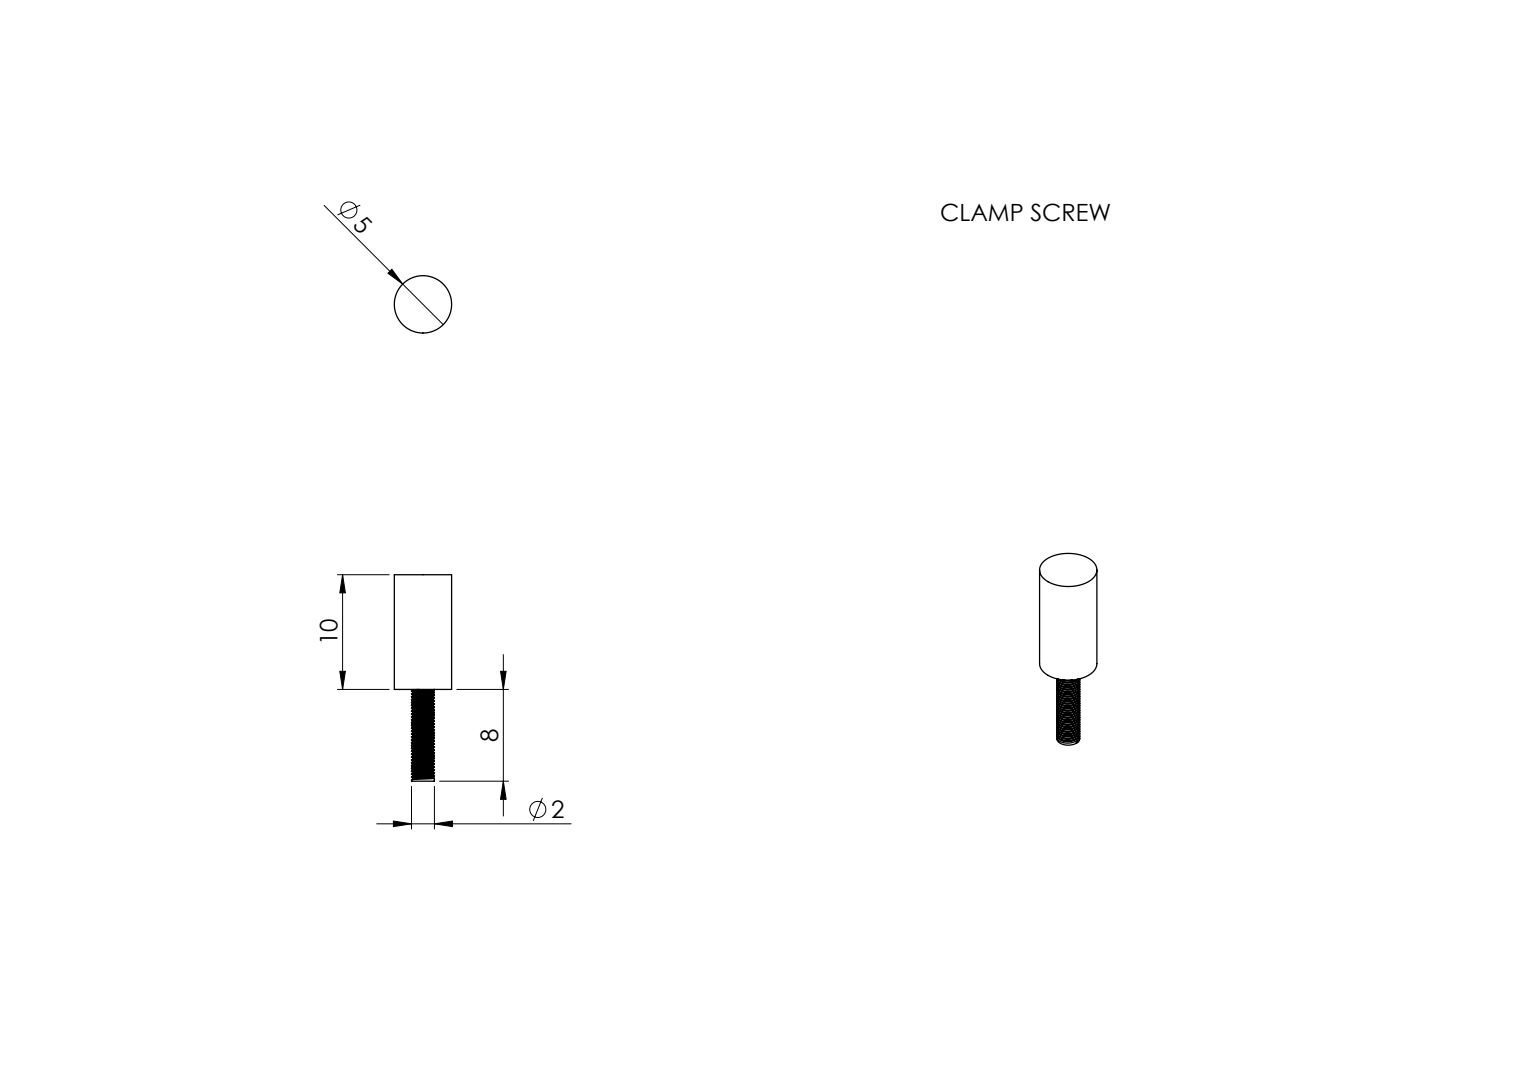
ISO-10303-21;
HEADER;
FILE_DESCRIPTION (('STEP AP214'),
    '1' );
FILE_NAME ('clamp screw.step',
    '2026-10-27T04:40:18',
    ( '' ),
    ( '' ),
    'SwSTEP 2.0',
    'SolidWorks 2026',
    '' );
FILE_SCHEMA (( 'AUTOMOTIVE_DESIGN' ));
ENDSEC;

DATA;
#2=CARTESIAN_POINT ( 'NONE',  ( -60.99999999999998579, 10.72916666666666607, 2.077350269189628840 ) ) ;
#3=CARTESIAN_POINT ( 'NONE',  ( -62.86468353124999453, 12.51562499965860198, 1.500000000000002220 ) ) ;
#4=CARTESIAN_POINT ( 'NONE',  ( -62.43234176562498305, 9.411458332991935904, 0.7511620957034662593 ) ) ;
#5=DIRECTION ( 'NONE',  ( 0.000000000000000000, 0.000000000000000000, -1.000000000000000000 ) ) ;
#7=CARTESIAN_POINT ( 'NONE',  ( -61.99999999999998579, 16.00000000000000000, 1.500000000000002220 ) ) ;
#8=CARTESIAN_POINT ( 'NONE',  ( -62.43234176562498305, 9.223958332991935904, 0.7511620957034662593 ) ) ;
#14=CARTESIAN_POINT ( 'NONE',  ( -62.86468353124998032, 15.68229166632526628, 1.000774730468978024 ) ) ;
#15=CARTESIAN_POINT ( 'NONE',  ( -61.99999999999998579, 11.14062499965860020, 0.5015494609379544944 ) ) ;
#16=CARTESIAN_POINT ( 'NONE',  ( -62.86468353124999453, 16.03645833299193768, 1.999225269531025750 ) ) ;
#17=CARTESIAN_POINT ( 'NONE',  ( -61.49999999999998579, 9.677083332650534331, 2.366025403784441927 ) ) ;
#18=ORIENTED_EDGE ( 'NONE', *, *, #1732, .F. ) ;
#19=CARTESIAN_POINT ( 'NONE',  ( -62.49999999999998579, 14.58333333333333393, 0.6339745962155627357 ) ) ;
#21=CARTESIAN_POINT ( 'NONE',  ( -61.56765823437498852, 8.598958332991934128, 2.248837904296538515 ) ) ;
#23=CARTESIAN_POINT ( 'NONE',  ( -61.49999999999998579, 13.67708333265053433, 2.366025403784441927 ) ) ;
#26=( BOUNDED_CURVE ( )  B_SPLINE_CURVE ( 2, ( #4662, #10727, #5554, #5432, #3111, #6399, #1393, #5495, #3837 ),
 .UNSPECIFIED., .F., .T. ) 
 B_SPLINE_CURVE_WITH_KNOTS ( ( 3, 2, 2, 2, 3 ),
 ( 0.3984375000000000000, 0.4010416666666666852, 0.4062500000000000000, 0.4114583333333333148, 0.4140625000000000000 ),
 .UNSPECIFIED. ) 
 CURVE ( )  GEOMETRIC_REPRESENTATION_ITEM ( )  RATIONAL_B_SPLINE_CURVE ( ( 0.9330127018922194093, 0.9330127018922194093, 1.000000000000000000, 0.8660254037844387076, 1.000000000000000000, 0.8660254037844387076, 1.000000000000000000, 0.9330127018922194093, 0.9330127018922194093 ) ) 
 REPRESENTATION_ITEM ( '' )  );
#27=CARTESIAN_POINT ( 'NONE',  ( -62.86468353124998032, 11.68229166632526983, 1.000774730468978024 ) ) ;
#31=CARTESIAN_POINT ( 'NONE',  ( -62.86468353124998742, 13.28645833299193413, 1.999225269531025972 ) ) ;
#32=CARTESIAN_POINT ( 'NONE',  ( -61.99999999999998579, 11.65624999931720218, 2.500000000000002665 ) ) ;
#35=VERTEX_POINT ( 'NONE', #9289 ) ;
#42=CARTESIAN_POINT ( 'NONE',  ( -61.99999999999998579, 8.703124999658601979, 0.5015494609379544944 ) ) ;
#43=CARTESIAN_POINT ( 'NONE',  ( -61.99999999999998579, 15.93749999999999645, 2.500000000000002665 ) ) ;
#44=AXIS2_PLACEMENT_3D ( 'NONE', #893, #1059, #6847 ) ;
#45=CARTESIAN_POINT ( 'NONE',  ( -61.13531646874998415, 12.66145833299193413, 1.000774730468978468 ) ) ;
#51=CARTESIAN_POINT ( 'NONE',  ( -62.99999999999998579, 11.57291666598387003, 0.9226497308103756012 ) ) ;
#52=CARTESIAN_POINT ( 'NONE',  ( -62.43234176562498305, 15.66145833299193590, 0.7511620957034662593 ) ) ;
#54=CARTESIAN_POINT ( 'NONE',  ( -61.49999999999998579, 12.51041666598386826, 0.6339745962155628467 ) ) ;
#55=CARTESIAN_POINT ( 'NONE',  ( -62.99999999999998579, 8.854166666666666075, 0.9226497308103756012 ) ) ;
#56=CARTESIAN_POINT ( 'NONE',  ( -61.13531646874997705, 12.41145833299193413, 1.000774730468978468 ) ) ;
#58=CARTESIAN_POINT ( 'NONE',  ( -61.13531646874998415, 9.057291666325266277, 1.999225269531026417 ) ) ;
#59=CARTESIAN_POINT ( 'NONE',  ( -61.49999999999998579, 9.208333333333333925, 2.366025403784441927 ) ) ;
#61=CARTESIAN_POINT ( 'NONE',  ( -61.13531646874998415, 9.661458332991932352, 1.000774730468978468 ) ) ;
#62=CARTESIAN_POINT ( 'NONE',  ( -62.99999999999998579, 14.07291666598387003, 0.9226497308103756012 ) ) ;
#64=VECTOR ( 'NONE', #9723, 1000.000000000000000 ) ;
#65=CARTESIAN_POINT ( 'NONE',  ( -61.99999999999998579, 12.81250000000000000, 0.5000000000000013323 ) ) ;
#66=CARTESIAN_POINT ( 'NONE',  ( -61.73205080756886076, 11.16741454900183328, 2.500000000000003109 ) ) ;
#67=CARTESIAN_POINT ( 'NONE',  ( -61.99999999999999289, 15.14062499965860198, 0.5015494609379544944 ) ) ;
#68=CARTESIAN_POINT ( 'NONE',  ( -62.43234176562499016, 10.74479166632526805, 2.248837904296538071 ) ) ;
#69=CARTESIAN_POINT ( 'NONE',  ( -61.99999999999999289, 15.82812499965860198, 2.498450539062049724 ) ) ;
#71=EDGE_LOOP ( 'NONE', ( #7087, #10551, #5486, #977 ) ) ;
#72=CARTESIAN_POINT ( 'NONE',  ( -62.49999999999998579, 15.08333333333333393, 0.6339745962155627357 ) ) ;
#73=CARTESIAN_POINT ( 'NONE',  ( -62.86468353124999453, 8.286458332991934128, 1.999225269531025750 ) ) ;
#74=CARTESIAN_POINT ( 'NONE',  ( -62.49999999999998579, 13.30208333265053433, 0.6339745962155627357 ) ) ;
#75=CARTESIAN_POINT ( 'NONE',  ( -62.99999999999998579, 13.12500000000000178, 1.500000000000001998 ) ) ;
#76=CARTESIAN_POINT ( 'NONE',  ( -61.99999999999998579, 9.812500000000000000, 0.5000000000000013323 ) ) ;
#77=CARTESIAN_POINT ( 'NONE',  ( -61.56765823437498852, 11.03645833299193590, 2.248837904296538515 ) ) ;
#78=( NAMED_UNIT ( * ) SI_UNIT ( $, .STERADIAN. ) SOLID_ANGLE_UNIT ( ) );
#79=CARTESIAN_POINT ( 'NONE',  ( -61.99999999999997868, 8.312499999999998224, 0.5000000000000013323 ) ) ;
#80=ORIENTED_EDGE ( 'NONE', *, *, #3705, .F. ) ;
#81=CARTESIAN_POINT ( 'NONE',  ( -61.99999999999998579, 12.15624999931720041, 2.500000000000002665 ) ) ;
#82=CARTESIAN_POINT ( 'NONE',  ( -61.13531646874998415, 13.16145833299193413, 1.000774730468978468 ) ) ;
#84=DIRECTION ( 'NONE',  ( -0.000000000000000000, -1.000000000000000000, -0.000000000000000000 ) ) ;
#85=CARTESIAN_POINT ( 'NONE',  ( -60.99999999999998579, 8.697916665983868256, 2.077350269189628840 ) ) ;
#87=( BOUNDED_CURVE ( )  B_SPLINE_CURVE ( 2, ( #8357, #10903, #5902, #8456, #10798, #841, #3187, #174, #6119 ),
 .UNSPECIFIED., .F., .T. ) 
 B_SPLINE_CURVE_WITH_KNOTS ( ( 3, 2, 2, 2, 3 ),
 ( 0.5703125000000000000, 0.5729166666666666297, 0.5781250000000000000, 0.5833333333333333703, 0.5859375000000000000 ),
 .UNSPECIFIED. ) 
 CURVE ( )  GEOMETRIC_REPRESENTATION_ITEM ( )  RATIONAL_B_SPLINE_CURVE ( ( 0.9330127018922194093, 0.9330127018922194093, 1.000000000000000000, 0.8660254037844387076, 1.000000000000000000, 0.8660254037844387076, 1.000000000000000000, 0.9330127018922194093, 0.9330127018922194093 ) ) 
 REPRESENTATION_ITEM ( '' )  );
#92=CARTESIAN_POINT ( 'NONE',  ( -62.43234176562498305, 11.91145833299193413, 0.7511620957034662593 ) ) ;
#94=CARTESIAN_POINT ( 'NONE',  ( -62.43234176562499016, 9.057291666325268054, 2.248837904296538071 ) ) ;
#95=LINE ( 'NONE', #7549, #8153 ) ;
#96=CARTESIAN_POINT ( 'NONE',  ( -61.56765823437498852, 12.59895833299193413, 2.248837904296538515 ) ) ;
#98=CARTESIAN_POINT ( 'NONE',  ( -61.99999999999998579, 8.281249999317202182, 0.5000000000000013323 ) ) ;
#100=CARTESIAN_POINT ( 'NONE',  ( -61.99999999999998579, 16.00000000000000000, 2.500000000000000444 ) ) ;
#101=ORIENTED_EDGE ( 'NONE', *, *, #9521, .F. ) ;
#102=CARTESIAN_POINT ( 'NONE',  ( -61.73205080756886076, 14.27008544963257108, 0.5000000000000014433 ) ) ;
#103=CARTESIAN_POINT ( 'NONE',  ( -61.13531646874998415, 15.30729166632526983, 1.999225269531026417 ) ) ;
#104=FACE_OUTER_BOUND ( 'NONE', #8107, .T. ) ;
#106=CARTESIAN_POINT ( 'NONE',  ( -62.49999999999998579, 12.30208333265053611, 0.6339745962155627357 ) ) ;
#108=CARTESIAN_POINT ( 'NONE',  ( -61.56765823437498852, 14.34895833299193413, 2.248837904296538515 ) ) ;
#109=CARTESIAN_POINT ( 'NONE',  ( -62.43234176562499016, 8.494791666325268054, 2.248837904296538071 ) ) ;
#110=CARTESIAN_POINT ( 'NONE',  ( -61.99999999999998579, 9.187500000000000000, 2.500000000000002665 ) ) ;
#112=CARTESIAN_POINT ( 'NONE',  ( -61.56765823437498142, 8.682291666325268054, 0.7511620957034663704 ) ) ;
#113=ADVANCED_FACE ( 'NONE', ( #788 ), #9184, .T. ) ;
#114=CARTESIAN_POINT ( 'NONE',  ( -62.49999999999998579, 14.05208333265053611, 0.6339745962155627357 ) ) ;
#119=CARTESIAN_POINT ( 'NONE',  ( -61.13531646874998415, 15.07812499965860020, 1.500000000000002220 ) ) ;
#120=CARTESIAN_POINT ( 'NONE',  ( -62.86468353124998032, 10.93229166632526805, 1.000774730468978246 ) ) ;
#121=CARTESIAN_POINT ( 'NONE',  ( -61.56765823437498852, 9.536458332991934128, 2.248837904296538515 ) ) ;
#122=ORIENTED_EDGE ( 'NONE', *, *, #10904, .T. ) ;
#123=CARTESIAN_POINT ( 'NONE',  ( -62.99999999999998579, 15.12500000000000000, 1.500000000000001998 ) ) ;
#124=CARTESIAN_POINT ( 'NONE',  ( -61.13531646874998415, 9.640624999658601979, 1.500000000000002220 ) ) ;
#127=CARTESIAN_POINT ( 'NONE',  ( -61.49999999999998579, 13.76041666598387003, 0.6339745962155628467 ) ) ;
#129=CARTESIAN_POINT ( 'NONE',  ( -61.99999999999998579, 14.90624999931720218, 2.500000000000002665 ) ) ;
#131=CARTESIAN_POINT ( 'NONE',  ( -62.86468353124999453, 11.97395833299193413, 1.999225269531025750 ) ) ;
#132=( NAMED_UNIT ( * ) PLANE_ANGLE_UNIT ( ) SI_UNIT ( $, .RADIAN. ) );
#133=LINE ( 'NONE', #9524, #10148 ) ;
#136=CARTESIAN_POINT ( 'NONE',  ( -61.13531646874998415, 12.91145833299193590, 1.000774730468978468 ) ) ;
#138=CARTESIAN_POINT ( 'NONE',  ( -60.99999999999998579, 10.22916666666666785, 2.077350269189628840 ) ) ;
#139=VECTOR ( 'NONE', #2970, 1000.000000000000000 ) ;
#140=CARTESIAN_POINT ( 'NONE',  ( -62.49999999999998579, 9.302083332650536107, 0.6339745962155627357 ) ) ;
#143=CARTESIAN_POINT ( 'NONE',  ( -61.73205080756886076, 14.05133545031537068, 0.5000000000000014433 ) ) ;
#145=CARTESIAN_POINT ( 'NONE',  ( -62.26794919243111082, 15.29241454900183328, 0.5000000000000013323 ) ) ;
#147=CARTESIAN_POINT ( 'NONE',  ( -61.13531646874998415, 11.05729166632526805, 1.999225269531026417 ) ) ;
#151=CARTESIAN_POINT ( 'NONE',  ( -61.13531646874998415, 8.411458332991934128, 1.000774730468978468 ) ) ;
#155=CARTESIAN_POINT ( 'NONE',  ( -61.56765823437498852, 14.09895833299193413, 2.248837904296538515 ) ) ;
#156=CARTESIAN_POINT ( 'NONE',  ( -62.49999999999998579, 9.302083332650536107, 0.6339745962155627357 ) ) ;
#157=ORIENTED_EDGE ( 'NONE', *, *, #473, .F. ) ;
#160=CARTESIAN_POINT ( 'NONE',  ( -62.49999999999998579, 10.83333333333333393, 0.6339745962155627357 ) ) ;
#161=CARTESIAN_POINT ( 'NONE',  ( -62.99999999999998579, 8.104166666666667851, 0.9226497308103756012 ) ) ;
#163=CARTESIAN_POINT ( 'NONE',  ( -61.99999999999997868, 8.781249999317202182, 0.5000000000000013323 ) ) ;
#164=DIRECTION ( 'NONE',  ( -0.000000000000000000, -1.000000000000000000, -0.000000000000000000 ) ) ;
#165=CARTESIAN_POINT ( 'NONE',  ( -61.73205080756888208, 10.69866454968463110, 2.500000000000006661 ) ) ;
#166=CARTESIAN_POINT ( 'NONE',  ( -61.13531646874997705, 13.41145833299193413, 1.000774730468978468 ) ) ;
#167=CARTESIAN_POINT ( 'NONE',  ( -61.56765823437498142, 8.869791666325268054, 0.7511620957034663704 ) ) ;
#168=LINE ( 'NONE', #6113, #341 ) ;
#170=CARTESIAN_POINT ( 'NONE',  ( -62.86468353124998742, 9.786458332991934128, 1.999225269531025972 ) ) ;
#172=ORIENTED_EDGE ( 'NONE', *, *, #7897, .T. ) ;
#174=CARTESIAN_POINT ( 'NONE',  ( -62.26794919243111082, 12.67633545031537068, 2.500000000000003109 ) ) ;
#175=EDGE_CURVE ( 'NONE', #2979, #4700, #8697, .T. ) ;
#177=CARTESIAN_POINT ( 'NONE',  ( -62.43234176562499016, 14.99479166632526805, 2.248837904296538071 ) ) ;
#178=CARTESIAN_POINT ( 'NONE',  ( -62.86468353124998742, 11.47395833299193590, 1.999225269531025972 ) ) ;
#180=ADVANCED_FACE ( 'NONE', ( #9080 ), #7568, .T. ) ;
#181=CARTESIAN_POINT ( 'NONE',  ( -61.13531646874998415, 8.578124999658601979, 1.500000000000002220 ) ) ;
#182=CARTESIAN_POINT ( 'NONE',  ( -61.99999999999998579, 11.40624999931720218, 2.500000000000002665 ) ) ;
#183=ORIENTED_EDGE ( 'NONE', *, *, #3221, .T. ) ;
#184=CARTESIAN_POINT ( 'NONE',  ( -62.99999999999998579, 14.60416666666666785, 0.9226497308103756012 ) ) ;
#185=CARTESIAN_POINT ( 'NONE',  ( -61.56765823437498852, 10.09895833299193413, 2.248837904296538515 ) ) ;
#186=CARTESIAN_POINT ( 'NONE',  ( -62.99999999999998579, 13.59374999931720218, 1.500000000000001998 ) ) ;
#188=ORIENTED_EDGE ( 'NONE', *, *, #5061, .T. ) ;
#189=CYLINDRICAL_SURFACE ( 'NONE', #9638, 0.9999999999999981126 ) ;
#190=CARTESIAN_POINT ( 'NONE',  ( -62.86468353124998032, 10.93229166632526805, 1.000774730468978024 ) ) ;
#191=CARTESIAN_POINT ( 'NONE',  ( -60.99999999999998579, 13.00000000000000178, 1.500000000000002220 ) ) ;
#193=CARTESIAN_POINT ( 'NONE',  ( -62.49999999999998579, 10.58333333333333393, 0.6339745962155627357 ) ) ;
#194=CARTESIAN_POINT ( 'NONE',  ( -61.73205080756886076, 15.91741454900183150, 2.500000000000003109 ) ) ;
#195=CARTESIAN_POINT ( 'NONE',  ( -62.86468353124999453, 14.26562499965860020, 1.500000000000002220 ) ) ;
#196=CARTESIAN_POINT ( 'NONE',  ( -62.49999999999998579, 13.91666666666666785, 2.366025403784441483 ) ) ;
#198=CARTESIAN_POINT ( 'NONE',  ( -62.99999999999998579, 8.614583332650536107, 2.077350269189627952 ) ) ;
#202=CARTESIAN_POINT ( 'NONE',  ( -61.73205080756886076, 10.02008544963257464, 0.5000000000000014433 ) ) ;
#203=CARTESIAN_POINT ( 'NONE',  ( -61.56765823437498142, 11.36979166632526805, 0.7511620957034663704 ) ) ;
#207=CARTESIAN_POINT ( 'NONE',  ( -61.13531646874998415, 10.91145833299193590, 1.000774730468978468 ) ) ;
#209=CARTESIAN_POINT ( 'NONE',  ( -61.13531646874998415, 14.16145833299193413, 1.000774730468978468 ) ) ;
#210=CARTESIAN_POINT ( 'NONE',  ( -62.26794919243111082, 9.292414549001833279, 0.5000000000000013323 ) ) ;
#217=CARTESIAN_POINT ( 'NONE',  ( -61.99999999999998579, 15.03124999931720218, 0.5000000000000013323 ) ) ;
#218=CARTESIAN_POINT ( 'NONE',  ( -61.99999999999998579, 8.437500000000000000, 2.654700538379254571 ) ) ;
#219=CARTESIAN_POINT ( 'NONE',  ( -61.99999999999998579, 13.68749999999999822, 2.500000000000002665 ) ) ;
#221=DIRECTION ( 'NONE',  ( -0.000000000000000000, -1.000000000000000000, -0.000000000000000000 ) ) ;
#223=CARTESIAN_POINT ( 'NONE',  ( -62.86468353124998032, 14.49479166632526983, 1.000774730468978024 ) ) ;
#225=CARTESIAN_POINT ( 'NONE',  ( -61.99999999999998579, 8.515624999658601979, 2.498450539062049724 ) ) ;
#226=CARTESIAN_POINT ( 'NONE',  ( -62.99999999999998579, 11.32291666598387181, 0.9226497308103756012 ) ) ;
#228=CARTESIAN_POINT ( 'NONE',  ( -61.13531646874998415, 10.11979166632526805, 1.999225269531026417 ) ) ;
#229=CARTESIAN_POINT ( 'NONE',  ( -61.99999999999998579, 14.03124999931720218, 0.5000000000000013323 ) ) ;
#232=CARTESIAN_POINT ( 'NONE',  ( -61.99999999999998579, 13.03124999931720218, 0.5000000000000013323 ) ) ;
#235=CARTESIAN_POINT ( 'NONE',  ( -61.13531646874997705, 15.59895833299193590, 1.000774730468978468 ) ) ;
#236=CARTESIAN_POINT ( 'NONE',  ( -61.56765823437498852, 13.03645833299193413, 2.248837904296538515 ) ) ;
#237=CARTESIAN_POINT ( 'NONE',  ( -61.99999999999999289, 8.265624999658601979, 2.498450539062049724 ) ) ;
#239=CARTESIAN_POINT ( 'NONE',  ( -62.26794919243111082, 14.07366454968463110, 0.5000000000000013323 ) ) ;
#240=CARTESIAN_POINT ( 'NONE',  ( -62.43234176562499016, 9.557291666325268054, 2.248837904296538071 ) ) ;
#241=CARTESIAN_POINT ( 'NONE',  ( -61.56765823437498852, 14.78645833299193413, 2.248837904296538515 ) ) ;
#243=CARTESIAN_POINT ( 'NONE',  ( -61.99999999999998579, 14.28124999931720396, 0.3452994616207497591 ) ) ;
#245=ORIENTED_EDGE ( 'NONE', *, *, #9568, .F. ) ;
#246=CARTESIAN_POINT ( 'NONE',  ( -61.73205080756886076, 9.801335450315370679, 0.5000000000000014433 ) ) ;
#248=CARTESIAN_POINT ( 'NONE',  ( -61.13531646874998415, 12.07812499965860198, 1.500000000000002220 ) ) ;
#249=CYLINDRICAL_SURFACE ( 'NONE', #10424, 0.9999999999999981126 ) ;
#252=CARTESIAN_POINT ( 'NONE',  ( -61.49999999999998579, 11.04166666666666607, 0.6339745962155628467 ) ) ;
#253=CARTESIAN_POINT ( 'NONE',  ( -61.99999999999998579, 8.531249999317203958, 0.5000000000000013323 ) ) ;
#254=CARTESIAN_POINT ( 'NONE',  ( -61.99999999999998579, 14.57812499965860198, 2.498450539062049724 ) ) ;
#255=( BOUNDED_CURVE ( )  B_SPLINE_CURVE ( 2, ( #5430, #6282, #8897, #2058, #9721, #9666, #6225, #10606, #9607 ),
 .UNSPECIFIED., .F., .T. ) 
 B_SPLINE_CURVE_WITH_KNOTS ( ( 3, 2, 2, 2, 3 ),
 ( 0.08593750000000000000, 0.08854166666666667129, 0.09375000000000000000, 0.09895833333333332871, 0.1015625000000000833 ),
 .UNSPECIFIED. ) 
 CURVE ( )  GEOMETRIC_REPRESENTATION_ITEM ( )  RATIONAL_B_SPLINE_CURVE ( ( 0.9330127018922194093, 0.9330127018922194093, 1.000000000000000000, 0.8660254037844387076, 1.000000000000000000, 0.8660254037844387076, 1.000000000000000000, 0.9330127018922171889, 0.9330127018922194093 ) ) 
 REPRESENTATION_ITEM ( '' )  );
#257=CARTESIAN_POINT ( 'NONE',  ( -61.99999999999998579, 13.93749999999999822, 2.500000000000002665 ) ) ;
#258=CARTESIAN_POINT ( 'NONE',  ( -62.99999999999998579, 9.364583332650536107, 2.077350269189627952 ) ) ;
#260=CARTESIAN_POINT ( 'NONE',  ( -61.49999999999998579, 13.54166666666666785, 0.6339745962155628467 ) ) ;
#261=CARTESIAN_POINT ( 'NONE',  ( -62.49999999999998579, 15.38541666598387003, 2.366025403784441483 ) ) ;
#262=CARTESIAN_POINT ( 'NONE',  ( -62.43234176562499016, 10.74479166632526805, 2.248837904296538071 ) ) ;
#263=ADVANCED_FACE ( 'NONE', ( #7011 ), #2615, .T. ) ;
#264=ORIENTED_EDGE ( 'NONE', *, *, #1352, .F. ) ;
#265=CARTESIAN_POINT ( 'NONE',  ( -62.43234176562499016, 10.05729166632526805, 2.248837904296538071 ) ) ;
#267=CARTESIAN_POINT ( 'NONE',  ( -61.13531646874998415, 13.86979166632526805, 1.999225269531026417 ) ) ;
#269=ORIENTED_EDGE ( 'NONE', *, *, #9235, .F. ) ;
#273=CARTESIAN_POINT ( 'NONE',  ( -62.49999999999998579, 8.416666666666666075, 2.366025403784441483 ) ) ;
#277=CARTESIAN_POINT ( 'NONE',  ( -61.56765823437498142, 13.93229166632526805, 0.7511620957034663704 ) ) ;
#278=CARTESIAN_POINT ( 'NONE',  ( -62.86468353124998742, 9.723958332991934128, 1.999225269531025972 ) ) ;
#280=CARTESIAN_POINT ( 'NONE',  ( -61.13531646874998415, 9.911458332991935904, 1.000774730468978468 ) ) ;
#281=CARTESIAN_POINT ( 'NONE',  ( -62.49999999999998579, 12.08333333333333393, 0.6339745962155627357 ) ) ;
#283=EDGE_CURVE ( 'NONE', #10857, #3037, #6901, .T. ) ;
#284=VECTOR ( 'NONE', #526, 1000.000000000000000 ) ;
#286=CARTESIAN_POINT ( 'NONE',  ( -60.99999999999998579, 12.98958333265053611, 0.9226497308103762673 ) ) ;
#287=ADVANCED_FACE ( 'NONE', ( #6844 ), #3445, .T. ) ;
#288=CARTESIAN_POINT ( 'NONE',  ( -62.26794919243111082, 10.04241454900183328, 0.5000000000000013323 ) ) ;
#289=CARTESIAN_POINT ( 'NONE',  ( -61.99999999999998579, 12.14062499965860198, 0.5015494609379544944 ) ) ;
#290=CARTESIAN_POINT ( 'NONE',  ( -61.99999999999999289, 8.890624999658601979, 0.5015494609379544944 ) ) ;
#293=CARTESIAN_POINT ( 'NONE',  ( -60.99999999999998579, 15.97916666666666607, 2.077350269189628840 ) ) ;
#294=CARTESIAN_POINT ( 'NONE',  ( -61.13531646874997705, 10.41145833299193413, 1.000774730468978468 ) ) ;
#296=CARTESIAN_POINT ( 'NONE',  ( -61.56765823437498142, 15.61979166632526628, 0.7511620957034663704 ) ) ;
#297=ADVANCED_FACE ( 'NONE', ( #7844 ), #6003, .T. ) ;
#298=CARTESIAN_POINT ( 'NONE',  ( -60.99999999999998579, 14.48958333265053788, 0.9226497308103762673 ) ) ;
#301=CYLINDRICAL_SURFACE ( 'NONE', #3236, 0.9999999999999981126 ) ;
#303=CARTESIAN_POINT ( 'NONE',  ( -61.56765823437498852, 12.78645833299193413, 2.248837904296538515 ) ) ;
#304=CARTESIAN_POINT ( 'NONE',  ( -61.56765823437498142, 8.619791666325268054, 0.7511620957034663704 ) ) ;
#305=CARTESIAN_POINT ( 'NONE',  ( -61.49999999999998579, 15.54166666666666607, 0.6339745962155628467 ) ) ;
#307=CARTESIAN_POINT ( 'NONE',  ( -61.99999999999998579, 12.18750000000000000, 2.654700538379254571 ) ) ;
#308=LINE ( 'NONE', #2873, #10328 ) ;
#309=CARTESIAN_POINT ( 'NONE',  ( -62.86468353124998032, 13.99479166632526983, 1.000774730468978246 ) ) ;
#311=CARTESIAN_POINT ( 'NONE',  ( -61.49999999999998579, 10.26041666598387003, 0.6339745962155628467 ) ) ;
#312=VERTEX_POINT ( 'NONE', #9336 ) ;
#314=CARTESIAN_POINT ( 'NONE',  ( -60.99999999999998579, 9.989583332650536107, 0.9226497308103762673 ) ) ;
#315=CARTESIAN_POINT ( 'NONE',  ( -61.99999999999998579, 12.89062499965860376, 0.5015494609379544944 ) ) ;
#316=ADVANCED_FACE ( 'NONE', ( #9447 ), #3389, .T. ) ;
#317=CARTESIAN_POINT ( 'NONE',  ( -61.49999999999998579, 15.95833333333333215, 2.366025403784441927 ) ) ;
#318=( BOUNDED_CURVE ( )  B_SPLINE_CURVE ( 2, ( #338, #1054, #8015, #9617, #7841, #6343, #2731, #6291, #1116 ),
 .UNSPECIFIED., .F., .T. ) 
 B_SPLINE_CURVE_WITH_KNOTS ( ( 3, 2, 2, 2, 3 ),
 ( 0.1953124999999999722, 0.1979166666666666574, 0.2031250000000000000, 0.2083333333333333426, 0.2109375000000000000 ),
 .UNSPECIFIED. ) 
 CURVE ( )  GEOMETRIC_REPRESENTATION_ITEM ( )  RATIONAL_B_SPLINE_CURVE ( ( 0.9330127018922194093, 0.9330127018922186322, 1.000000000000000000, 0.8660254037844387076, 1.000000000000000000, 0.8660254037844387076, 1.000000000000000000, 0.9330127018922194093, 0.9330127018922194093 ) ) 
 REPRESENTATION_ITEM ( '' )  );
#319=EDGE_LOOP ( 'NONE', ( #4285, #2336, #2477, #10429 ) ) ;
#320=EDGE_CURVE ( 'NONE', #4602, #5526, #6439, .T. ) ;
#321=CARTESIAN_POINT ( 'NONE',  ( -61.99999999999998579, 10.20312499965860198, 0.5015494609379544944 ) ) ;
#323=CARTESIAN_POINT ( 'NONE',  ( -61.56765823437498852, 14.34895833299193413, 2.248837904296538515 ) ) ;
#329=ORIENTED_EDGE ( 'NONE', *, *, #3272, .T. ) ;
#331=CARTESIAN_POINT ( 'NONE',  ( -60.99999999999998579, 8.000000000000000000, 1.500000000000002220 ) ) ;
#335=CARTESIAN_POINT ( 'NONE',  ( -62.86468353124999453, 14.26562499965860020, 1.500000000000002220 ) ) ;
#336=CARTESIAN_POINT ( 'NONE',  ( -61.13531646874998415, 10.32812499965860198, 1.500000000000002220 ) ) ;
#337=CARTESIAN_POINT ( 'NONE',  ( -61.99999999999998579, 13.28124999931720041, 0.5000000000000013323 ) ) ;
#338=CARTESIAN_POINT ( 'NONE',  ( -61.99999999999998579, 9.562500000000000000, 0.5000000000000013323 ) ) ;
#340=CARTESIAN_POINT ( 'NONE',  ( -62.86468353124998742, 10.78645833299193413, 1.999225269531025972 ) ) ;
#341=VECTOR ( 'NONE', #8505, 1000.000000000000000 ) ;
#347=ORIENTED_EDGE ( 'NONE', *, *, #4046, .F. ) ;
#348=CARTESIAN_POINT ( 'NONE',  ( -61.13531646874998415, 8.140624999658601979, 1.500000000000002220 ) ) ;
#349=CARTESIAN_POINT ( 'NONE',  ( -61.13531646874998415, 12.55729166632526805, 1.999225269531026417 ) ) ;
#350=CARTESIAN_POINT ( 'NONE',  ( -61.56765823437498852, 8.786458332991934128, 2.248837904296538515 ) ) ;
#354=DIRECTION ( 'NONE',  ( -0.000000000000000000, -1.000000000000000000, -0.000000000000000000 ) ) ;
#355=CARTESIAN_POINT ( 'NONE',  ( -61.99999999999999289, 10.32812499965860198, 2.498450539062049724 ) ) ;
#357=CARTESIAN_POINT ( 'NONE',  ( -62.43234176562499016, 14.74479166632526805, 2.248837904296538071 ) ) ;
#358=VECTOR ( 'NONE', #7829, 1000.000000000000000 ) ;
#359=CARTESIAN_POINT ( 'NONE',  ( -60.99999999999998579, 13.94791666598387003, 2.077350269189628840 ) ) ;
#360=CYLINDRICAL_SURFACE ( 'NONE', #3974, 0.9999999999999981126 ) ;
#363=CARTESIAN_POINT ( 'NONE',  ( -61.99999999999998579, 16.00000000000000000, 1.500000000000002220 ) ) ;
#366=CARTESIAN_POINT ( 'NONE',  ( -61.13531646874998415, 12.57812499965860198, 1.500000000000002220 ) ) ;
#368=CARTESIAN_POINT ( 'NONE',  ( -62.43234176562499016, 8.994791666325268054, 2.248837904296538071 ) ) ;
#369=CARTESIAN_POINT ( 'NONE',  ( -62.99999999999998579, 10.59374999931720396, 1.500000000000001998 ) ) ;
#370=EDGE_LOOP ( 'NONE', ( #10927, #3084, #707, #1709 ) ) ;
#371=CARTESIAN_POINT ( 'NONE',  ( -62.99999999999998579, 12.87500000000000178, 1.500000000000001998 ) ) ;
#373=CARTESIAN_POINT ( 'NONE',  ( -61.13531646874998415, 14.64062499965860020, 1.500000000000002220 ) ) ;
#374=CARTESIAN_POINT ( 'NONE',  ( -62.26794919243111082, 13.92633545031537068, 2.500000000000003109 ) ) ;
#375=CARTESIAN_POINT ( 'NONE',  ( -61.49999999999998579, 11.26041666598387003, 0.6339745962155628467 ) ) ;
#376=ORIENTED_EDGE ( 'NONE', *, *, #2316, .F. ) ;
#379=CARTESIAN_POINT ( 'NONE',  ( -61.13531646874998415, 12.30729166632526628, 1.999225269531026417 ) ) ;
#381=VERTEX_POINT ( 'NONE', #7734 ) ;
#382=CARTESIAN_POINT ( 'NONE',  ( -61.13531646874998415, 10.14062499965860198, 1.500000000000002220 ) ) ;
#383=CYLINDRICAL_SURFACE ( 'NONE', #5279, 0.9999999999999981126 ) ;
#384=CARTESIAN_POINT ( 'NONE',  ( -62.86468353124999453, 14.76562499965860020, 1.500000000000002220 ) ) ;
#385=DIRECTION ( 'NONE',  ( -0.000000000000000000, -1.000000000000000000, -0.000000000000000000 ) ) ;
#388=EDGE_CURVE ( 'NONE', #8021, #5388, #10231, .T. ) ;
#389=( BOUNDED_CURVE ( )  B_SPLINE_CURVE ( 2, ( #8655, #9486, #5983, #9430, #1883, #5039, #9376, #1038, #1666 ),
 .UNSPECIFIED., .F., .F. ) 
 B_SPLINE_CURVE_WITH_KNOTS ( ( 3, 2, 2, 2, 3 ),
 ( 0.6484375000000000000, 0.6510416666666666297, 0.6562500000000000000, 0.6614583333333333703, 0.6640625000000000000 ),
 .UNSPECIFIED. ) 
 CURVE ( )  GEOMETRIC_REPRESENTATION_ITEM ( )  RATIONAL_B_SPLINE_CURVE ( ( 0.9330127018922194093, 0.9330127018922194093, 1.000000000000000000, 0.8660254037844387076, 1.000000000000000000, 0.8660254037844387076, 1.000000000000000000, 0.9330127018922194093, 0.9330127018922194093 ) ) 
 REPRESENTATION_ITEM ( '' )  );
#390=AXIS2_PLACEMENT_3D ( 'NONE', #8453, #10271, #7624 ) ;
#393=CARTESIAN_POINT ( 'NONE',  ( -60.99999999999998579, 8.479166666666666075, 2.077350269189628840 ) ) ;
#394=CARTESIAN_POINT ( 'NONE',  ( -62.26794919243111082, 9.645085449632574637, 2.500000000000006217 ) ) ;
#395=CARTESIAN_POINT ( 'NONE',  ( -61.99999999999998579, 14.28124999931720218, 0.5000000000000013323 ) ) ;
#397=CARTESIAN_POINT ( 'NONE',  ( -62.86468353124999453, 14.78645833299193058, 1.999225269531025750 ) ) ;
#398=CARTESIAN_POINT ( 'NONE',  ( -62.43234176562498305, 10.16145833299193413, 0.7511620957034662593 ) ) ;
#400=CARTESIAN_POINT ( 'NONE',  ( -62.99999999999998579, 11.36458333265053611, 2.077350269189627952 ) ) ;
#403=CARTESIAN_POINT ( 'NONE',  ( -61.13531646874998415, 11.14062499965860020, 1.500000000000002220 ) ) ;
#411=CARTESIAN_POINT ( 'NONE',  ( -61.73205080756886787, 10.16741454900183150, 2.500000000000004885 ) ) ;
#413=CARTESIAN_POINT ( 'NONE',  ( -61.13531646874998415, 12.84895833299193413, 1.000774730468978468 ) ) ;
#414=VECTOR ( 'NONE', #2699, 1000.000000000000000 ) ;
#415=CARTESIAN_POINT ( 'NONE',  ( -61.56765823437498142, 10.61979166632526805, 0.7511620957034663704 ) ) ;
#416=CARTESIAN_POINT ( 'NONE',  ( -61.99999999999998579, 16.00000000000000000, 0.5000000000000041078 ) ) ;
#418=CARTESIAN_POINT ( 'NONE',  ( -60.99999999999998579, 8.468749999317202182, 1.500000000000002220 ) ) ;
#419=CARTESIAN_POINT ( 'NONE',  ( -61.13531646874998415, 11.14062499965860020, 1.500000000000002220 ) ) ;
#421=CARTESIAN_POINT ( 'NONE',  ( -61.99999999999998579, 14.76562499965859843, 2.498450539062049724 ) ) ;
#422=CARTESIAN_POINT ( 'NONE',  ( -60.99999999999998579, 15.19791666598387181, 2.077350269189628840 ) ) ;
#424=VERTEX_POINT ( 'NONE', #4552 ) ;
#428=CARTESIAN_POINT ( 'NONE',  ( -61.56765823437498852, 13.28645833299193413, 2.248837904296538515 ) ) ;
#429=DIRECTION ( 'NONE',  ( -0.000000000000000000, -1.000000000000000000, -0.000000000000000000 ) ) ;
#432=CARTESIAN_POINT ( 'NONE',  ( -60.99999999999998579, 12.50000000000000000, 1.500000000000002220 ) ) ;
#434=CARTESIAN_POINT ( 'NONE',  ( -60.99999999999998579, 15.94791666598386826, 2.077350269189628840 ) ) ;
#436=CARTESIAN_POINT ( 'NONE',  ( -62.99999999999998579, 14.36458333265053611, 2.077350269189627952 ) ) ;
#437=CARTESIAN_POINT ( 'NONE',  ( -62.99999999999998579, 10.86458333265053611, 2.077350269189627952 ) ) ;
#439=CARTESIAN_POINT ( 'NONE',  ( -61.99999999999998579, 8.000000000000000000, 1.500000000000002220 ) ) ;
#440=CARTESIAN_POINT ( 'NONE',  ( -62.86468353124999453, 12.95312499965860198, 1.500000000000002220 ) ) ;
#442=ORIENTED_EDGE ( 'NONE', *, *, #9663, .T. ) ;
#443=CARTESIAN_POINT ( 'NONE',  ( -61.56765823437498142, 10.68229166632526805, 0.7511620957034663704 ) ) ;
#444=CARTESIAN_POINT ( 'NONE',  ( -62.26794919243111082, 12.54241454900183150, 0.5000000000000013323 ) ) ;
#446=CARTESIAN_POINT ( 'NONE',  ( -62.43234176562498305, 15.47395833299193590, 0.7511620957034662593 ) ) ;
#447=CARTESIAN_POINT ( 'NONE',  ( -61.73205080756885366, 9.020085449632572860, 0.5000000000000028866 ) ) ;
#452=CARTESIAN_POINT ( 'NONE',  ( -62.49999999999998579, 9.416666666666666075, 2.366025403784441483 ) ) ;
#455=CARTESIAN_POINT ( 'NONE',  ( -61.99999999999998579, 8.937500000000001776, 2.500000000000002665 ) ) ;
#456=CARTESIAN_POINT ( 'NONE',  ( -61.56765823437498142, 9.869791666325268054, 0.7511620957034663704 ) ) ;
#458=CARTESIAN_POINT ( 'NONE',  ( -62.49999999999998579, 8.302083332650536107, 0.6339745962155627357 ) ) ;
#459=CARTESIAN_POINT ( 'NONE',  ( -62.86468353124998032, 10.49479166632526983, 1.000774730468978246 ) ) ;
#463=CARTESIAN_POINT ( 'NONE',  ( -62.26794919243111082, 9.073664549684631098, 0.5000000000000013323 ) ) ;
#466=EDGE_CURVE ( 'NONE', #3158, #5222, #8079, .T. ) ;
#467=CARTESIAN_POINT ( 'NONE',  ( -61.13531646874998415, 12.05729166632526628, 1.999225269531026417 ) ) ;
#468=CARTESIAN_POINT ( 'NONE',  ( -62.86468353124999453, 10.20312499965860198, 1.500000000000002220 ) ) ;
#470=VERTEX_POINT ( 'NONE', #8792 ) ;
#471=CARTESIAN_POINT ( 'NONE',  ( -62.49999999999998579, 10.88541666598386826, 2.366025403784441483 ) ) ;
#472=CARTESIAN_POINT ( 'NONE',  ( -62.86468353124999453, 11.28645833299193590, 1.999225269531025750 ) ) ;
#473=EDGE_CURVE ( 'NONE', #4413, #2594, #6911, .T. ) ;
#475=CARTESIAN_POINT ( 'NONE',  ( -62.43234176562499016, 15.99479166632526628, 2.248837904296538071 ) ) ;
#476=CARTESIAN_POINT ( 'NONE',  ( -60.99999999999998579, 14.21874999931720218, 1.500000000000002220 ) ) ;
#479=EDGE_CURVE ( 'NONE', #827, #9464, #8846, .T. ) ;
#481=CARTESIAN_POINT ( 'NONE',  ( -62.43234176562498305, 13.41145833299193413, 0.7511620957034662593 ) ) ;
#482=FACE_OUTER_BOUND ( 'NONE', #8139, .T. ) ;
#483=DIRECTION ( 'NONE',  ( 0.000000000000000000, 0.000000000000000000, 1.000000000000000000 ) ) ;
#485=CARTESIAN_POINT ( 'NONE',  ( -62.99999999999998579, 12.85416666666666607, 0.9226497308103756012 ) ) ;
#486=CARTESIAN_POINT ( 'NONE',  ( -62.99999999999998579, 13.36458333265053433, 2.077350269189627952 ) ) ;
#488=CARTESIAN_POINT ( 'NONE',  ( -62.49999999999998579, 10.88541666598386826, 2.366025403784441483 ) ) ;
#491=CARTESIAN_POINT ( 'NONE',  ( -62.49999999999998579, 14.83333333333333393, 0.6339745962155627357 ) ) ;
#492=( BOUNDED_CURVE ( )  B_SPLINE_CURVE ( 2, ( #3999, #2659, #9428, #769, #3480, #1604, #9318, #6668, #43 ),
 .UNSPECIFIED., .F., .F. ) 
 B_SPLINE_CURVE_WITH_KNOTS ( ( 3, 2, 2, 2, 3 ),
 ( 0.9765625000000000000, 0.9791666666666666297, 0.9843750000000000000, 0.9895833333333333703, 0.9921875000000000000 ),
 .UNSPECIFIED. ) 
 CURVE ( )  GEOMETRIC_REPRESENTATION_ITEM ( )  RATIONAL_B_SPLINE_CURVE ( ( 0.9330127018922194093, 0.9330127018922194093, 1.000000000000000000, 0.8660254037844387076, 1.000000000000000000, 0.8660254037844387076, 1.000000000000000000, 0.9330127018922194093, 0.9330127018922194093 ) ) 
 REPRESENTATION_ITEM ( '' )  );
#493=CARTESIAN_POINT ( 'NONE',  ( -61.56765823437498852, 12.03645833299193413, 2.248837904296538515 ) ) ;
#496=CARTESIAN_POINT ( 'NONE',  ( -62.86468353124999453, 11.76562499965860198, 1.500000000000002220 ) ) ;
#497=EDGE_CURVE ( 'NONE', #2222, #3158, #7324, .T. ) ;
#500=CARTESIAN_POINT ( 'NONE',  ( -62.86468353124999453, 16.01562499965860198, 1.500000000000002220 ) ) ;
#504=DIRECTION ( 'NONE',  ( 0.000000000000000000, 0.000000000000000000, -1.000000000000000000 ) ) ;
#507=CARTESIAN_POINT ( 'NONE',  ( -60.99999999999998579, 8.697916665983868256, 2.077350269189628840 ) ) ;
#509=CARTESIAN_POINT ( 'NONE',  ( -60.99999999999998579, 10.27083333333333393, 0.9226497308103762673 ) ) ;
#513=CARTESIAN_POINT ( 'NONE',  ( -62.49999999999998579, 8.385416665983870033, 2.366025403784441483 ) ) ;
#515=CARTESIAN_POINT ( 'NONE',  ( -61.56765823437498142, 12.43229166632526805, 0.7511620957034663704 ) ) ;
#516=CARTESIAN_POINT ( 'NONE',  ( -62.49999999999998579, 13.58333333333333215, 0.6339745962155627357 ) ) ;
#519=CARTESIAN_POINT ( 'NONE',  ( -61.99999999999998579, 9.187500000000000000, 2.500000000000002665 ) ) ;
#521=ORIENTED_EDGE ( 'NONE', *, *, #9600, .F. ) ;
#522=CARTESIAN_POINT ( 'NONE',  ( -61.99999999999998579, 16.00000000000000000, 1.500000000000002220 ) ) ;
#523=CARTESIAN_POINT ( 'NONE',  ( -62.86468353124998742, 13.72395833299193413, 1.999225269531025972 ) ) ;
#525=CARTESIAN_POINT ( 'NONE',  ( -61.13531646874997705, 10.84895833299193413, 1.000774730468978468 ) ) ;
#526=DIRECTION ( 'NONE',  ( 0.000000000000000000, -1.000000000000000000, 0.000000000000000000 ) ) ;
#529=CARTESIAN_POINT ( 'NONE',  ( -62.43234176562498305, 10.97395833299193590, 0.7511620957034662593 ) ) ;
#532=CARTESIAN_POINT ( 'NONE',  ( -61.99999999999998579, 15.40624999931720218, 2.654700538379254571 ) ) ;
#533=CARTESIAN_POINT ( 'NONE',  ( -62.26794919243111082, 16.04241454900182973, 0.5000000000000013323 ) ) ;
#535=EDGE_CURVE ( 'NONE', #10303, #6298, #1585, .T. ) ;
#538=ADVANCED_FACE ( 'NONE', ( #8017 ), #3731, .F. ) ;
#540=CARTESIAN_POINT ( 'NONE',  ( -61.13531646874998415, 13.07812499965860198, 1.500000000000002220 ) ) ;
#541=CARTESIAN_POINT ( 'NONE',  ( -61.13531646874998415, 9.578124999658600203, 1.500000000000002220 ) ) ;
#543=CARTESIAN_POINT ( 'NONE',  ( -61.99999999999998579, 11.81249999999999822, 0.5000000000000013323 ) ) ;
#545=CARTESIAN_POINT ( 'NONE',  ( -62.49999999999998579, 13.08333333333333215, 0.6339745962155627357 ) ) ;
#546=CARTESIAN_POINT ( 'NONE',  ( -61.99999999999998579, 8.937500000000001776, 2.500000000000002665 ) ) ;
#548=CARTESIAN_POINT ( 'NONE',  ( -62.99999999999998579, 11.11458333265053611, 2.077350269189627952 ) ) ;
#550=CARTESIAN_POINT ( 'NONE',  ( -62.49999999999998579, 14.91666666666666607, 2.366025403784441483 ) ) ;
#552=CARTESIAN_POINT ( 'NONE',  ( -61.99999999999998579, 12.26562499965860198, 2.498450539062049724 ) ) ;
#556=CARTESIAN_POINT ( 'NONE',  ( -61.99999999999998579, 11.82812499965860198, 2.498450539062049724 ) ) ;
#557=CARTESIAN_POINT ( 'NONE',  ( -62.99999999999998579, 12.61458333265053611, 2.077350269189627952 ) ) ;
#559=ORIENTED_EDGE ( 'NONE', *, *, #4763, .T. ) ;
#561=CARTESIAN_POINT ( 'NONE',  ( -62.99999999999998579, 11.10416666666666607, 0.9226497308103756012 ) ) ;
#562=VERTEX_POINT ( 'NONE', #8127 ) ;
#563=CARTESIAN_POINT ( 'NONE',  ( -62.99999999999998579, 9.822916665983871809, 0.9226497308103756012 ) ) ;
#564=CARTESIAN_POINT ( 'NONE',  ( -62.99999999999998579, 9.125000000000000000, 1.500000000000001998 ) ) ;
#565=CARTESIAN_POINT ( 'NONE',  ( -61.99999999999998579, 26.00000000000000355, -1.000000000000000000 ) ) ;
#568=DIRECTION ( 'NONE',  ( -0.000000000000000000, -1.000000000000000000, -0.000000000000000000 ) ) ;
#569=CARTESIAN_POINT ( 'NONE',  ( -62.43234176562498305, 11.72395833299193590, 0.7511620957034662593 ) ) ;
#575=CARTESIAN_POINT ( 'NONE',  ( -60.99999999999998579, 14.21874999931720218, 1.500000000000002220 ) ) ;
#576=CARTESIAN_POINT ( 'NONE',  ( -61.99999999999998579, 13.64062499965860198, 0.5015494609379544944 ) ) ;
#577=CARTESIAN_POINT ( 'NONE',  ( -61.56765823437498852, 9.786458332991934128, 2.248837904296538515 ) ) ;
#579=CARTESIAN_POINT ( 'NONE',  ( -61.99999999999998579, 14.18750000000000000, 2.500000000000002665 ) ) ;
#581=CARTESIAN_POINT ( 'NONE',  ( -61.56765823437498142, 11.68229166632526805, 0.7511620957034663704 ) ) ;
#582=CARTESIAN_POINT ( 'NONE',  ( -62.43234176562498305, 14.72395833299193413, 0.7511620957034662593 ) ) ;
#584=CARTESIAN_POINT ( 'NONE',  ( -62.49999999999998579, 13.55208333265053433, 0.6339745962155627357 ) ) ;
#585=CARTESIAN_POINT ( 'NONE',  ( -61.49999999999998579, 16.17708333265053255, 2.366025403784441927 ) ) ;
#590=CARTESIAN_POINT ( 'NONE',  ( -60.99999999999998579, 15.23958333265053611, 0.9226497308103762673 ) ) ;
#593=CARTESIAN_POINT ( 'NONE',  ( -61.13531646874998415, 14.07812499965860198, 1.500000000000002220 ) ) ;
#594=CARTESIAN_POINT ( 'NONE',  ( -61.99999999999998579, 10.14062499965860198, 0.5015494609379544944 ) ) ;
#597=CARTESIAN_POINT ( 'NONE',  ( -62.99999999999998579, 14.12499999999999822, 1.500000000000001998 ) ) ;
#598=CARTESIAN_POINT ( 'NONE',  ( -61.99999999999998579, 13.40624999931720041, 2.500000000000002665 ) ) ;
#601=CARTESIAN_POINT ( 'NONE',  ( -61.99999999999998579, 11.53124999931720396, 0.3452994616207497591 ) ) ;
#602=EDGE_CURVE ( 'NONE', #6810, #5402, #2367, .T. ) ;
#603=DIRECTION ( 'NONE',  ( 0.000000000000000000, 0.000000000000000000, -1.000000000000000000 ) ) ;
#605=CARTESIAN_POINT ( 'NONE',  ( -61.99999999999998579, 13.89062499965860198, 0.5015494609379544944 ) ) ;
#606=LINE ( 'NONE', #2414, #9719 ) ;
#607=VERTEX_POINT ( 'NONE', #3951 ) ;
#608=CARTESIAN_POINT ( 'NONE',  ( -61.13531646874998415, 12.11979166632526628, 1.999225269531026417 ) ) ;
#609=CARTESIAN_POINT ( 'NONE',  ( -61.99999999999998579, 16.00000000000000000, 1.500000000000002220 ) ) ;
#612=EDGE_LOOP ( 'NONE', ( #5930, #4640, #8433, #5603 ) ) ;
#613=LINE ( 'NONE', #4764, #9060 ) ;
#617=CARTESIAN_POINT ( 'NONE',  ( -61.49999999999998579, 9.458333333333332149, 2.366025403784441927 ) ) ;
#619=CARTESIAN_POINT ( 'NONE',  ( -61.13531646874998415, 8.161458332991935904, 1.000774730468978468 ) ) ;
#620=CARTESIAN_POINT ( 'NONE',  ( -61.99999999999998579, 14.90624999931720218, 2.500000000000002665 ) ) ;
#621=( BOUNDED_CURVE ( )  B_SPLINE_CURVE ( 2, ( #8138, #7301, #6474, #4787, #7352, #7561, #3283, #6631, #630 ),
 .UNSPECIFIED., .F., .T. ) 
 B_SPLINE_CURVE_WITH_KNOTS ( ( 3, 2, 2, 2, 3 ),
 ( 0.4296875000000000555, 0.4322916666666666852, 0.4375000000000000000, 0.4427083333333333148, 0.4453125000000000000 ),
 .UNSPECIFIED. ) 
 CURVE ( )  GEOMETRIC_REPRESENTATION_ITEM ( )  RATIONAL_B_SPLINE_CURVE ( ( 0.9330127018922192983, 0.9330127018922207416, 1.000000000000000000, 0.8660254037844387076, 1.000000000000000000, 0.8660254037844387076, 1.000000000000000000, 0.9330127018922194093, 0.9330127018922194093 ) ) 
 REPRESENTATION_ITEM ( '' )  );
#622=CARTESIAN_POINT ( 'NONE',  ( -61.99999999999998579, 8.406249999317202182, 2.654700538379254571 ) ) ;
#623=CARTESIAN_POINT ( 'NONE',  ( -61.13531646874998415, 12.11979166632526628, 1.999225269531026417 ) ) ;
#625=CARTESIAN_POINT ( 'NONE',  ( -61.99999999999998579, 8.000000000000000000, 0.5000000000000041078 ) ) ;
#628=CARTESIAN_POINT ( 'NONE',  ( -61.13531646874998415, 13.84895833299193413, 1.000774730468978468 ) ) ;
#630=CARTESIAN_POINT ( 'NONE',  ( -61.99999999999998579, 11.78124999931720218, 0.5000000000000013323 ) ) ;
#632=CARTESIAN_POINT ( 'NONE',  ( -62.86468353124998032, 11.99479166632526628, 1.000774730468978024 ) ) ;
#633=CARTESIAN_POINT ( 'NONE',  ( -61.56765823437498852, 15.09895833299193590, 2.248837904296538515 ) ) ;
#635=CARTESIAN_POINT ( 'NONE',  ( -62.43234176562498305, 8.473958332991934128, 0.7511620957034662593 ) ) ;
#636=CARTESIAN_POINT ( 'NONE',  ( -62.49999999999998579, 10.33333333333333393, 0.6339745962155627357 ) ) ;
#637=ORIENTED_EDGE ( 'NONE', *, *, #7042, .T. ) ;
#638=CARTESIAN_POINT ( 'NONE',  ( -62.49999999999998579, 11.80208333265053611, 0.6339745962155627357 ) ) ;
#641=CARTESIAN_POINT ( 'NONE',  ( -62.43234176562499016, 13.74479166632526805, 2.248837904296538071 ) ) ;
#642=CARTESIAN_POINT ( 'NONE',  ( -62.86468353124998742, 10.22395833299193413, 1.999225269531025972 ) ) ;
#645=CARTESIAN_POINT ( 'NONE',  ( -62.99999999999998579, 13.12500000000000178, 1.500000000000001998 ) ) ;
#646=EDGE_CURVE ( 'NONE', #607, #3158, #4934, .T. ) ;
#647=CARTESIAN_POINT ( 'NONE',  ( -62.49999999999998579, 13.30208333265053433, 0.6339745962155627357 ) ) ;
#648=CARTESIAN_POINT ( 'NONE',  ( -62.99999999999998579, 11.32291666598386826, 0.9226497308103756012 ) ) ;
#649=CARTESIAN_POINT ( 'NONE',  ( -61.56765823437498852, 14.03645833299193413, 2.248837904296538515 ) ) ;
#652=CARTESIAN_POINT ( 'NONE',  ( -61.99999999999998579, 11.45312499965860020, 0.5015494609379544944 ) ) ;
#653=CARTESIAN_POINT ( 'NONE',  ( -60.99999999999998579, 12.21874999931720218, 1.500000000000002220 ) ) ;
#654=CARTESIAN_POINT ( 'NONE',  ( -61.13531646874998415, 15.41145833299193413, 1.000774730468978468 ) ) ;
#659=ORIENTED_EDGE ( 'NONE', *, *, #9592, .T. ) ;
#660=CARTESIAN_POINT ( 'NONE',  ( -61.49999999999998579, 8.677083332650536107, 2.366025403784441927 ) ) ;
#661=CARTESIAN_POINT ( 'NONE',  ( -62.49999999999998579, 9.166666666666666075, 2.366025403784441483 ) ) ;
#662=CARTESIAN_POINT ( 'NONE',  ( -61.49999999999998579, 8.541666666666666075, 0.6339745962155628467 ) ) ;
#663=CARTESIAN_POINT ( 'NONE',  ( -61.99999999999998579, 10.53124999931720396, 0.5000000000000013323 ) ) ;
#664=CARTESIAN_POINT ( 'NONE',  ( -62.43234176562499016, 11.55729166632526805, 2.248837904296538071 ) ) ;
#665=CARTESIAN_POINT ( 'NONE',  ( -62.26794919243111082, 14.54241454900183150, 0.5000000000000013323 ) ) ;
#671=CARTESIAN_POINT ( 'NONE',  ( -62.43234176562498305, 13.41145833299193413, 0.7511620957034662593 ) ) ;
#674=( BOUNDED_CURVE ( )  B_SPLINE_CURVE ( 2, ( #2327, #7336, #4041, #563, #4820, #3995, #2377, #9107, #2277 ),
 .UNSPECIFIED., .F., .T. ) 
 B_SPLINE_CURVE_WITH_KNOTS ( ( 3, 2, 2, 2, 3 ),
 ( 0.1953124999999999445, 0.1979166666666666574, 0.2031250000000000000, 0.2083333333333333426, 0.2109375000000000000 ),
 .UNSPECIFIED. ) 
 CURVE ( )  GEOMETRIC_REPRESENTATION_ITEM ( )  RATIONAL_B_SPLINE_CURVE ( ( 0.9330127018922192983, 0.9330127018922178550, 1.000000000000000000, 0.8660254037844387076, 1.000000000000000000, 0.8660254037844387076, 1.000000000000000000, 0.9330127018922194093, 0.9330127018922194093 ) ) 
 REPRESENTATION_ITEM ( '' )  );
#675=CARTESIAN_POINT ( 'NONE',  ( -62.99999999999998579, 14.10416666666666785, 0.9226497308103756012 ) ) ;
#676=CARTESIAN_POINT ( 'NONE',  ( -61.56765823437498142, 12.43229166632526805, 0.7511620957034663704 ) ) ;
#679=CARTESIAN_POINT ( 'NONE',  ( -61.56765823437498142, 15.18229166632526805, 0.7511620957034663704 ) ) ;
#681=CARTESIAN_POINT ( 'NONE',  ( -62.26794919243111082, 15.07366454968462932, 0.5000000000000013323 ) ) ;
#682=CARTESIAN_POINT ( 'NONE',  ( -62.86468353124998032, 8.244791666325268054, 1.000774730468978246 ) ) ;
#684=CARTESIAN_POINT ( 'NONE',  ( -61.99999999999998579, 10.43750000000000000, 2.500000000000002665 ) ) ;
#689=CARTESIAN_POINT ( 'NONE',  ( -61.56765823437498142, 14.36979166632526983, 0.7511620957034663704 ) ) ;
#690=CARTESIAN_POINT ( 'NONE',  ( -62.86468353124998032, 9.932291666325269830, 1.000774730468978246 ) ) ;
#691=CARTESIAN_POINT ( 'NONE',  ( -61.13531646874997705, 15.16145833299193590, 1.000774730468978468 ) ) ;
#695=CARTESIAN_POINT ( 'NONE',  ( -62.99999999999998579, 13.62500000000000000, 1.500000000000001998 ) ) ;
#697=EDGE_CURVE ( 'NONE', #5580, #8781, #5764, .T. ) ;
#700=CARTESIAN_POINT ( 'NONE',  ( -62.49999999999998579, 12.30208333265053611, 0.6339745962155627357 ) ) ;
#703=EDGE_CURVE ( 'NONE', #827, #5087, #9117, .T. ) ;
#704=CARTESIAN_POINT ( 'NONE',  ( -61.13531646874998415, 14.59895833299193590, 1.000774730468978468 ) ) ;
#705=CARTESIAN_POINT ( 'NONE',  ( -61.73205080756886076, 11.55133545031537068, 0.5000000000000014433 ) ) ;
#706=VECTOR ( 'NONE', #9292, 1000.000000000000000 ) ;
#707=ORIENTED_EDGE ( 'NONE', *, *, #7222, .T. ) ;
#708=CARTESIAN_POINT ( 'NONE',  ( -61.56765823437498142, 12.18229166632526628, 0.7511620957034663704 ) ) ;
#709=CARTESIAN_POINT ( 'NONE',  ( -61.99999999999998579, 11.53124999931720218, 0.5000000000000013323 ) ) ;
#711=DIRECTION ( 'NONE',  ( -0.000000000000000000, -1.000000000000000000, -0.000000000000000000 ) ) ;
#714=CARTESIAN_POINT ( 'NONE',  ( -61.56765823437498142, 15.36979166632526805, 0.7511620957034663704 ) ) ;
#717=CARTESIAN_POINT ( 'NONE',  ( -62.99999999999998579, 10.60416666666666607, 0.9226497308103756012 ) ) ;
#718=FACE_OUTER_BOUND ( 'NONE', #3346, .T. ) ;
#720=CARTESIAN_POINT ( 'NONE',  ( -61.99999999999998579, 9.156249999317202182, 2.654700538379254571 ) ) ;
#721=CARTESIAN_POINT ( 'NONE',  ( -62.43234176562498305, 11.97395833299193413, 0.7511620957034662593 ) ) ;
#722=EDGE_CURVE ( 'NONE', #7043, #3002, #2720, .T. ) ;
#723=CARTESIAN_POINT ( 'NONE',  ( -62.49999999999998579, 14.63541666598387003, 2.366025403784441483 ) ) ;
#728=CARTESIAN_POINT ( 'NONE',  ( -61.13531646874998415, 14.34895833299193413, 1.000774730468978468 ) ) ;
#732=CARTESIAN_POINT ( 'NONE',  ( -61.13531646874998415, 13.14062499965860198, 1.500000000000002220 ) ) ;
#733=CARTESIAN_POINT ( 'NONE',  ( -62.86468353124999453, 15.01562499965860020, 1.500000000000002220 ) ) ;
#736=CARTESIAN_POINT ( 'NONE',  ( -62.49999999999998579, 15.80208333265053788, 0.6339745962155627357 ) ) ;
#737=CARTESIAN_POINT ( 'NONE',  ( -61.99999999999998579, 16.00000000000000000, 1.500000000000002220 ) ) ;
#742=( BOUNDED_CURVE ( )  B_SPLINE_CURVE ( 2, ( #3926, #8157, #8263, #9979, #10644, #4696, #7423, #8104, #2361 ),
 .UNSPECIFIED., .F., .T. ) 
 B_SPLINE_CURVE_WITH_KNOTS ( ( 3, 2, 2, 2, 3 ),
 ( 0.3515625000000000000, 0.3541666666666666852, 0.3593750000000000000, 0.3645833333333333148, 0.3671875000000000000 ),
 .UNSPECIFIED. ) 
 CURVE ( )  GEOMETRIC_REPRESENTATION_ITEM ( )  RATIONAL_B_SPLINE_CURVE ( ( 0.9330127018922194093, 0.9330127018922194093, 1.000000000000000000, 0.8660254037844387076, 1.000000000000000000, 0.8660254037844387076, 1.000000000000000000, 0.9330127018922194093, 0.9330127018922194093 ) ) 
 REPRESENTATION_ITEM ( '' )  );
#744=CARTESIAN_POINT ( 'NONE',  ( -62.43234176562499016, 13.99479166632526805, 2.248837904296538071 ) ) ;
#745=CARTESIAN_POINT ( 'NONE',  ( -61.13531646874998415, 9.807291666325268054, 1.999225269531026417 ) ) ;
#746=CARTESIAN_POINT ( 'NONE',  ( -61.99999999999999289, 16.07812499965860198, 2.498450539062049724 ) ) ;
#747=CARTESIAN_POINT ( 'NONE',  ( -61.73205080756886076, 14.41741454900183150, 2.500000000000003109 ) ) ;
#748=ORIENTED_EDGE ( 'NONE', *, *, #4906, .F. ) ;
#749=CARTESIAN_POINT ( 'NONE',  ( -61.99999999999998579, 13.56250000000000000, 0.3452994616207497591 ) ) ;
#750=CARTESIAN_POINT ( 'NONE',  ( -62.43234176562498305, 9.223958332991935904, 0.7511620957034662593 ) ) ;
#751=CARTESIAN_POINT ( 'NONE',  ( -62.49999999999998579, 11.55208333265053611, 0.6339745962155627357 ) ) ;
#752=AXIS2_PLACEMENT_3D ( 'NONE', #1956, #4720, #7126 ) ;
#754=CARTESIAN_POINT ( 'NONE',  ( -61.99999999999998579, 10.93750000000000000, 2.500000000000002665 ) ) ;
#755=CARTESIAN_POINT ( 'NONE',  ( -61.13531646874998415, 13.30729166632526983, 1.999225269531026417 ) ) ;
#757=EDGE_LOOP ( 'NONE', ( #9977, #1342, #4104, #2542 ) ) ;
#758=AXIS2_PLACEMENT_3D ( 'NONE', #10274, #3559, #3502 ) ;
#759=CIRCLE ( 'NONE', #7138, 0.9999999999999983347 ) ;
#760=CARTESIAN_POINT ( 'NONE',  ( -61.99999999999998579, 13.32812499965860198, 2.498450539062049724 ) ) ;
#763=ORIENTED_EDGE ( 'NONE', *, *, #2423, .F. ) ;
#765=ORIENTED_EDGE ( 'NONE', *, *, #9254, .T. ) ;
#766=CARTESIAN_POINT ( 'NONE',  ( -62.49999999999998579, 11.16666666666666607, 2.366025403784441483 ) ) ;
#768=CARTESIAN_POINT ( 'NONE',  ( -60.99999999999998579, 8.520833333333333925, 0.9226497308103762673 ) ) ;
#769=CARTESIAN_POINT ( 'NONE',  ( -62.99999999999998579, 15.85416666666666607, 0.9226497308103756012 ) ) ;
#773=CARTESIAN_POINT ( 'NONE',  ( -61.13531646874998415, 13.61979166632526983, 1.999225269531026417 ) ) ;
#775=ORIENTED_EDGE ( 'NONE', *, *, #4849, .F. ) ;
#776=CARTESIAN_POINT ( 'NONE',  ( -61.49999999999998579, 11.01041666598386826, 0.6339745962155628467 ) ) ;
#778=CARTESIAN_POINT ( 'NONE',  ( -61.99999999999998579, 14.28124999931720218, 0.5000000000000013323 ) ) ;
#779=CARTESIAN_POINT ( 'NONE',  ( -61.13531646874998415, 14.55729166632526628, 1.999225269531026417 ) ) ;
#783=CARTESIAN_POINT ( 'NONE',  ( -61.99999999999999289, 12.70312499965860198, 0.5015494609379544944 ) ) ;
#784=CARTESIAN_POINT ( 'NONE',  ( -62.86468353124998032, 14.99479166632526805, 1.000774730468978246 ) ) ;
#787=CARTESIAN_POINT ( 'NONE',  ( -61.13531646874998415, 8.911458332991934128, 1.000774730468978468 ) ) ;
#788=FACE_OUTER_BOUND ( 'NONE', #1381, .T. ) ;
#791=CARTESIAN_POINT ( 'NONE',  ( -61.99999999999998579, 16.00000000000000000, 1.500000000000002220 ) ) ;
#792=EDGE_CURVE ( 'NONE', #4570, #3615, #389, .T. ) ;
#793=CARTESIAN_POINT ( 'NONE',  ( -61.56765823437498852, 14.03645833299193413, 2.248837904296538515 ) ) ;
#794=CARTESIAN_POINT ( 'NONE',  ( -61.99999999999998579, 11.76562499965860198, 2.498450539062049724 ) ) ;
#796=CARTESIAN_POINT ( 'NONE',  ( -61.99999999999999289, 15.32812499965860198, 2.498450539062049724 ) ) ;
#797=CARTESIAN_POINT ( 'NONE',  ( -61.49999999999998579, 14.42708333265053611, 2.366025403784441927 ) ) ;
#799=CARTESIAN_POINT ( 'NONE',  ( -61.99999999999998579, 13.43749999999999822, 2.654700538379254571 ) ) ;
#800=CARTESIAN_POINT ( 'NONE',  ( -62.86468353124999453, 8.265624999658601979, 1.500000000000002220 ) ) ;
#801=EDGE_CURVE ( 'NONE', #5222, #6754, #4636, .T. ) ;
#802=CARTESIAN_POINT ( 'NONE',  ( -60.99999999999998579, 12.94791666598387003, 2.077350269189628840 ) ) ;
#804=CARTESIAN_POINT ( 'NONE',  ( -61.99999999999998579, 9.437499999999998224, 2.500000000000002665 ) ) ;
#805=( BOUNDED_CURVE ( )  B_SPLINE_CURVE ( 2, ( #6919, #4287, #1801, #9519, #7697, #5285, #9408, #246, #76 ),
 .UNSPECIFIED., .F., .T. ) 
 B_SPLINE_CURVE_WITH_KNOTS ( ( 3, 2, 2, 2, 3 ),
 ( 0.2109375000000000000, 0.2135416666666666574, 0.2187500000000000000, 0.2239583333333333426, 0.2265625000000000000 ),
 .UNSPECIFIED. ) 
 CURVE ( )  GEOMETRIC_REPRESENTATION_ITEM ( )  RATIONAL_B_SPLINE_CURVE ( ( 0.9330127018922194093, 0.9330127018922194093, 1.000000000000000000, 0.8660254037844387076, 1.000000000000000000, 0.8660254037844387076, 1.000000000000000000, 0.9330127018922194093, 0.9330127018922194093 ) ) 
 REPRESENTATION_ITEM ( '' )  );
#806=CARTESIAN_POINT ( 'NONE',  ( -61.13531646874998415, 14.07812499965860198, 1.500000000000002220 ) ) ;
#807=ORIENTED_EDGE ( 'NONE', *, *, #3016, .T. ) ;
#809=CARTESIAN_POINT ( 'NONE',  ( -62.43234176562498305, 12.72395833299193413, 0.7511620957034662593 ) ) ;
#810=CYLINDRICAL_SURFACE ( 'NONE', #2113, 0.9999999999999981126 ) ;
#811=EDGE_CURVE ( 'NONE', #6260, #5909, #3801, .T. ) ;
#815=CARTESIAN_POINT ( 'NONE',  ( -61.49999999999998579, 14.70833333333333393, 2.366025403784441927 ) ) ;
#817=CARTESIAN_POINT ( 'NONE',  ( -60.99999999999998579, 11.52083333333333393, 0.9226497308103762673 ) ) ;
#818=ORIENTED_EDGE ( 'NONE', *, *, #2165, .F. ) ;
#819=CARTESIAN_POINT ( 'NONE',  ( -61.13531646874998415, 8.661458332991935904, 1.000774730468978468 ) ) ;
#820=DIRECTION ( 'NONE',  ( -0.000000000000000000, -1.000000000000000000, -0.000000000000000000 ) ) ;
#821=EDGE_CURVE ( 'NONE', #7309, #7701, #10603, .T. ) ;
#822=CARTESIAN_POINT ( 'NONE',  ( -61.13531646874998415, 13.39062499965860020, 1.500000000000002220 ) ) ;
#823=CARTESIAN_POINT ( 'NONE',  ( -61.73205080756885366, 8.270085449632572860, 0.5000000000000027756 ) ) ;
#827=VERTEX_POINT ( 'NONE', #6776 ) ;
#828=CARTESIAN_POINT ( 'NONE',  ( -60.99999999999998579, 12.75000000000000178, 1.500000000000002220 ) ) ;
#829=CARTESIAN_POINT ( 'NONE',  ( -61.99999999999998579, 15.39062499965860198, 0.5015494609379544944 ) ) ;
#830=CARTESIAN_POINT ( 'NONE',  ( -60.99999999999998579, 16.00000000000000000, 1.500000000000002220 ) ) ;
#832=CARTESIAN_POINT ( 'NONE',  ( -62.43234176562499016, 13.05729166632526805, 2.248837904296538071 ) ) ;
#833=CARTESIAN_POINT ( 'NONE',  ( -61.56765823437498852, 15.34895833299193590, 2.248837904296538515 ) ) ;
#834=CARTESIAN_POINT ( 'NONE',  ( -61.99999999999998579, 16.00000000000000000, 1.500000000000002220 ) ) ;
#835=CARTESIAN_POINT ( 'NONE',  ( -61.99999999999998579, 8.812500000000000000, 0.5000000000000013323 ) ) ;
#837=CARTESIAN_POINT ( 'NONE',  ( -62.86468353124998742, 9.536458332991935904, 1.999225269531025972 ) ) ;
#838=DIRECTION ( 'NONE',  ( 0.000000000000000000, 0.000000000000000000, -1.000000000000000000 ) ) ;
#841=CARTESIAN_POINT ( 'NONE',  ( -62.99999999999998579, 12.64583333333333393, 2.077350269189627952 ) ) ;
#842=CARTESIAN_POINT ( 'NONE',  ( -61.56765823437498142, 15.11979166632526805, 0.7511620957034663704 ) ) ;
#843=CARTESIAN_POINT ( 'NONE',  ( -61.56765823437498142, 11.61979166632526805, 0.7511620957034663704 ) ) ;
#845=CARTESIAN_POINT ( 'NONE',  ( -62.43234176562498305, 15.47395833299193590, 0.7511620957034662593 ) ) ;
#848=CARTESIAN_POINT ( 'NONE',  ( -60.99999999999998579, 14.47916666666666607, 2.077350269189628840 ) ) ;
#849=CARTESIAN_POINT ( 'NONE',  ( -61.13531646874998415, 8.140624999658601979, 1.500000000000002220 ) ) ;
#852=CARTESIAN_POINT ( 'NONE',  ( -60.99999999999998579, 12.96874999931720396, 1.500000000000002220 ) ) ;
#857=CARTESIAN_POINT ( 'NONE',  ( -62.86468353124998032, 12.18229166632526628, 1.000774730468978024 ) ) ;
#858=ORIENTED_EDGE ( 'NONE', *, *, #4449, .T. ) ;
#860=CARTESIAN_POINT ( 'NONE',  ( -61.13531646874998415, 13.41145833299193235, 1.000774730468978468 ) ) ;
#861=CARTESIAN_POINT ( 'NONE',  ( -61.06765823437498852, 16.03906249982930277, 1.500000000000002220 ) ) ;
#864=CARTESIAN_POINT ( 'NONE',  ( -61.99999999999998579, 9.281249999317202182, 0.5000000000000013323 ) ) ;
#867=VECTOR ( 'NONE', #10902, 1000.000000000000000 ) ;
#868=ADVANCED_FACE ( 'NONE', ( #4599 ), #2169, .T. ) ;
#869=VERTEX_POINT ( 'NONE', #5544 ) ;
#871=CARTESIAN_POINT ( 'NONE',  ( -62.43234176562499016, 8.557291666325268054, 2.248837904296538071 ) ) ;
#872=CARTESIAN_POINT ( 'NONE',  ( -60.99999999999998579, 14.22916666666666785, 2.077350269189628840 ) ) ;
#874=CARTESIAN_POINT ( 'NONE',  ( -62.43234176562499016, 13.55729166632526805, 2.248837904296538071 ) ) ;
#876=CARTESIAN_POINT ( 'NONE',  ( -62.99999999999998579, 12.84374999931720396, 1.500000000000001998 ) ) ;
#878=CARTESIAN_POINT ( 'NONE',  ( -61.49999999999998579, 10.92708333265053611, 2.366025403784441927 ) ) ;
#879=AXIS2_PLACEMENT_3D ( 'NONE', #2223, #3056, #5655 ) ;
#881=CARTESIAN_POINT ( 'NONE',  ( -62.26794919243111082, 11.54241454900183150, 0.5000000000000013323 ) ) ;
#882=CARTESIAN_POINT ( 'NONE',  ( -61.99999999999998579, 14.64062499965860020, 0.5015494609379544944 ) ) ;
#884=CARTESIAN_POINT ( 'NONE',  ( -61.99999999999998579, 12.40624999931720218, 2.500000000000002665 ) ) ;
#885=CARTESIAN_POINT ( 'NONE',  ( -61.73205080756886076, 10.80133545031537068, 0.5000000000000014433 ) ) ;
#886=CARTESIAN_POINT ( 'NONE',  ( -61.56765823437498852, 12.34895833299193413, 2.248837904296538515 ) ) ;
#887=CARTESIAN_POINT ( 'NONE',  ( -62.43234176562498305, 8.661458332991934128, 0.7511620957034662593 ) ) ;
#889=CARTESIAN_POINT ( 'NONE',  ( -62.43234176562498305, 8.973958332991934128, 0.7511620957034662593 ) ) ;
#890=CARTESIAN_POINT ( 'NONE',  ( -61.73205080756886076, 15.66741454900183506, 2.500000000000003109 ) ) ;
#893=CARTESIAN_POINT ( 'NONE',  ( -61.99999999999998579, 16.00000000000000000, 1.500000000000002220 ) ) ;
#894=CARTESIAN_POINT ( 'NONE',  ( -62.86468353124999453, 15.45312499965860020, 1.500000000000002220 ) ) ;
#895=CARTESIAN_POINT ( 'NONE',  ( -61.13531646874998415, 11.84895833299193413, 1.000774730468978468 ) ) ;
#896=CARTESIAN_POINT ( 'NONE',  ( -62.86468353124998032, 15.24479166632526805, 1.000774730468978024 ) ) ;
#899=CARTESIAN_POINT ( 'NONE',  ( -62.99999999999998579, 14.62500000000000000, 1.500000000000001998 ) ) ;
#900=CARTESIAN_POINT ( 'NONE',  ( -61.99999999999999289, 8.453124999658601979, 0.5015494609379544944 ) ) ;
#901=EDGE_CURVE ( 'NONE', #10100, #8518, #3651, .T. ) ;
#902=CARTESIAN_POINT ( 'NONE',  ( -61.49999999999998579, 13.01041666598386826, 0.6339745962155628467 ) ) ;
#904=CARTESIAN_POINT ( 'NONE',  ( -61.99999999999998579, 11.31250000000000000, 0.5000000000000013323 ) ) ;
#906=CARTESIAN_POINT ( 'NONE',  ( -62.86468353124999453, 10.97395833299193413, 1.999225269531025750 ) ) ;
#909=ORIENTED_EDGE ( 'NONE', *, *, #963, .T. ) ;
#910=CARTESIAN_POINT ( 'NONE',  ( -62.99999999999998579, 12.89583333333333037, 2.077350269189627952 ) ) ;
#912=CARTESIAN_POINT ( 'NONE',  ( -61.56765823437498142, 13.18229166632526805, 0.7511620957034663704 ) ) ;
#913=CARTESIAN_POINT ( 'NONE',  ( -61.99999999999998579, 16.00000000000000000, 2.500000000000000444 ) ) ;
#915=CARTESIAN_POINT ( 'NONE',  ( -62.49999999999998579, 9.885416665983870033, 2.366025403784441483 ) ) ;
#916=ORIENTED_EDGE ( 'NONE', *, *, #2745, .F. ) ;
#918=VERTEX_POINT ( 'NONE', #9716 ) ;
#919=CARTESIAN_POINT ( 'NONE',  ( -60.99999999999998579, 14.72916666666666607, 2.077350269189628840 ) ) ;
#920=CARTESIAN_POINT ( 'NONE',  ( -62.43234176562498305, 10.66145833299193413, 0.7511620957034662593 ) ) ;
#923=ORIENTED_EDGE ( 'NONE', *, *, #6486, .F. ) ;
#925=CARTESIAN_POINT ( 'NONE',  ( -61.99999999999998579, 9.453124999658600203, 0.5015494609379544944 ) ) ;
#926=CARTESIAN_POINT ( 'NONE',  ( -62.99999999999998579, 13.82291666598387003, 0.9226497308103756012 ) ) ;
#929=CARTESIAN_POINT ( 'NONE',  ( -62.86468353124998032, 13.49479166632526805, 1.000774730468978246 ) ) ;
#934=VECTOR ( 'NONE', #6411, 1000.000000000000000 ) ;
#935=CARTESIAN_POINT ( 'NONE',  ( -62.49999999999998579, 11.63541666598387003, 2.366025403784441483 ) ) ;
#936=CARTESIAN_POINT ( 'NONE',  ( -61.56765823437498852, 14.53645833299193413, 2.248837904296538515 ) ) ;
#938=CARTESIAN_POINT ( 'NONE',  ( -60.99999999999998579, 12.47916666666666785, 2.077350269189628840 ) ) ;
#940=CARTESIAN_POINT ( 'NONE',  ( -61.99999999999999289, 14.07812499965860020, 2.498450539062049724 ) ) ;
#941=CARTESIAN_POINT ( 'NONE',  ( -62.86468353124999453, 8.453124999658601979, 1.500000000000002220 ) ) ;
#942=CARTESIAN_POINT ( 'NONE',  ( -61.99999999999998579, 16.00000000000000000, 1.500000000000002220 ) ) ;
#945=CARTESIAN_POINT ( 'NONE',  ( -62.86468353124998742, 9.286458332991934128, 1.999225269531025972 ) ) ;
#947=VERTEX_POINT ( 'NONE', #1277 ) ;
#950=CARTESIAN_POINT ( 'NONE',  ( -61.56765823437498852, 15.78645833299193590, 2.248837904296538515 ) ) ;
#951=CARTESIAN_POINT ( 'NONE',  ( -61.13531646874998415, 10.55729166632526805, 1.999225269531026417 ) ) ;
#952=CARTESIAN_POINT ( 'NONE',  ( -62.43234176562499016, 9.494791666325268054, 2.248837904296538071 ) ) ;
#954=CARTESIAN_POINT ( 'NONE',  ( -62.99999999999998579, 14.85416666666666607, 0.9226497308103756012 ) ) ;
#955=CARTESIAN_POINT ( 'NONE',  ( -61.99999999999999289, 10.70312499965860198, 0.5015494609379544944 ) ) ;
#957=CARTESIAN_POINT ( 'NONE',  ( -61.99999999999998579, 12.90624999931720396, 2.654700538379254571 ) ) ;
#958=CARTESIAN_POINT ( 'NONE',  ( -62.49999999999998579, 13.16666666666666607, 2.366025403784441483 ) ) ;
#959=( BOUNDED_CURVE ( )  B_SPLINE_CURVE ( 2, ( #8529, #966, #8702, #10294, #191, #3522, #4402, #10355, #8759 ),
 .UNSPECIFIED., .F., .T. ) 
 B_SPLINE_CURVE_WITH_KNOTS ( ( 3, 2, 2, 2, 3 ),
 ( 0.6171875000000000000, 0.6197916666666666297, 0.6250000000000000000, 0.6302083333333333703, 0.6328125000000000000 ),
 .UNSPECIFIED. ) 
 CURVE ( )  GEOMETRIC_REPRESENTATION_ITEM ( )  RATIONAL_B_SPLINE_CURVE ( ( 0.9330127018922194093, 0.9330127018922194093, 1.000000000000000000, 0.8660254037844387076, 1.000000000000000000, 0.8660254037844387076, 1.000000000000000000, 0.9330127018922194093, 0.9330127018922194093 ) ) 
 REPRESENTATION_ITEM ( '' )  );
#962=CARTESIAN_POINT ( 'NONE',  ( -61.99999999999999289, 11.89062499965860553, 0.5015494609379544944 ) ) ;
#963=EDGE_CURVE ( 'NONE', #2018, #6810, #1525, .T. ) ;
#965=DIRECTION ( 'NONE',  ( -0.000000000000000000, -1.000000000000000000, -0.000000000000000000 ) ) ;
#966=CARTESIAN_POINT ( 'NONE',  ( -61.73205080756886076, 12.94866454968462932, 2.500000000000003109 ) ) ;
#967=EDGE_LOOP ( 'NONE', ( #3059, #1127, #10448, #2159 ) ) ;
#969=CARTESIAN_POINT ( 'NONE',  ( -61.56765823437498852, 12.34895833299193413, 2.248837904296538515 ) ) ;
#971=CARTESIAN_POINT ( 'NONE',  ( -62.26794919243111082, 13.82366454968463110, 0.5000000000000013323 ) ) ;
#972=CARTESIAN_POINT ( 'NONE',  ( -62.99999999999998579, 9.843749999317202182, 1.500000000000001998 ) ) ;
#975=CARTESIAN_POINT ( 'NONE',  ( -61.99999999999998579, 16.00000000000000000, 1.500000000000002220 ) ) ;
#976=CARTESIAN_POINT ( 'NONE',  ( -62.43234176562498305, 11.16145833299193590, 0.7511620957034662593 ) ) ;
#977=ORIENTED_EDGE ( 'NONE', *, *, #9014, .T. ) ;
#978=CARTESIAN_POINT ( 'NONE',  ( -62.86468353124999453, 9.265624999658600203, 1.500000000000002220 ) ) ;
#981=CARTESIAN_POINT ( 'NONE',  ( -62.86468353124998032, 14.99479166632526805, 1.000774730468978246 ) ) ;
#982=CARTESIAN_POINT ( 'NONE',  ( -62.99999999999998579, 9.343749999317202182, 1.500000000000001998 ) ) ;
#986=EDGE_LOOP ( 'NONE', ( #1772, #5582, #9425, #3019 ) ) ;
#987=CARTESIAN_POINT ( 'NONE',  ( -61.99999999999998579, 13.15624999931720218, 2.500000000000002665 ) ) ;
#988=CARTESIAN_POINT ( 'NONE',  ( -60.99999999999998579, 8.250000000000000000, 1.500000000000002220 ) ) ;
#990=CARTESIAN_POINT ( 'NONE',  ( -60.99999999999998579, 12.52083333333333215, 0.9226497308103762673 ) ) ;
#992=CARTESIAN_POINT ( 'NONE',  ( -61.13531646874997705, 14.11979166632526805, 1.999225269531026417 ) ) ;
#993=CARTESIAN_POINT ( 'NONE',  ( -61.99999999999998579, 8.640624999658601979, 0.5015494609379544944 ) ) ;
#996=CARTESIAN_POINT ( 'NONE',  ( -62.86468353124999453, 9.765624999658601979, 1.500000000000002220 ) ) ;
#1000=FACE_OUTER_BOUND ( 'NONE', #6370, .T. ) ;
#1002=CARTESIAN_POINT ( 'NONE',  ( -61.56765823437498852, 16.03645833299193768, 2.248837904296538515 ) ) ;
#1003=EDGE_CURVE ( 'NONE', #6871, #7309, #7220, .T. ) ;
#1004=CARTESIAN_POINT ( 'NONE',  ( -62.86468353124999453, 11.45312499965860020, 1.500000000000002220 ) ) ;
#1005=CARTESIAN_POINT ( 'NONE',  ( -61.56765823437498852, 8.286458332991934128, 2.248837904296538515 ) ) ;
#1007=CARTESIAN_POINT ( 'NONE',  ( -61.49999999999998579, 15.29166666666666607, 0.6339745962155628467 ) ) ;
#1008=CARTESIAN_POINT ( 'NONE',  ( -61.99999999999999289, 10.20312499965860198, 0.5015494609379544944 ) ) ;
#1011=CARTESIAN_POINT ( 'NONE',  ( -62.99999999999998579, 13.11458333265053433, 2.077350269189627952 ) ) ;
#1012=CARTESIAN_POINT ( 'NONE',  ( -62.26794919243111082, 13.17633545031536890, 2.500000000000003109 ) ) ;
#1014=DIRECTION ( 'NONE',  ( 0.000000000000000000, 0.000000000000000000, -1.000000000000000000 ) ) ;
#1015=AXIS2_PLACEMENT_3D ( 'NONE', #7511, #8290, #2342 ) ;
#1016=CARTESIAN_POINT ( 'NONE',  ( -61.13531646874998415, 11.32812499965860020, 1.500000000000002220 ) ) ;
#1018=DIRECTION ( 'NONE',  ( 0.8660254037844418162, 0.4999999999999947264, -0.000000000000000000 ) ) ;
#1019=ORIENTED_EDGE ( 'NONE', *, *, #10039, .F. ) ;
#1020=CARTESIAN_POINT ( 'NONE',  ( -62.49999999999998579, 11.33333333333333393, 0.6339745962155627357 ) ) ;
#1022=CARTESIAN_POINT ( 'NONE',  ( -61.56765823437498142, 14.18229166632526805, 0.7511620957034663704 ) ) ;
#1023=( BOUNDED_CURVE ( )  B_SPLINE_CURVE ( 2, ( #1890, #6286, #10383, #10558, #1287, #9611, #1048, #2843, #8840 ),
 .UNSPECIFIED., .F., .F. ) 
 B_SPLINE_CURVE_WITH_KNOTS ( ( 3, 2, 2, 2, 3 ),
 ( 0.3046874999999999445, 0.3072916666666666852, 0.3125000000000000000, 0.3177083333333333148, 0.3203125000000000000 ),
 .UNSPECIFIED. ) 
 CURVE ( )  GEOMETRIC_REPRESENTATION_ITEM ( )  RATIONAL_B_SPLINE_CURVE ( ( 0.9330127018922192983, 0.9330127018922178550, 1.000000000000000000, 0.8660254037844387076, 1.000000000000000000, 0.8660254037844387076, 1.000000000000000000, 0.9330127018922194093, 0.9330127018922194093 ) ) 
 REPRESENTATION_ITEM ( '' )  );
#1026=CARTESIAN_POINT ( 'NONE',  ( -60.99999999999998579, 8.989583332650536107, 0.9226497308103762673 ) ) ;
#1031=CARTESIAN_POINT ( 'NONE',  ( -62.86468353124999453, 10.95312499965860020, 1.500000000000002220 ) ) ;
#1032=AXIS2_PLACEMENT_3D ( 'NONE', #4772, #3269, #6667 ) ;
#1034=CARTESIAN_POINT ( 'NONE',  ( -62.43234176562498305, 9.723958332991934128, 0.7511620957034662593 ) ) ;
#1035=CARTESIAN_POINT ( 'NONE',  ( -62.26794919243111082, 15.54241454900183506, 0.5000000000000013323 ) ) ;
#1036=AXIS2_PLACEMENT_3D ( 'NONE', #5926, #711, #4093 ) ;
#1037=CARTESIAN_POINT ( 'NONE',  ( -61.56765823437498852, 15.09895833299193590, 2.248837904296538515 ) ) ;
#1038=CARTESIAN_POINT ( 'NONE',  ( -61.73205080756886076, 13.30133545031536890, 0.5000000000000014433 ) ) ;
#1040=CARTESIAN_POINT ( 'NONE',  ( -61.99999999999998579, 15.31250000000000000, 0.5000000000000013323 ) ) ;
#1044=CARTESIAN_POINT ( 'NONE',  ( -61.99999999999998579, 15.89062499965860198, 0.5015494609379544944 ) ) ;
#1046=CARTESIAN_POINT ( 'NONE',  ( -61.99999999999998579, 16.00000000000000000, 1.500000000000002220 ) ) ;
#1047=CARTESIAN_POINT ( 'NONE',  ( -61.49999999999998579, 12.42708333265053611, 2.366025403784441927 ) ) ;
#1048=CARTESIAN_POINT ( 'NONE',  ( -61.49999999999998579, 10.76041666598386826, 0.6339745962155628467 ) ) ;
#1049=CARTESIAN_POINT ( 'NONE',  ( -61.13531646874997705, 14.41145833299193413, 1.000774730468978468 ) ) ;
#1050=CARTESIAN_POINT ( 'NONE',  ( -61.99999999999998579, 9.140624999658601979, 0.5015494609379544944 ) ) ;
#1054=CARTESIAN_POINT ( 'NONE',  ( -62.26794919243111082, 9.573664549684629321, 0.4999999999999998890 ) ) ;
#1055=CARTESIAN_POINT ( 'NONE',  ( -62.86468353124998032, 9.994791666325268054, 1.000774730468978246 ) ) ;
#1057=ORIENTED_EDGE ( 'NONE', *, *, #4867, .F. ) ;
#1059=DIRECTION ( 'NONE',  ( -0.000000000000000000, -1.000000000000000000, -0.000000000000000000 ) ) ;
#1060=VECTOR ( 'NONE', #10492, 1000.000000000000000 ) ;
#1062=CARTESIAN_POINT ( 'NONE',  ( -61.13531646874998415, 15.82812499965860198, 1.500000000000002220 ) ) ;
#1063=CARTESIAN_POINT ( 'NONE',  ( -61.99999999999998579, 12.26562499965860198, 2.498450539062049724 ) ) ;
#1064=CARTESIAN_POINT ( 'NONE',  ( -62.86468353124999453, 9.223958332991935904, 1.999225269531025750 ) ) ;
#1066=VERTEX_POINT ( 'NONE', #4484 ) ;
#1067=CARTESIAN_POINT ( 'NONE',  ( -60.99999999999998579, 14.52083333333333215, 0.9226497308103762673 ) ) ;
#1068=CARTESIAN_POINT ( 'NONE',  ( -61.13531646874997705, 9.869791666325266277, 1.999225269531026417 ) ) ;
#1069=CARTESIAN_POINT ( 'NONE',  ( -61.13531646874998415, 14.82812499965860020, 1.500000000000002220 ) ) ;
#1070=CARTESIAN_POINT ( 'NONE',  ( -60.99999999999998579, 14.69791666598386826, 2.077350269189628840 ) ) ;
#1071=CARTESIAN_POINT ( 'NONE',  ( -62.99999999999998579, 13.14583333333333215, 2.077350269189627952 ) ) ;
#1072=ORIENTED_EDGE ( 'NONE', *, *, #7222, .F. ) ;
#1073=ADVANCED_FACE ( 'NONE', ( #5964 ), #10913, .T. ) ;
#1074=CARTESIAN_POINT ( 'NONE',  ( -61.99999999999998579, 12.93750000000000178, 2.500000000000002665 ) ) ;
#1075=CARTESIAN_POINT ( 'NONE',  ( -62.43234176562498305, 11.91145833299193413, 0.7511620957034662593 ) ) ;
#1076=CARTESIAN_POINT ( 'NONE',  ( -62.43234176562498305, 9.161458332991935904, 0.7511620957034662593 ) ) ;
#1079=CARTESIAN_POINT ( 'NONE',  ( -62.49999999999998579, 10.83333333333333393, 0.6339745962155627357 ) ) ;
#1081=CARTESIAN_POINT ( 'NONE',  ( -62.86468353124998032, 14.49479166632526805, 1.000774730468978246 ) ) ;
#1083=CARTESIAN_POINT ( 'NONE',  ( -60.99999999999998579, 8.739583332650536107, 0.9226497308103762673 ) ) ;
#1086=CARTESIAN_POINT ( 'NONE',  ( -61.49999999999998579, 14.04166666666666785, 0.6339745962155628467 ) ) ;
#1089=CARTESIAN_POINT ( 'NONE',  ( -61.13531646874998415, 11.32812499965860020, 1.500000000000002220 ) ) ;
#1091=( BOUNDED_CURVE ( )  B_SPLINE_CURVE ( 2, ( #4781, #2016, #7067, #9850, #10450, #2236, #5617, #2964, #2851 ),
 .UNSPECIFIED., .F., .T. ) 
 B_SPLINE_CURVE_WITH_KNOTS ( ( 3, 2, 2, 2, 3 ),
 ( 0.8984375000000000000, 0.9010416666666666297, 0.9062500000000000000, 0.9114583333333333703, 0.9140625000000000000 ),
 .UNSPECIFIED. ) 
 CURVE ( )  GEOMETRIC_REPRESENTATION_ITEM ( )  RATIONAL_B_SPLINE_CURVE ( ( 0.9330127018922194093, 0.9330127018922194093, 1.000000000000000000, 0.8660254037844387076, 1.000000000000000000, 0.8660254037844387076, 1.000000000000000000, 0.9330127018922194093, 0.9330127018922194093 ) ) 
 REPRESENTATION_ITEM ( '' )  );
#1094=CARTESIAN_POINT ( 'NONE',  ( -61.13531646874998415, 9.661458332991932352, 1.000774730468978468 ) ) ;
#1095=CARTESIAN_POINT ( 'NONE',  ( -61.99999999999998579, 15.53124999931720041, 0.5000000000000013323 ) ) ;
#1097=CARTESIAN_POINT ( 'NONE',  ( -61.13531646874998415, 14.36979166632527161, 1.999225269531026417 ) ) ;
#1099=ORIENTED_EDGE ( 'NONE', *, *, #10096, .F. ) ;
#1102=CARTESIAN_POINT ( 'NONE',  ( -61.73205080756886076, 10.44866454968463110, 2.500000000000003109 ) ) ;
#1103=VECTOR ( 'NONE', #4447, 1000.000000000000000 ) ;
#1104=VERTEX_POINT ( 'NONE', #7534 ) ;
#1105=FACE_BOUND ( 'NONE', #1192, .T. ) ;
#1108=CARTESIAN_POINT ( 'NONE',  ( -61.49999999999998579, 8.458333333333333925, 2.366025403784441927 ) ) ;
#1109=DIRECTION ( 'NONE',  ( -0.000000000000000000, -1.000000000000000000, -0.000000000000000000 ) ) ;
#1113=CARTESIAN_POINT ( 'NONE',  ( -61.99999999999999289, 13.45312499965860376, 0.5015494609379544944 ) ) ;
#1114=AXIS2_PLACEMENT_3D ( 'NONE', #2207, #7091, #483 ) ;
#1115=CARTESIAN_POINT ( 'NONE',  ( -62.86468353124998742, 8.973958332991934128, 1.999225269531025972 ) ) ;
#1116=CARTESIAN_POINT ( 'NONE',  ( -61.99999999999998579, 9.687500000000000000, 2.500000000000002665 ) ) ;
#1117=CARTESIAN_POINT ( 'NONE',  ( -61.56765823437498142, 10.18229166632526805, 0.7511620957034663704 ) ) ;
#1121=CARTESIAN_POINT ( 'NONE',  ( -62.99999999999998579, 11.39583333333333393, 2.077350269189627952 ) ) ;
#1123=CARTESIAN_POINT ( 'NONE',  ( -61.99999999999998579, 16.00000000000000000, 0.5000000000000041078 ) ) ;
#1124=CARTESIAN_POINT ( 'NONE',  ( -61.56765823437498852, 12.53645833299193413, 2.248837904296538515 ) ) ;
#1125=CARTESIAN_POINT ( 'NONE',  ( -62.43234176562499016, 8.494791666325268054, 2.248837904296538071 ) ) ;
#1127=ORIENTED_EDGE ( 'NONE', *, *, #1789, .T. ) ;
#1129=CARTESIAN_POINT ( 'NONE',  ( -61.99999999999999289, 9.953124999658601979, 0.5015494609379544944 ) ) ;
#1131=CARTESIAN_POINT ( 'NONE',  ( -62.86468353124998032, 15.18229166632526805, 1.000774730468978246 ) ) ;
#1132=CARTESIAN_POINT ( 'NONE',  ( -61.99999999999998579, 14.15624999931720218, 2.654700538379254571 ) ) ;
#1137=ADVANCED_FACE ( 'NONE', ( #1695 ), #5069, .T. ) ;
#1138=CARTESIAN_POINT ( 'NONE',  ( -61.99999999999999289, 12.39062499965860376, 0.5015494609379544944 ) ) ;
#1139=CARTESIAN_POINT ( 'NONE',  ( -62.43234176562499016, 8.244791666325268054, 2.248837904296538071 ) ) ;
#1140=DIRECTION ( 'NONE',  ( -0.000000000000000000, -1.000000000000000000, -0.000000000000000000 ) ) ;
#1142=CARTESIAN_POINT ( 'NONE',  ( -60.99999999999998579, 12.52083333333333215, 0.9226497308103762673 ) ) ;
#1143=CARTESIAN_POINT ( 'NONE',  ( -62.99999999999998579, 10.14583333333333570, 2.077350269189627952 ) ) ;
#1144=CARTESIAN_POINT ( 'NONE',  ( -61.56765823437498142, 14.68229166632526805, 0.7511620957034663704 ) ) ;
#1147=CARTESIAN_POINT ( 'NONE',  ( -61.99999999999998579, 10.53124999931720396, 0.3452994616207497591 ) ) ;
#1151=CARTESIAN_POINT ( 'NONE',  ( -62.86468353124998032, 11.68229166632526805, 1.000774730468978246 ) ) ;
#1155=CARTESIAN_POINT ( 'NONE',  ( -62.86468353124999453, 10.01562499965860198, 1.500000000000002220 ) ) ;
#1156=CARTESIAN_POINT ( 'NONE',  ( -61.99999999999998579, 14.31250000000000000, 0.5000000000000013323 ) ) ;
#1157=CARTESIAN_POINT ( 'NONE',  ( -61.56765823437498142, 14.93229166632526805, 0.7511620957034663704 ) ) ;
#1158=CARTESIAN_POINT ( 'NONE',  ( -60.99999999999998579, 8.989583332650536107, 0.9226497308103762673 ) ) ;
#1159=VERTEX_POINT ( 'NONE', #754 ) ;
#1160=DIRECTION ( 'NONE',  ( -0.000000000000000000, -1.000000000000000000, -0.000000000000000000 ) ) ;
#1161=( BOUNDED_CURVE ( )  B_SPLINE_CURVE ( 2, ( #5127, #7756, #2642, #10771, #5968, #910, #4240, #3161, #7702 ),
 .UNSPECIFIED., .F., .T. ) 
 B_SPLINE_CURVE_WITH_KNOTS ( ( 3, 2, 2, 2, 3 ),
 ( 0.6015625000000000000, 0.6041666666666666297, 0.6093750000000000000, 0.6145833333333333703, 0.6171875000000000000 ),
 .UNSPECIFIED. ) 
 CURVE ( )  GEOMETRIC_REPRESENTATION_ITEM ( )  RATIONAL_B_SPLINE_CURVE ( ( 0.9330127018922194093, 0.9330127018922194093, 1.000000000000000000, 0.8660254037844387076, 1.000000000000000000, 0.8660254037844387076, 1.000000000000000000, 0.9330127018922194093, 0.9330127018922194093 ) ) 
 REPRESENTATION_ITEM ( '' )  );
#1164=CARTESIAN_POINT ( 'NONE',  ( -62.49999999999998579, 9.083333333333333925, 0.6339745962155627357 ) ) ;
#1166=EDGE_CURVE ( 'NONE', #6004, #424, #5332, .T. ) ;
#1167=FACE_OUTER_BOUND ( 'NONE', #6254, .T. ) ;
#1168=CARTESIAN_POINT ( 'NONE',  ( -61.99999999999999289, 14.57812499965860198, 2.498450539062049724 ) ) ;
#1169=CARTESIAN_POINT ( 'NONE',  ( -61.56765823437498852, 10.03645833299193413, 2.248837904296538515 ) ) ;
#1171=CARTESIAN_POINT ( 'NONE',  ( -60.99999999999998579, 11.96874999931720218, 1.500000000000002220 ) ) ;
#1173=CARTESIAN_POINT ( 'NONE',  ( -62.43234176562498305, 10.97395833299193590, 0.7511620957034662593 ) ) ;
#1174=CARTESIAN_POINT ( 'NONE',  ( -62.26794919243111082, 13.57366454968463110, 0.5000000000000013323 ) ) ;
#1176=CARTESIAN_POINT ( 'NONE',  ( -61.73205080756886076, 14.02008544963257286, 0.5000000000000014433 ) ) ;
#1178=CARTESIAN_POINT ( 'NONE',  ( -61.99999999999998579, 13.15624999931720218, 2.500000000000002665 ) ) ;
#1180=CARTESIAN_POINT ( 'NONE',  ( -61.99999999999998579, 16.00000000000000000, 0.5000000000000041078 ) ) ;
#1181=CARTESIAN_POINT ( 'NONE',  ( -61.99999999999998579, 13.14062499965860198, 0.5015494609379544944 ) ) ;
#1182=CARTESIAN_POINT ( 'NONE',  ( -61.13531646874997705, 8.557291666325268054, 1.999225269531026417 ) ) ;
#1183=LINE ( 'NONE', #2138, #284 ) ;
#1185=CARTESIAN_POINT ( 'NONE',  ( -61.99999999999998579, 15.93750000000000000, 2.654700538379254571 ) ) ;
#1186=CARTESIAN_POINT ( 'NONE',  ( -62.86468353124999453, 9.786458332991934128, 1.999225269531025750 ) ) ;
#1187=CARTESIAN_POINT ( 'NONE',  ( -61.99999999999998579, 15.39062499965860198, 0.5015494609379544944 ) ) ;
#1188=CARTESIAN_POINT ( 'NONE',  ( -62.49999999999998579, 14.38541666598387003, 2.366025403784441483 ) ) ;
#1189=CARTESIAN_POINT ( 'NONE',  ( -61.99999999999998579, 14.65624999931719863, 2.500000000000002665 ) ) ;
#1191=FACE_OUTER_BOUND ( 'NONE', #4245, .T. ) ;
#1192=EDGE_LOOP ( 'NONE', ( #4332, #9103, #1729, #5757 ) ) ;
#1193=CARTESIAN_POINT ( 'NONE',  ( -61.13531646874997705, 12.30729166632526628, 1.999225269531026417 ) ) ;
#1194=CARTESIAN_POINT ( 'NONE',  ( -62.86468353124998032, 8.182291666325269830, 1.000774730468978246 ) ) ;
#1196=CARTESIAN_POINT ( 'NONE',  ( -61.99999999999998579, 15.15624999931720218, 2.500000000000002665 ) ) ;
#1197=ORIENTED_EDGE ( 'NONE', *, *, #1892, .T. ) ;
#1198=CARTESIAN_POINT ( 'NONE',  ( -62.99999999999998579, 12.60416666666666607, 0.9226497308103756012 ) ) ;
#1199=CARTESIAN_POINT ( 'NONE',  ( -61.99999999999998579, 10.06250000000000000, 0.5000000000000013323 ) ) ;
#1200=CARTESIAN_POINT ( 'NONE',  ( -61.13531646874998415, 13.66145833299193590, 1.000774730468978468 ) ) ;
#1202=CARTESIAN_POINT ( 'NONE',  ( -61.99999999999998579, 16.00000000000000000, 2.500000000000000444 ) ) ;
#1203=CARTESIAN_POINT ( 'NONE',  ( -60.99999999999998579, 10.21874999931720218, 1.500000000000002220 ) ) ;
#1204=EDGE_CURVE ( 'NONE', #6502, #5311, #805, .T. ) ;
#1207=DIRECTION ( 'NONE',  ( -0.000000000000000000, -1.000000000000000000, -0.000000000000000000 ) ) ;
#1209=CARTESIAN_POINT ( 'NONE',  ( -61.13531646874998415, 12.80729166632526805, 1.999225269531026417 ) ) ;
#1212=CARTESIAN_POINT ( 'NONE',  ( -61.99999999999998579, 10.45312499965860198, 0.5015494609379544944 ) ) ;
#1213=CARTESIAN_POINT ( 'NONE',  ( -62.49999999999998579, 15.55208333265053611, 0.6339745962155627357 ) ) ;
#1215=CARTESIAN_POINT ( 'NONE',  ( -61.13531646874998415, 13.89062499965860198, 1.500000000000002220 ) ) ;
#1216=CARTESIAN_POINT ( 'NONE',  ( -61.99999999999998579, 16.00000000000000000, 0.5000000000000041078 ) ) ;
#1217=EDGE_LOOP ( 'NONE', ( #6853, #818, #9578, #559 ) ) ;
#1221=VECTOR ( 'NONE', #1539, 1000.000000000000000 ) ;
#1224=CARTESIAN_POINT ( 'NONE',  ( -60.99999999999998579, 8.770833333333333925, 0.9226497308103762673 ) ) ;
#1225=CARTESIAN_POINT ( 'NONE',  ( -62.99999999999998579, 9.593749999317202182, 1.500000000000001998 ) ) ;
#1228=CARTESIAN_POINT ( 'NONE',  ( -61.13531646874997705, 14.86979166632526805, 1.999225269531026417 ) ) ;
#1229=CARTESIAN_POINT ( 'NONE',  ( -61.13531646874998415, 9.578124999658600203, 1.500000000000002220 ) ) ;
#1231=CARTESIAN_POINT ( 'NONE',  ( -62.43234176562499016, 11.05729166632526805, 2.248837904296538071 ) ) ;
#1233=CARTESIAN_POINT ( 'NONE',  ( -62.99999999999998579, 13.62500000000000000, 1.500000000000001998 ) ) ;
#1235=( BOUNDED_CURVE ( )  B_SPLINE_CURVE ( 2, ( #2228, #3944, #10497, #7288, #1225, #10608, #2896, #394, #2117 ),
 .UNSPECIFIED., .F., .T. ) 
 B_SPLINE_CURVE_WITH_KNOTS ( ( 3, 2, 2, 2, 3 ),
 ( 0.1640624999999999722, 0.1666666666666666574, 0.1718750000000000000, 0.1770833333333333426, 0.1796875000000000555 ),
 .UNSPECIFIED. ) 
 CURVE ( )  GEOMETRIC_REPRESENTATION_ITEM ( )  RATIONAL_B_SPLINE_CURVE ( ( 0.9330127018922194093, 0.9330127018922186322, 1.000000000000000000, 0.8660254037844387076, 1.000000000000000000, 0.8660254037844387076, 1.000000000000000000, 0.9330127018922178550, 0.9330127018922192983 ) ) 
 REPRESENTATION_ITEM ( '' )  );
#1237=CARTESIAN_POINT ( 'NONE',  ( -62.49999999999998579, 9.083333333333333925, 0.6339745962155627357 ) ) ;
#1239=VERTEX_POINT ( 'NONE', #129 ) ;
#1240=CARTESIAN_POINT ( 'NONE',  ( -61.99999999999998579, 10.15624999931720041, 2.500000000000002665 ) ) ;
#1241=CARTESIAN_POINT ( 'NONE',  ( -61.99999999999998579, 12.89062499965860376, 0.5015494609379544944 ) ) ;
#1242=CARTESIAN_POINT ( 'NONE',  ( -61.13531646874997705, 10.05729166632526983, 1.999225269531026417 ) ) ;
#1245=VERTEX_POINT ( 'NONE', #1074 ) ;
#1246=CARTESIAN_POINT ( 'NONE',  ( -61.99999999999998579, 14.06250000000000000, 0.5000000000000013323 ) ) ;
#1247=CARTESIAN_POINT ( 'NONE',  ( -62.43234176562499016, 12.05729166632526628, 2.248837904296538071 ) ) ;
#1249=CARTESIAN_POINT ( 'NONE',  ( -61.99999999999998579, 15.76562499965860020, 2.498450539062049724 ) ) ;
#1251=CARTESIAN_POINT ( 'NONE',  ( -61.49999999999998579, 15.01041666598386826, 0.6339745962155628467 ) ) ;
#1254=CARTESIAN_POINT ( 'NONE',  ( -61.99999999999998579, 15.28124999931720218, 0.5000000000000013323 ) ) ;
#1257=CARTESIAN_POINT ( 'NONE',  ( -61.13531646874997705, 12.84895833299193413, 1.000774730468978468 ) ) ;
#1258=CARTESIAN_POINT ( 'NONE',  ( -62.43234176562498305, 8.661458332991934128, 0.7511620957034662593 ) ) ;
#1259=DIRECTION ( 'NONE',  ( -0.000000000000000000, -1.000000000000000000, -0.000000000000000000 ) ) ;
#1260=VERTEX_POINT ( 'NONE', #3461 ) ;
#1261=CARTESIAN_POINT ( 'NONE',  ( -62.99999999999998579, 11.89583333333333215, 2.077350269189627952 ) ) ;
#1263=CARTESIAN_POINT ( 'NONE',  ( -61.49999999999998579, 15.92708333265053433, 2.366025403784441927 ) ) ;
#1264=CARTESIAN_POINT ( 'NONE',  ( -62.43234176562499016, 14.05729166632526805, 2.248837904296538071 ) ) ;
#1266=CARTESIAN_POINT ( 'NONE',  ( -62.99999999999998579, 14.32291666598387003, 0.9226497308103756012 ) ) ;
#1267=CARTESIAN_POINT ( 'NONE',  ( -60.99999999999998579, 9.947916665983868256, 2.077350269189628840 ) ) ;
#1268=VERTEX_POINT ( 'NONE', #904 ) ;
#1269=CARTESIAN_POINT ( 'NONE',  ( -61.99999999999998579, 15.40624999931720218, 2.500000000000002665 ) ) ;
#1270=CARTESIAN_POINT ( 'NONE',  ( -61.56765823437498852, 12.28645833299193413, 2.248837904296538515 ) ) ;
#1272=ADVANCED_FACE ( 'NONE', ( #8756 ), #189, .T. ) ;
#1274=CARTESIAN_POINT ( 'NONE',  ( -61.13531646874998415, 10.16145833299193413, 1.000774730468978468 ) ) ;
#1276=CARTESIAN_POINT ( 'NONE',  ( -61.13531646874998415, 15.89062499965860198, 1.500000000000002220 ) ) ;
#1277=CARTESIAN_POINT ( 'NONE',  ( -61.99999999999998579, 26.00000000000000355, 4.000000000000004441 ) ) ;
#1278=EDGE_LOOP ( 'NONE', ( #2312, #1859, #4529, #3092 ) ) ;
#1279=FACE_OUTER_BOUND ( 'NONE', #6316, .T. ) ;
#1281=EDGE_CURVE ( 'NONE', #10876, #5522, #9466, .T. ) ;
#1283=CARTESIAN_POINT ( 'NONE',  ( -62.49999999999998579, 15.13541666598387003, 2.366025403784441483 ) ) ;
#1284=CARTESIAN_POINT ( 'NONE',  ( -62.49999999999998579, 10.08333333333333215, 0.6339745962155627357 ) ) ;
#1287=CARTESIAN_POINT ( 'NONE',  ( -60.99999999999998579, 10.71874999931720396, 1.500000000000002220 ) ) ;
#1289=CARTESIAN_POINT ( 'NONE',  ( -61.13531646874998415, 10.05729166632526983, 1.999225269531026417 ) ) ;
#1290=CARTESIAN_POINT ( 'NONE',  ( -61.99999999999998579, 16.00000000000000000, 2.500000000000000444 ) ) ;
#1292=AXIS2_PLACEMENT_3D ( 'NONE', #7583, #3406, #9982 ) ;
#1293=CARTESIAN_POINT ( 'NONE',  ( -62.86468353124998032, 10.24479166632526983, 1.000774730468978246 ) ) ;
#1294=DIRECTION ( 'NONE',  ( 0.000000000000000000, 0.000000000000000000, 1.000000000000000000 ) ) ;
#1298=PRODUCT_DEFINITION_CONTEXT ( 'detailed design', #6771, 'design' ) ;
#1299=CARTESIAN_POINT ( 'NONE',  ( -61.99999999999998579, 16.00000000000000000, 2.500000000000000444 ) ) ;
#1300=ORIENTED_EDGE ( 'NONE', *, *, #4359, .T. ) ;
#1301=CARTESIAN_POINT ( 'NONE',  ( -60.99999999999998579, 10.21874999931720218, 1.500000000000002220 ) ) ;
#1302=CARTESIAN_POINT ( 'NONE',  ( -62.86468353124999453, 12.95312499965860198, 1.500000000000002220 ) ) ;
#1303=CARTESIAN_POINT ( 'NONE',  ( -61.13531646874997705, 10.09895833299193413, 1.000774730468978468 ) ) ;
#1304=PLANE ( 'NONE',  #10493 ) ;
#1305=ORIENTED_EDGE ( 'NONE', *, *, #1734, .F. ) ;
#1307=CARTESIAN_POINT ( 'NONE',  ( -62.43234176562499016, 10.80729166632526805, 2.248837904296538071 ) ) ;
#1308=ADVANCED_FACE ( 'NONE', ( #7920 ), #301, .T. ) ;
#1310=CARTESIAN_POINT ( 'NONE',  ( -61.56765823437498852, 15.03645833299193590, 2.248837904296538515 ) ) ;
#1311=CARTESIAN_POINT ( 'NONE',  ( -61.99999999999998579, 14.40624999931720218, 2.654700538379254571 ) ) ;
#1315=CARTESIAN_POINT ( 'NONE',  ( -61.99999999999998579, 13.53124999931720041, 0.5000000000000013323 ) ) ;
#1316=EDGE_LOOP ( 'NONE', ( #2338, #10742, #637, #5601 ) ) ;
#1318=CARTESIAN_POINT ( 'NONE',  ( -61.56765823437498142, 13.11979166632526805, 0.7511620957034663704 ) ) ;
#1319=CARTESIAN_POINT ( 'NONE',  ( -61.99999999999998579, 8.640624999658601979, 0.5015494609379544944 ) ) ;
#1323=CARTESIAN_POINT ( 'NONE',  ( -60.99999999999998579, 12.27083333333333393, 0.9226497308103762673 ) ) ;
#1325=CARTESIAN_POINT ( 'NONE',  ( -62.26794919243111082, 13.39508544963257286, 2.500000000000003109 ) ) ;
#1326=EDGE_CURVE ( 'NONE', #869, #5526, #7085, .T. ) ;
#1329=CARTESIAN_POINT ( 'NONE',  ( -61.99999999999998579, 10.03124999931720396, 0.3452994616207497591 ) ) ;
#1330=VERTEX_POINT ( 'NONE', #1315 ) ;
#1331=DIRECTION ( 'NONE',  ( 0.000000000000000000, 0.000000000000000000, 1.000000000000000000 ) ) ;
#1333=CARTESIAN_POINT ( 'NONE',  ( -62.86468353124999453, 12.70312499965860198, 1.500000000000002220 ) ) ;
#1336=CARTESIAN_POINT ( 'NONE',  ( -61.56765823437498852, 11.34895833299193590, 2.248837904296538515 ) ) ;
#1337=CARTESIAN_POINT ( 'NONE',  ( -61.99999999999998579, 13.03124999931720218, 0.5000000000000013323 ) ) ;
#1338=CARTESIAN_POINT ( 'NONE',  ( -61.56765823437498142, 15.68229166632526628, 0.7511620957034663704 ) ) ;
#1339=CARTESIAN_POINT ( 'NONE',  ( -61.99999999999998579, 9.031249999317202182, 0.5000000000000013323 ) ) ;
#1342=ORIENTED_EDGE ( 'NONE', *, *, #7597, .T. ) ;
#1343=DIRECTION ( 'NONE',  ( -0.000000000000000000, -1.000000000000000000, -0.000000000000000000 ) ) ;
#1344=CARTESIAN_POINT ( 'NONE',  ( -62.99999999999998579, 9.645833333333332149, 2.077350269189627952 ) ) ;
#1346=CARTESIAN_POINT ( 'NONE',  ( -61.99999999999998579, 10.28124999931720218, 0.5000000000000013323 ) ) ;
#1347=CARTESIAN_POINT ( 'NONE',  ( -60.99999999999998579, 8.270833333333333925, 0.9226497308103762673 ) ) ;
#1348=EDGE_CURVE ( 'NONE', #4452, #8833, #3865, .T. ) ;
#1349=CARTESIAN_POINT ( 'NONE',  ( -61.13531646874998415, 10.55729166632526805, 1.999225269531026417 ) ) ;
#1351=CARTESIAN_POINT ( 'NONE',  ( -62.43234176562499016, 12.30729166632526805, 2.248837904296538071 ) ) ;
#1352=EDGE_CURVE ( 'NONE', #2202, #2668, #7554, .T. ) ;
#1353=DIRECTION ( 'NONE',  ( 0.000000000000000000, 1.000000000000000000, 0.000000000000000000 ) ) ;
#1358=CARTESIAN_POINT ( 'NONE',  ( -62.99999999999998579, 10.09374999931720218, 1.500000000000001998 ) ) ;
#1359=CARTESIAN_POINT ( 'NONE',  ( -62.43234176562498305, 13.66145833299193413, 0.7511620957034662593 ) ) ;
#1360=CARTESIAN_POINT ( 'NONE',  ( -62.86468353124999453, 10.47395833299193235, 1.999225269531025750 ) ) ;
#1363=CARTESIAN_POINT ( 'NONE',  ( -61.99999999999998579, 11.43750000000000000, 2.500000000000002665 ) ) ;
#1364=CARTESIAN_POINT ( 'NONE',  ( -62.86468353124998032, 10.74479166632526805, 1.000774730468978024 ) ) ;
#1365=CARTESIAN_POINT ( 'NONE',  ( -62.99999999999998579, 15.14583333333333215, 2.077350269189627952 ) ) ;
#1366=CARTESIAN_POINT ( 'NONE',  ( -62.49999999999998579, 16.05208333265053255, 0.6339745962155627357 ) ) ;
#1367=CARTESIAN_POINT ( 'NONE',  ( -61.99999999999998579, 14.78124999931720218, 0.5000000000000013323 ) ) ;
#1371=EDGE_CURVE ( 'NONE', #2202, #3478, #5006, .T. ) ;
#1372=CARTESIAN_POINT ( 'NONE',  ( -62.86468353124998032, 12.93229166632526805, 1.000774730468978024 ) ) ;
#1373=CARTESIAN_POINT ( 'NONE',  ( -61.99999999999998579, 10.26562499965860376, 2.498450539062049724 ) ) ;
#1375=CARTESIAN_POINT ( 'NONE',  ( -61.49999999999998579, 13.04166666666666607, 0.6339745962155628467 ) ) ;
#1377=CARTESIAN_POINT ( 'NONE',  ( -62.99999999999998579, 11.07291666598386826, 0.9226497308103756012 ) ) ;
#1378=CARTESIAN_POINT ( 'NONE',  ( -61.99999999999998579, 13.43749999999999822, 2.500000000000002665 ) ) ;
#1379=CARTESIAN_POINT ( 'NONE',  ( -62.43234176562499016, 12.99479166632526805, 2.248837904296538071 ) ) ;
#1381=EDGE_LOOP ( 'NONE', ( #2924, #6869, #5450, #5185 ) ) ;
#1382=CARTESIAN_POINT ( 'NONE',  ( -61.56765823437498142, 10.93229166632526805, 0.7511620957034663704 ) ) ;
#1384=EDGE_CURVE ( 'NONE', #8873, #9906, #9440, .T. ) ;
#1386=CARTESIAN_POINT ( 'NONE',  ( -61.99999999999998579, 15.57812499965860198, 2.498450539062049724 ) ) ;
#1389=VECTOR ( 'NONE', #1722, 1000.000000000000000 ) ;
#1390=ORIENTED_EDGE ( 'NONE', *, *, #8995, .F. ) ;
#1392=CARTESIAN_POINT ( 'NONE',  ( -62.99999999999998579, 9.395833333333333925, 2.077350269189627952 ) ) ;
#1393=CARTESIAN_POINT ( 'NONE',  ( -61.49999999999998579, 11.29166666666666607, 0.6339745962155628467 ) ) ;
#1394=DIRECTION ( 'NONE',  ( 0.000000000000000000, 0.000000000000000000, -1.000000000000000000 ) ) ;
#1395=CARTESIAN_POINT ( 'NONE',  ( -62.49999999999998579, 14.80208333265053611, 0.6339745962155627357 ) ) ;
#1396=( BOUNDED_CURVE ( )  B_SPLINE_CURVE ( 2, ( #7764, #145, #6149, #10482, #6326, #9655, #261, #3644, #1269 ),
 .UNSPECIFIED., .F., .T. ) 
 B_SPLINE_CURVE_WITH_KNOTS ( ( 3, 2, 2, 2, 3 ),
 ( 0.8828125000000000000, 0.8854166666666666297, 0.8906250000000000000, 0.8958333333333333703, 0.8984375000000000000 ),
 .UNSPECIFIED. ) 
 CURVE ( )  GEOMETRIC_REPRESENTATION_ITEM ( )  RATIONAL_B_SPLINE_CURVE ( ( 0.9330127018922194093, 0.9330127018922194093, 1.000000000000000000, 0.8660254037844387076, 1.000000000000000000, 0.8660254037844387076, 1.000000000000000000, 0.9330127018922194093, 0.9330127018922194093 ) ) 
 REPRESENTATION_ITEM ( '' )  );
#1397=CARTESIAN_POINT ( 'NONE',  ( -62.99999999999998579, 8.364583332650536107, 2.077350269189627952 ) ) ;
#1399=CARTESIAN_POINT ( 'NONE',  ( -61.56765823437498142, 11.43229166632526805, 0.7511620957034663704 ) ) ;
#1402=CARTESIAN_POINT ( 'NONE',  ( -61.73205080756886076, 9.270085449632572860, 0.5000000000000014433 ) ) ;
#1403=DIRECTION ( 'NONE',  ( 0.000000000000000000, 0.000000000000000000, -1.000000000000000000 ) ) ;
#1406=CARTESIAN_POINT ( 'NONE',  ( -61.73205080756886076, 14.16741454900183328, 2.500000000000003109 ) ) ;
#1407=CARTESIAN_POINT ( 'NONE',  ( -61.13531646874998415, 14.30729166632526983, 1.999225269531026417 ) ) ;
#1409=CARTESIAN_POINT ( 'NONE',  ( -62.43234176562499016, 10.49479166632526983, 2.248837904296538071 ) ) ;
#1413=CARTESIAN_POINT ( 'NONE',  ( -62.86468353124999453, 11.03645833299193590, 1.999225269531025750 ) ) ;
#1416=CARTESIAN_POINT ( 'NONE',  ( -60.99999999999998579, 15.73958333265053611, 0.9226497308103762673 ) ) ;
#1422=CARTESIAN_POINT ( 'NONE',  ( -62.43234176562498305, 14.16145833299193413, 0.7511620957034662593 ) ) ;
#1423=CARTESIAN_POINT ( 'NONE',  ( -61.56765823437498142, 10.11979166632526805, 0.7511620957034663704 ) ) ;
#1424=CARTESIAN_POINT ( 'NONE',  ( -60.99999999999998579, 16.10937499965860198, 1.500000000000002220 ) ) ;
#1426=CARTESIAN_POINT ( 'NONE',  ( -61.49999999999998579, 14.29166666666666785, 0.6339745962155628467 ) ) ;
#1430=CARTESIAN_POINT ( 'NONE',  ( -62.49999999999998579, 11.63541666598387003, 2.366025403784441483 ) ) ;
#1433=CARTESIAN_POINT ( 'NONE',  ( -62.99999999999998579, 14.89583333333333925, 2.077350269189627952 ) ) ;
#1434=AXIS2_PLACEMENT_3D ( 'NONE', #8540, #1762, #10194 ) ;
#1435=CARTESIAN_POINT ( 'NONE',  ( -61.13531646874998415, 12.55729166632526805, 1.999225269531026417 ) ) ;
#1437=CARTESIAN_POINT ( 'NONE',  ( -62.43234176562498305, 11.97395833299193413, 0.7511620957034662593 ) ) ;
#1439=CARTESIAN_POINT ( 'NONE',  ( -61.99999999999998579, 15.95312499965860198, 0.5015494609379544944 ) ) ;
#1443=CARTESIAN_POINT ( 'NONE',  ( -61.49999999999998579, 8.760416665983868256, 0.6339745962155628467 ) ) ;
#1444=CARTESIAN_POINT ( 'NONE',  ( -61.49999999999998579, 9.291666666666666075, 0.6339745962155628467 ) ) ;
#1446=FACE_OUTER_BOUND ( 'NONE', #6334, .T. ) ;
#1448=EDGE_CURVE ( 'NONE', #8888, #10687, #4798, .T. ) ;
#1449=CARTESIAN_POINT ( 'NONE',  ( -62.99999999999998579, 8.343749999317202182, 1.500000000000001998 ) ) ;
#1450=CARTESIAN_POINT ( 'NONE',  ( -62.86468353124998742, 12.03645833299193413, 1.999225269531025972 ) ) ;
#1455=DIRECTION ( 'NONE',  ( -0.000000000000000000, -1.000000000000000000, -0.000000000000000000 ) ) ;
#1460=CARTESIAN_POINT ( 'NONE',  ( -62.43234176562498305, 14.16145833299193413, 0.7511620957034662593 ) ) ;
#1461=CARTESIAN_POINT ( 'NONE',  ( -61.99999999999999289, 10.26562499965860376, 2.498450539062049724 ) ) ;
#1463=( BOUNDED_CURVE ( )  B_SPLINE_CURVE ( 2, ( #9631, #3856, #2025, #4682, #418, #7137, #3741, #7856, #10519 ),
 .UNSPECIFIED., .F., .F. ) 
 B_SPLINE_CURVE_WITH_KNOTS ( ( 3, 2, 2, 2, 3 ),
 ( 0.02343749999999996531, 0.02604166666666666782, 0.03125000000000000000, 0.03645833333333333565, 0.03906250000000003469 ),
 .UNSPECIFIED. ) 
 CURVE ( )  GEOMETRIC_REPRESENTATION_ITEM ( )  RATIONAL_B_SPLINE_CURVE ( ( 0.9330127018922194093, 0.9330127018922185211, 1.000000000000000000, 0.8660254037844387076, 1.000000000000000000, 0.8660254037844387076, 1.000000000000000000, 0.9330127018922185211, 0.9330127018922194093 ) ) 
 REPRESENTATION_ITEM ( '' )  );
#1464=CARTESIAN_POINT ( 'NONE',  ( -61.99999999999998579, 8.281249999317202182, 0.5000000000000013323 ) ) ;
#1466=CARTESIAN_POINT ( 'NONE',  ( -61.56765823437498852, 11.34895833299193590, 2.248837904296538515 ) ) ;
#1467=CARTESIAN_POINT ( 'NONE',  ( -61.13531646874998415, 8.098958332991934128, 1.000774730468978468 ) ) ;
#1470=CARTESIAN_POINT ( 'NONE',  ( -61.13531646874998415, 8.390624999658601979, 1.500000000000002220 ) ) ;
#1471=DIRECTION ( 'NONE',  ( 0.000000000000000000, 0.000000000000000000, -1.000000000000000000 ) ) ;
#1475=CARTESIAN_POINT ( 'NONE',  ( -62.86468353124998032, 13.93229166632526805, 1.000774730468978024 ) ) ;
#1476=CARTESIAN_POINT ( 'NONE',  ( -61.56765823437498142, 9.369791666325268054, 0.7511620957034663704 ) ) ;
#1477=CARTESIAN_POINT ( 'NONE',  ( -61.99999999999998579, 10.43750000000000000, 2.500000000000002665 ) ) ;
#1479=CARTESIAN_POINT ( 'NONE',  ( -62.49999999999998579, 14.33333333333333393, 0.6339745962155627357 ) ) ;
#1483=ADVANCED_FACE ( 'NONE', ( #1191 ), #4634, .T. ) ;
#1484=CARTESIAN_POINT ( 'NONE',  ( -61.99999999999998579, 12.40624999931720218, 2.654700538379254571 ) ) ;
#1487=CARTESIAN_POINT ( 'NONE',  ( -62.86468353124998032, 14.43229166632526805, 1.000774730468978246 ) ) ;
#1488=ORIENTED_EDGE ( 'NONE', *, *, #6990, .F. ) ;
#1489=CARTESIAN_POINT ( 'NONE',  ( -61.99999999999998579, 10.95312499965860020, 0.5015494609379544944 ) ) ;
#1491=VECTOR ( 'NONE', #1699, 1000.000000000000000 ) ;
#1492=CARTESIAN_POINT ( 'NONE',  ( -61.56765823437498852, 15.59895833299193590, 2.248837904296538515 ) ) ;
#1493=ORIENTED_EDGE ( 'NONE', *, *, #9866, .F. ) ;
#1496=ORIENTED_EDGE ( 'NONE', *, *, #3408, .F. ) ;
#1498=CARTESIAN_POINT ( 'NONE',  ( -60.99999999999998579, 9.229166666666667851, 2.077350269189628840 ) ) ;
#1502=DIRECTION ( 'NONE',  ( -0.000000000000000000, -1.000000000000000000, -0.000000000000000000 ) ) ;
#1503=CARTESIAN_POINT ( 'NONE',  ( -61.99999999999998579, 12.20312499965860198, 0.5015494609379544944 ) ) ;
#1504=CARTESIAN_POINT ( 'NONE',  ( -62.99999999999998579, 9.114583332650536107, 2.077350269189627952 ) ) ;
#1510=CARTESIAN_POINT ( 'NONE',  ( -62.43234176562499016, 13.49479166632526805, 2.248837904296538071 ) ) ;
#1512=CARTESIAN_POINT ( 'NONE',  ( -61.99999999999998579, 14.56249999999999822, 0.5000000000000013323 ) ) ;
#1513=DIRECTION ( 'NONE',  ( -0.000000000000000000, -1.000000000000000000, -0.000000000000000000 ) ) ;
#1514=CARTESIAN_POINT ( 'NONE',  ( -62.86468353124999453, 12.28645833299193413, 1.999225269531025750 ) ) ;
#1515=CARTESIAN_POINT ( 'NONE',  ( -62.86468353124998032, 15.99479166632526805, 1.000774730468978246 ) ) ;
#1518=CYLINDRICAL_SURFACE ( 'NONE', #8159, 2.500000000000002220 ) ;
#1520=CARTESIAN_POINT ( 'NONE',  ( -61.49999999999998579, 15.51041666598387003, 0.6339745962155628467 ) ) ;
#1521=DIRECTION ( 'NONE',  ( -0.000000000000000000, -1.000000000000000000, -0.000000000000000000 ) ) ;
#1523=DIRECTION ( 'NONE',  ( -0.000000000000000000, -1.000000000000000000, -0.000000000000000000 ) ) ;
#1524=CARTESIAN_POINT ( 'NONE',  ( -61.99999999999998579, 8.062500000000000000, 0.5000000000000013323 ) ) ;
#1525=( BOUNDED_CURVE ( )  B_SPLINE_CURVE ( 2, ( #7048, #8778, #9543, #4655, #8948, #1158, #8116, #447, #1339 ),
 .UNSPECIFIED., .F., .T. ) 
 B_SPLINE_CURVE_WITH_KNOTS ( ( 3, 2, 2, 2, 3 ),
 ( 0.08593750000000000000, 0.08854166666666667129, 0.09375000000000000000, 0.09895833333333332871, 0.1015624999999999722 ),
 .UNSPECIFIED. ) 
 CURVE ( )  GEOMETRIC_REPRESENTATION_ITEM ( )  RATIONAL_B_SPLINE_CURVE ( ( 0.9330127018922194093, 0.9330127018922194093, 1.000000000000000000, 0.8660254037844387076, 1.000000000000000000, 0.8660254037844387076, 1.000000000000000000, 0.9330127018922200755, 0.9330127018922194093 ) ) 
 REPRESENTATION_ITEM ( '' )  );
#1526=CARTESIAN_POINT ( 'NONE',  ( -61.13531646874997705, 14.84895833299193413, 1.000774730468978468 ) ) ;
#1527=CARTESIAN_POINT ( 'NONE',  ( -62.43234176562499016, 9.244791666325268054, 2.248837904296538071 ) ) ;
#1528=CARTESIAN_POINT ( 'NONE',  ( -62.86468353124999453, 15.78645833299193590, 1.999225269531025750 ) ) ;
#1530=CARTESIAN_POINT ( 'NONE',  ( -62.49999999999998579, 14.41666666666666785, 2.366025403784441483 ) ) ;
#1531=CARTESIAN_POINT ( 'NONE',  ( -61.99999999999998579, 13.65624999931720218, 2.500000000000002665 ) ) ;
#1532=CARTESIAN_POINT ( 'NONE',  ( -61.49999999999998579, 12.42708333265053611, 2.366025403784441927 ) ) ;
#1534=CARTESIAN_POINT ( 'NONE',  ( -62.43234176562499016, 13.49479166632526805, 2.248837904296538071 ) ) ;
#1535=CARTESIAN_POINT ( 'NONE',  ( -60.99999999999998579, 11.50000000000000000, 1.500000000000002220 ) ) ;
#1538=CARTESIAN_POINT ( 'NONE',  ( -62.86468353124998742, 11.78645833299193590, 1.999225269531025972 ) ) ;
#1539=DIRECTION ( 'NONE',  ( -0.000000000000000000, -1.000000000000000000, -0.000000000000000000 ) ) ;
#1541=ORIENTED_EDGE ( 'NONE', *, *, #7256, .T. ) ;
#1543=ORIENTED_EDGE ( 'NONE', *, *, #5697, .T. ) ;
#1544=CARTESIAN_POINT ( 'NONE',  ( -60.99999999999998579, 9.468749999317202182, 1.500000000000002220 ) ) ;
#1545=CARTESIAN_POINT ( 'NONE',  ( -61.49999999999998579, 11.45833333333333393, 2.366025403784441927 ) ) ;
#1547=CARTESIAN_POINT ( 'NONE',  ( -60.99999999999998579, 8.479166666666666075, 2.077350269189628840 ) ) ;
#1548=CARTESIAN_POINT ( 'NONE',  ( -61.49999999999998579, 12.29166666666666607, 0.6339745962155628467 ) ) ;
#1549=CARTESIAN_POINT ( 'NONE',  ( -61.99999999999998579, 8.656249999317202182, 2.654700538379254571 ) ) ;
#1551=CARTESIAN_POINT ( 'NONE',  ( -61.13531646874998415, 11.89062499965860198, 1.500000000000002220 ) ) ;
#1554=CARTESIAN_POINT ( 'NONE',  ( -61.99999999999998579, 9.156249999317203958, 2.500000000000002665 ) ) ;
#1559=CARTESIAN_POINT ( 'NONE',  ( -61.56765823437498142, 14.36979166632526983, 0.7511620957034663704 ) ) ;
#1561=CARTESIAN_POINT ( 'NONE',  ( -62.99999999999998579, 8.364583332650536107, 2.077350269189627952 ) ) ;
#1562=CARTESIAN_POINT ( 'NONE',  ( -61.13531646874998415, 12.14062499965860198, 1.500000000000002220 ) ) ;
#1564=CARTESIAN_POINT ( 'NONE',  ( -61.13531646874998415, 8.078124999658601979, 1.500000000000002220 ) ) ;
#1567=CARTESIAN_POINT ( 'NONE',  ( -62.99999999999998579, 15.36458333265053611, 2.077350269189627952 ) ) ;
#1573=CARTESIAN_POINT ( 'NONE',  ( -61.99999999999999289, 14.01562499965860376, 2.498450539062049724 ) ) ;
#1574=CARTESIAN_POINT ( 'NONE',  ( -61.13531646874998415, 10.09895833299193413, 1.000774730468978468 ) ) ;
#1575=CARTESIAN_POINT ( 'NONE',  ( -61.56765823437498852, 15.09895833299193590, 2.248837904296538515 ) ) ;
#1579=CARTESIAN_POINT ( 'NONE',  ( -61.49999999999998579, 13.20833333333333215, 2.366025403784441927 ) ) ;
#1580=CARTESIAN_POINT ( 'NONE',  ( -61.13531646874997705, 9.369791666325268054, 1.999225269531026417 ) ) ;
#1581=VECTOR ( 'NONE', #4734, 1000.000000000000000 ) ;
#1582=CARTESIAN_POINT ( 'NONE',  ( -62.99999999999998579, 12.07291666598386826, 0.9226497308103756012 ) ) ;
#1585=( BOUNDED_CURVE ( )  B_SPLINE_CURVE ( 2, ( #6236, #9729, #281, #3844, #2013, #7234, #5387, #7959, #5563 ),
 .UNSPECIFIED., .F., .F. ) 
 B_SPLINE_CURVE_WITH_KNOTS ( ( 3, 2, 2, 2, 3 ),
 ( 0.5078125000000000000, 0.5104166666666666297, 0.5156250000000000000, 0.5208333333333333703, 0.5234375000000000000 ),
 .UNSPECIFIED. ) 
 CURVE ( )  GEOMETRIC_REPRESENTATION_ITEM ( )  RATIONAL_B_SPLINE_CURVE ( ( 0.9330127018922194093, 0.9330127018922194093, 1.000000000000000000, 0.8660254037844387076, 1.000000000000000000, 0.8660254037844387076, 1.000000000000000000, 0.9330127018922194093, 0.9330127018922194093 ) ) 
 REPRESENTATION_ITEM ( '' )  );
#1586=CARTESIAN_POINT ( 'NONE',  ( -61.99999999999998579, 14.14062499965860020, 0.5015494609379544944 ) ) ;
#1592=CARTESIAN_POINT ( 'NONE',  ( -61.56765823437498852, 12.59895833299193413, 2.248837904296538515 ) ) ;
#1593=CARTESIAN_POINT ( 'NONE',  ( -61.99999999999998579, 16.00000000000000000, 1.500000000000002220 ) ) ;
#1601=CARTESIAN_POINT ( 'NONE',  ( -62.99999999999998579, 11.14583333333333393, 2.077350269189627952 ) ) ;
#1603=CARTESIAN_POINT ( 'NONE',  ( -61.49999999999998579, 8.458333333333333925, 2.366025403784441927 ) ) ;
#1604=CARTESIAN_POINT ( 'NONE',  ( -62.99999999999998579, 15.89583333333333215, 2.077350269189627952 ) ) ;
#1606=CARTESIAN_POINT ( 'NONE',  ( -62.43234176562498305, 12.97395833299193590, 0.7511620957034662593 ) ) ;
#1607=CARTESIAN_POINT ( 'NONE',  ( -62.99999999999998579, 9.072916665983868256, 0.9226497308103756012 ) ) ;
#1608=VERTEX_POINT ( 'NONE', #5742 ) ;
#1611=( BOUNDED_CURVE ( )  B_SPLINE_CURVE ( 2, ( #9651, #9237, #4999, #7208, #10058, #2212, #4164, #1621, #6635 ),
 .UNSPECIFIED., .F., .F. ) 
 B_SPLINE_CURVE_WITH_KNOTS ( ( 3, 2, 2, 2, 3 ),
 ( 0.8671875000000000000, 0.8697916666666666297, 0.8750000000000000000, 0.8802083333333333703, 0.8828125000000000000 ),
 .UNSPECIFIED. ) 
 CURVE ( )  GEOMETRIC_REPRESENTATION_ITEM ( )  RATIONAL_B_SPLINE_CURVE ( ( 0.9330127018922194093, 0.9330127018922194093, 1.000000000000000000, 0.8660254037844387076, 1.000000000000000000, 0.8660254037844387076, 1.000000000000000000, 0.9330127018922194093, 0.9330127018922194093 ) ) 
 REPRESENTATION_ITEM ( '' )  );
#1614=EDGE_CURVE ( 'NONE', #3158, #10494, #1941, .T. ) ;
#1615=CARTESIAN_POINT ( 'NONE',  ( -61.13531646874998415, 14.59895833299193590, 1.000774730468978468 ) ) ;
#1617=DIRECTION ( 'NONE',  ( -0.000000000000000000, -1.000000000000000000, -0.000000000000000000 ) ) ;
#1618=CARTESIAN_POINT ( 'NONE',  ( -62.43234176562499016, 12.55729166632526805, 2.248837904296538071 ) ) ;
#1619=CARTESIAN_POINT ( 'NONE',  ( -62.43234176562498305, 15.22395833299193590, 0.7511620957034662593 ) ) ;
#1621=CARTESIAN_POINT ( 'NONE',  ( -61.73205080756886076, 15.05133545031537068, 0.5000000000000014433 ) ) ;
#1624=CARTESIAN_POINT ( 'NONE',  ( -61.13531646874998415, 8.640624999658601979, 1.500000000000002220 ) ) ;
#1626=EDGE_LOOP ( 'NONE', ( #5551, #6407, #1989, #2000 ) ) ;
#1628=CARTESIAN_POINT ( 'NONE',  ( -60.99999999999998579, 8.000000000000000000, 1.500000000000002220 ) ) ;
#1630=CARTESIAN_POINT ( 'NONE',  ( -62.43234176562498305, 14.66145833299193413, 0.7511620957034662593 ) ) ;
#1632=CARTESIAN_POINT ( 'NONE',  ( -61.13531646874998415, 11.57812499965860198, 1.500000000000002220 ) ) ;
#1633=CARTESIAN_POINT ( 'NONE',  ( -62.86468353124999453, 8.203124999658601979, 1.500000000000002220 ) ) ;
#1636=CARTESIAN_POINT ( 'NONE',  ( -62.49999999999998579, 13.91666666666666785, 2.366025403784441483 ) ) ;
#1637=CARTESIAN_POINT ( 'NONE',  ( -61.13531646874998415, 8.890624999658601979, 1.500000000000002220 ) ) ;
#1638=( LENGTH_UNIT ( ) NAMED_UNIT ( * ) SI_UNIT ( .MILLI., .METRE. ) );
#1639=CARTESIAN_POINT ( 'NONE',  ( -62.49999999999998579, 12.55208333265053611, 0.6339745962155627357 ) ) ;
#1645=CARTESIAN_POINT ( 'NONE',  ( -61.13531646874998415, 13.55729166632526805, 1.999225269531026417 ) ) ;
#1647=EDGE_CURVE ( 'NONE', #10509, #1800, #87, .T. ) ;
#1649=AXIS2_PLACEMENT_3D ( 'NONE', #791, #6592, #7472 ) ;
#1651=CARTESIAN_POINT ( 'NONE',  ( -62.86468353124999453, 13.51562499965860020, 1.500000000000002220 ) ) ;
#1653=ADVANCED_FACE ( 'NONE', ( #2736 ), #8678, .T. ) ;
#1655=ORIENTED_EDGE ( 'NONE', *, *, #8885, .T. ) ;
#1659=CARTESIAN_POINT ( 'NONE',  ( -60.99999999999998579, 11.25000000000000000, 1.500000000000002220 ) ) ;
#1661=EDGE_LOOP ( 'NONE', ( #7893, #2024, #4379, #10621 ) ) ;
#1662=CARTESIAN_POINT ( 'NONE',  ( -62.86468353124999453, 9.515624999658600203, 1.500000000000002220 ) ) ;
#1665=CARTESIAN_POINT ( 'NONE',  ( -62.43234176562499016, 13.30729166632526805, 2.248837904296538071 ) ) ;
#1666=CARTESIAN_POINT ( 'NONE',  ( -61.99999999999998579, 13.31249999999999822, 0.5000000000000013323 ) ) ;
#1667=ORIENTED_EDGE ( 'NONE', *, *, #3852, .T. ) ;
#1668=LINE ( 'NONE', #7665, #7103 ) ;
#1669=ORIENTED_EDGE ( 'NONE', *, *, #5664, .F. ) ;
#1670=CARTESIAN_POINT ( 'NONE',  ( -61.99999999999998579, 9.937500000000000000, 2.500000000000002665 ) ) ;
#1672=CARTESIAN_POINT ( 'NONE',  ( -62.86468353124999453, 14.95312499965860020, 1.500000000000002220 ) ) ;
#1673=CARTESIAN_POINT ( 'NONE',  ( -62.49999999999998579, 11.91666666666666607, 2.366025403784441483 ) ) ;
#1675=CARTESIAN_POINT ( 'NONE',  ( -61.99999999999998579, 10.81250000000000000, 0.5000000000000013323 ) ) ;
#1676=CARTESIAN_POINT ( 'NONE',  ( -62.43234176562499016, 13.30729166632526805, 2.248837904296538071 ) ) ;
#1677=CARTESIAN_POINT ( 'NONE',  ( -61.13531646874998415, 15.11979166632526628, 1.999225269531026417 ) ) ;
#1679=CARTESIAN_POINT ( 'NONE',  ( -60.99999999999998579, 9.270833333333333925, 0.9226497308103762673 ) ) ;
#1680=CARTESIAN_POINT ( 'NONE',  ( -62.86468353124998032, 9.244791666325268054, 1.000774730468978246 ) ) ;
#1681=CARTESIAN_POINT ( 'NONE',  ( -62.99999999999998579, 10.37500000000000000, 1.500000000000001998 ) ) ;
#1682=EDGE_LOOP ( 'NONE', ( #6021, #5235, #10747, #9316 ) ) ;
#1685=CARTESIAN_POINT ( 'NONE',  ( -62.86468353124999453, 14.97395833299193590, 1.999225269531025750 ) ) ;
#1686=CARTESIAN_POINT ( 'NONE',  ( -61.13531646874998415, 10.80729166632526628, 1.999225269531026417 ) ) ;
#1687=CARTESIAN_POINT ( 'NONE',  ( -62.86468353124998032, 15.49479166632526628, 1.000774730468978024 ) ) ;
#1689=EDGE_LOOP ( 'NONE', ( #1390, #4553, #3987, #4068 ) ) ;
#1690=CARTESIAN_POINT ( 'NONE',  ( -60.99999999999998579, 14.97916666666666785, 2.077350269189628840 ) ) ;
#1691=CARTESIAN_POINT ( 'NONE',  ( -61.99999999999999289, 9.078124999658601979, 2.498450539062049724 ) ) ;
#1692=CARTESIAN_POINT ( 'NONE',  ( -62.99999999999998579, 13.86458333265053611, 2.077350269189627952 ) ) ;
#1695=FACE_OUTER_BOUND ( 'NONE', #6216, .T. ) ;
#1696=CARTESIAN_POINT ( 'NONE',  ( -61.99999999999998579, 14.26562499965860020, 2.498450539062049724 ) ) ;
#1699=DIRECTION ( 'NONE',  ( -0.000000000000000000, -1.000000000000000000, -0.000000000000000000 ) ) ;
#1700=CARTESIAN_POINT ( 'NONE',  ( -61.56765823437498852, 13.09895833299193413, 2.248837904296538515 ) ) ;
#1701=FACE_OUTER_BOUND ( 'NONE', #4474, .T. ) ;
#1704=ORIENTED_EDGE ( 'NONE', *, *, #473, .T. ) ;
#1706=DIRECTION ( 'NONE',  ( 1.000000000000000000, 0.000000000000000000, 0.000000000000000000 ) ) ;
#1708=ADVANCED_FACE ( 'NONE', ( #1000 ), #1900, .T. ) ;
#1709=ORIENTED_EDGE ( 'NONE', *, *, #3265, .T. ) ;
#1710=CARTESIAN_POINT ( 'NONE',  ( -61.13531646874998415, 8.911458332991934128, 1.000774730468978468 ) ) ;
#1712=CARTESIAN_POINT ( 'NONE',  ( -61.99999999999998579, 12.82812499965860198, 2.498450539062049724 ) ) ;
#1716=ORIENTED_EDGE ( 'NONE', *, *, #3494, .T. ) ;
#1718=EDGE_CURVE ( 'NONE', #7701, #9934, #9836, .T. ) ;
#1719=CARTESIAN_POINT ( 'NONE',  ( -62.43234176562498305, 15.16145833299193590, 0.7511620957034662593 ) ) ;
#1720=CARTESIAN_POINT ( 'NONE',  ( -61.49999999999998579, 13.70833333333333215, 2.366025403784441927 ) ) ;
#1721=CARTESIAN_POINT ( 'NONE',  ( -61.73205080756886076, 12.41741454900183150, 2.500000000000003109 ) ) ;
#1722=DIRECTION ( 'NONE',  ( -0.000000000000000000, -1.000000000000000000, -0.000000000000000000 ) ) ;
#1723=CARTESIAN_POINT ( 'NONE',  ( -61.13531646874997705, 12.66145833299193413, 1.000774730468978468 ) ) ;
#1724=CARTESIAN_POINT ( 'NONE',  ( -62.86468353124999453, 8.703124999658601979, 1.500000000000002220 ) ) ;
#1727=CARTESIAN_POINT ( 'NONE',  ( -62.86468353124998032, 8.744791666325268054, 1.000774730468978246 ) ) ;
#1729=ORIENTED_EDGE ( 'NONE', *, *, #4171, .T. ) ;
#1730=LINE ( 'NONE', #6063, #2660 ) ;
#1732=EDGE_CURVE ( 'NONE', #1268, #9081, #3088, .T. ) ;
#1733=CARTESIAN_POINT ( 'NONE',  ( -62.43234176562499016, 15.99479166632526628, 2.248837904296538071 ) ) ;
#1734=EDGE_CURVE ( 'NONE', #6626, #1104, #4194, .T. ) ;
#1735=CARTESIAN_POINT ( 'NONE',  ( -62.86468353124999453, 10.70312499965860020, 1.500000000000002220 ) ) ;
#1736=AXIS2_PLACEMENT_3D ( 'NONE', #10398, #354, #10574 ) ;
#1737=CARTESIAN_POINT ( 'NONE',  ( -62.86468353124999453, 15.51562499965860198, 1.500000000000002220 ) ) ;
#1740=CARTESIAN_POINT ( 'NONE',  ( -62.99999999999998579, 15.37500000000000000, 1.500000000000001998 ) ) ;
#1742=CARTESIAN_POINT ( 'NONE',  ( -61.13531646874997705, 9.161458332991935904, 1.000774730468978468 ) ) ;
#1744=CARTESIAN_POINT ( 'NONE',  ( -61.99999999999998579, 13.03124999931720396, 0.3452994616207497591 ) ) ;
#1746=( BOUNDED_CURVE ( )  B_SPLINE_CURVE ( 2, ( #8611, #4210, #6836, #938, #5096, #990, #6109, #1778, #2555 ),
 .UNSPECIFIED., .F., .T. ) 
 B_SPLINE_CURVE_WITH_KNOTS ( ( 3, 2, 2, 2, 3 ),
 ( 0.5546875000000000000, 0.5572916666666666297, 0.5625000000000000000, 0.5677083333333333703, 0.5703125000000000000 ),
 .UNSPECIFIED. ) 
 CURVE ( )  GEOMETRIC_REPRESENTATION_ITEM ( )  RATIONAL_B_SPLINE_CURVE ( ( 0.9330127018922194093, 0.9330127018922194093, 1.000000000000000000, 0.8660254037844387076, 1.000000000000000000, 0.8660254037844387076, 1.000000000000000000, 0.9330127018922194093, 0.9330127018922194093 ) ) 
 REPRESENTATION_ITEM ( '' )  );
#1749=CARTESIAN_POINT ( 'NONE',  ( -61.99999999999999289, 10.89062499965859843, 0.5015494609379544944 ) ) ;
#1750=CYLINDRICAL_SURFACE ( 'NONE', #8142, 0.9999999999999981126 ) ;
#1754=CARTESIAN_POINT ( 'NONE',  ( -62.86468353124998032, 13.24479166632526983, 1.000774730468978246 ) ) ;
#1757=CARTESIAN_POINT ( 'NONE',  ( -61.99999999999998579, 9.781249999317202182, 0.3452994616207497591 ) ) ;
#1762=DIRECTION ( 'NONE',  ( -0.000000000000000000, -1.000000000000000000, -0.000000000000000000 ) ) ;
#1764=CARTESIAN_POINT ( 'NONE',  ( -61.56765823437498142, 11.86979166632526805, 0.7511620957034663704 ) ) ;
#1767=CARTESIAN_POINT ( 'NONE',  ( -61.56765823437498142, 8.682291666325268054, 0.7511620957034663704 ) ) ;
#1768=CARTESIAN_POINT ( 'NONE',  ( -61.73205080756886076, 14.30133545031537068, 0.5000000000000014433 ) ) ;
#1770=CARTESIAN_POINT ( 'NONE',  ( -62.86468353124998742, 12.78645833299193413, 1.999225269531025972 ) ) ;
#1772=ORIENTED_EDGE ( 'NONE', *, *, #2448, .F. ) ;
#1773=CARTESIAN_POINT ( 'NONE',  ( -61.99999999999998579, 16.00000000000000000, 2.500000000000000444 ) ) ;
#1775=CARTESIAN_POINT ( 'NONE',  ( -61.73205080756886076, 12.80133545031537068, 0.5000000000000014433 ) ) ;
#1776=CARTESIAN_POINT ( 'NONE',  ( -61.56765823437498852, 15.53645833299193590, 2.248837904296538515 ) ) ;
#1778=CARTESIAN_POINT ( 'NONE',  ( -61.73205080756886076, 12.55133545031537068, 0.5000000000000014433 ) ) ;
#1781=CARTESIAN_POINT ( 'NONE',  ( -62.43234176562498305, 13.97395833299193413, 0.7511620957034662593 ) ) ;
#1782=CARTESIAN_POINT ( 'NONE',  ( -62.86468353124998742, 9.223958332991935904, 1.999225269531025972 ) ) ;
#1783=CYLINDRICAL_SURFACE ( 'NONE', #3519, 0.9999999999999981126 ) ;
#1784=CARTESIAN_POINT ( 'NONE',  ( -61.73205080756886076, 13.52008544963257286, 0.5000000000000014433 ) ) ;
#1785=CARTESIAN_POINT ( 'NONE',  ( -61.13531646874998415, 8.869791666325268054, 1.999225269531026417 ) ) ;
#1786=CARTESIAN_POINT ( 'NONE',  ( -61.73205080756886076, 15.77008544963257108, 0.5000000000000014433 ) ) ;
#1787=ORIENTED_EDGE ( 'NONE', *, *, #2951, .T. ) ;
#1788=LINE ( 'NONE', #4220, #2469 ) ;
#1789=EDGE_CURVE ( 'NONE', #1800, #562, #3017, .T. ) ;
#1791=CARTESIAN_POINT ( 'NONE',  ( -62.86468353124999453, 15.72395833299193590, 1.999225269531025750 ) ) ;
#1792=CARTESIAN_POINT ( 'NONE',  ( -62.86468353124998032, 10.68229166632526628, 1.000774730468978246 ) ) ;
#1793=CARTESIAN_POINT ( 'NONE',  ( -62.43234176562498305, 8.911458332991934128, 0.7511620957034662593 ) ) ;
#1795=ORIENTED_EDGE ( 'NONE', *, *, #792, .F. ) ;
#1796=CARTESIAN_POINT ( 'NONE',  ( -61.99999999999998579, 14.43750000000000000, 2.654700538379254571 ) ) ;
#1797=CARTESIAN_POINT ( 'NONE',  ( -62.86468353124998032, 8.744791666325268054, 1.000774730468978024 ) ) ;
#1798=CARTESIAN_POINT ( 'NONE',  ( -62.99999999999998579, 13.82291666598387003, 0.9226497308103756012 ) ) ;
#1800=VERTEX_POINT ( 'NONE', #2187 ) ;
#1801=CARTESIAN_POINT ( 'NONE',  ( -61.49999999999998579, 9.708333333333332149, 2.366025403784441927 ) ) ;
#1803=CARTESIAN_POINT ( 'NONE',  ( -61.13531646874997705, 11.84895833299193413, 1.000774730468978468 ) ) ;
#1804=( LENGTH_UNIT ( ) NAMED_UNIT ( * ) SI_UNIT ( .MILLI., .METRE. ) );
#1805=DIRECTION ( 'NONE',  ( 0.000000000000000000, 0.000000000000000000, 1.000000000000000000 ) ) ;
#1806=ORIENTED_EDGE ( 'NONE', *, *, #7042, .F. ) ;
#1809=CARTESIAN_POINT ( 'NONE',  ( -62.86468353124998742, 13.03645833299193235, 1.999225269531025972 ) ) ;
#1810=( BOUNDED_CURVE ( )  B_SPLINE_CURVE ( 2, ( #3263, #3367, #815, #919, #8596, #5976, #7710, #6663, #3476 ),
 .UNSPECIFIED., .F., .T. ) 
 B_SPLINE_CURVE_WITH_KNOTS ( ( 3, 2, 2, 2, 3 ),
 ( 0.8359375000000000000, 0.8385416666666666297, 0.8437500000000000000, 0.8489583333333333703, 0.8515625000000000000 ),
 .UNSPECIFIED. ) 
 CURVE ( )  GEOMETRIC_REPRESENTATION_ITEM ( )  RATIONAL_B_SPLINE_CURVE ( ( 0.9330127018922194093, 0.9330127018922194093, 1.000000000000000000, 0.8660254037844387076, 1.000000000000000000, 0.8660254037844387076, 1.000000000000000000, 0.9330127018922194093, 0.9330127018922194093 ) ) 
 REPRESENTATION_ITEM ( '' )  );
#1811=CARTESIAN_POINT ( 'NONE',  ( -61.73205080756886076, 10.19866454968463110, 2.500000000000003109 ) ) ;
#1813=CARTESIAN_POINT ( 'NONE',  ( -61.99999999999998579, 8.906249999317203958, 2.654700538379254571 ) ) ;
#1815=ORIENTED_EDGE ( 'NONE', *, *, #7660, .F. ) ;
#1817=ORIENTED_EDGE ( 'NONE', *, *, #5195, .T. ) ;
#1818=DIRECTION ( 'NONE',  ( -0.000000000000000000, -1.000000000000000000, -0.000000000000000000 ) ) ;
#1819=VECTOR ( 'NONE', #10581, 1000.000000000000000 ) ;
#1820=CARTESIAN_POINT ( 'NONE',  ( -62.86468353124999453, 11.95312499965860198, 1.500000000000002220 ) ) ;
#1823=CARTESIAN_POINT ( 'NONE',  ( -61.13531646874998415, 9.161458332991935904, 1.000774730468978468 ) ) ;
#1826=CARTESIAN_POINT ( 'NONE',  ( -62.86468353124999453, 13.51562499965860020, 1.500000000000002220 ) ) ;
#1830=ADVANCED_FACE ( 'NONE', ( #9009 ), #10511, .T. ) ;
#1832=ORIENTED_EDGE ( 'NONE', *, *, #8649, .T. ) ;
#1834=CARTESIAN_POINT ( 'NONE',  ( -61.49999999999998579, 13.26041666598387003, 0.6339745962155628467 ) ) ;
#1835=CARTESIAN_POINT ( 'NONE',  ( -61.13531646874998415, 14.80729166632526805, 1.999225269531026417 ) ) ;
#1836=CARTESIAN_POINT ( 'NONE',  ( -62.99999999999998579, 9.875000000000000000, 1.500000000000001998 ) ) ;
#1838=LINE ( 'NONE', #8612, #6358 ) ;
#1839=CARTESIAN_POINT ( 'NONE',  ( -62.86468353124998032, 13.99479166632526983, 1.000774730468978024 ) ) ;
#1840=CARTESIAN_POINT ( 'NONE',  ( -61.99999999999998579, 9.015624999658603755, 2.498450539062049724 ) ) ;
#1841=CARTESIAN_POINT ( 'NONE',  ( -61.99999999999998579, 16.00000000000000000, 1.500000000000002220 ) ) ;
#1843=CARTESIAN_POINT ( 'NONE',  ( -61.56765823437498142, 9.432291666325268054, 0.7511620957034663704 ) ) ;
#1847=CARTESIAN_POINT ( 'NONE',  ( -62.99999999999998579, 11.37500000000000000, 1.500000000000001998 ) ) ;
#1848=EDGE_CURVE ( 'NONE', #7344, #9337, #10951, .T. ) ;
#1849=CARTESIAN_POINT ( 'NONE',  ( -61.13531646874997705, 15.09895833299193590, 1.000774730468978468 ) ) ;
#1850=CARTESIAN_POINT ( 'NONE',  ( -61.56765823437498142, 11.36979166632526805, 0.7511620957034663704 ) ) ;
#1851=CARTESIAN_POINT ( 'NONE',  ( -62.86468353124999453, 8.973958332991934128, 1.999225269531025750 ) ) ;
#1854=CARTESIAN_POINT ( 'NONE',  ( -61.99999999999998579, 15.18750000000000000, 2.654700538379254571 ) ) ;
#1855=EDGE_CURVE ( 'NONE', #9209, #7667, #1091, .T. ) ;
#1856=CARTESIAN_POINT ( 'NONE',  ( -61.13531646874997705, 10.16145833299193413, 1.000774730468978468 ) ) ;
#1857=CARTESIAN_POINT ( 'NONE',  ( -62.49999999999998579, 13.05208333265053611, 0.6339745962155627357 ) ) ;
#1859=ORIENTED_EDGE ( 'NONE', *, *, #4382, .F. ) ;
#1860=DIRECTION ( 'NONE',  ( -0.000000000000000000, -1.000000000000000000, -0.000000000000000000 ) ) ;
#1861=CARTESIAN_POINT ( 'NONE',  ( -61.13531646874998415, 11.07812499965860020, 1.500000000000002220 ) ) ;
#1862=DIRECTION ( 'NONE',  ( -0.000000000000000000, -1.000000000000000000, -0.000000000000000000 ) ) ;
#1863=DIRECTION ( 'NONE',  ( 0.000000000000000000, 1.000000000000000000, 0.000000000000000000 ) ) ;
#1864=ORIENTED_EDGE ( 'NONE', *, *, #5528, .T. ) ;
#1865=CARTESIAN_POINT ( 'NONE',  ( -62.49999999999998579, 10.66666666666666607, 2.366025403784441483 ) ) ;
#1867=CARTESIAN_POINT ( 'NONE',  ( -61.56765823437498852, 14.34895833299193413, 2.248837904296538515 ) ) ;
#1869=CARTESIAN_POINT ( 'NONE',  ( -61.73205080756886076, 10.94866454968462932, 2.500000000000003109 ) ) ;
#1870=CARTESIAN_POINT ( 'NONE',  ( -60.99999999999998579, 9.468749999317202182, 1.500000000000002220 ) ) ;
#1871=ORIENTED_EDGE ( 'NONE', *, *, #5613, .T. ) ;
#1875=CARTESIAN_POINT ( 'NONE',  ( -61.13531646874998415, 11.07812499965860020, 1.500000000000002220 ) ) ;
#1878=( BOUNDED_CURVE ( )  B_SPLINE_CURVE ( 2, ( #5392, #411, #5509, #8913, #1301, #4676, #3850, #6414, #2190 ),
 .UNSPECIFIED., .F., .T. ) 
 B_SPLINE_CURVE_WITH_KNOTS ( ( 3, 2, 2, 2, 3 ),
 ( 0.2421874999999999722, 0.2447916666666666574, 0.2500000000000000000, 0.2552083333333333148, 0.2578125000000000000 ),
 .UNSPECIFIED. ) 
 CURVE ( )  GEOMETRIC_REPRESENTATION_ITEM ( )  RATIONAL_B_SPLINE_CURVE ( ( 0.9330127018922194093, 0.9330127018922186322, 1.000000000000000000, 0.8660254037844387076, 1.000000000000000000, 0.8660254037844387076, 1.000000000000000000, 0.9330127018922194093, 0.9330127018922194093 ) ) 
 REPRESENTATION_ITEM ( '' )  );
#1879=VERTEX_POINT ( 'NONE', #8083 ) ;
#1880=CARTESIAN_POINT ( 'NONE',  ( -61.13531646874998415, 9.140624999658601979, 1.500000000000002220 ) ) ;
#1882=CARTESIAN_POINT ( 'NONE',  ( -61.99999999999998579, 15.07812499965860198, 2.498450539062049724 ) ) ;
#1883=CARTESIAN_POINT ( 'NONE',  ( -60.99999999999998579, 13.25000000000000000, 1.500000000000002220 ) ) ;
#1884=ORIENTED_EDGE ( 'NONE', *, *, #4763, .F. ) ;
#1885=CARTESIAN_POINT ( 'NONE',  ( -61.99999999999998579, 16.00000000000000000, 0.5000000000000041078 ) ) ;
#1887=CARTESIAN_POINT ( 'NONE',  ( -61.99999999999998579, 8.062500000000000000, 0.3452994616207497591 ) ) ;
#1890=CARTESIAN_POINT ( 'NONE',  ( -61.99999999999997868, 10.65624999931720218, 2.500000000000002665 ) ) ;
#1891=CARTESIAN_POINT ( 'NONE',  ( -61.13531646874997705, 13.66145833299193413, 1.000774730468978468 ) ) ;
#1892=EDGE_CURVE ( 'NONE', #10833, #10050, #5506, .T. ) ;
#1893=CARTESIAN_POINT ( 'NONE',  ( -61.13531646874998415, 8.557291666325268054, 1.999225269531026417 ) ) ;
#1894=DIRECTION ( 'NONE',  ( -0.000000000000000000, -1.000000000000000000, -0.000000000000000000 ) ) ;
#1896=CARTESIAN_POINT ( 'NONE',  ( -61.56765823437498852, 9.848958332991934128, 2.248837904296538515 ) ) ;
#1899=CARTESIAN_POINT ( 'NONE',  ( -61.99999999999998579, 10.15624999931720041, 2.500000000000002665 ) ) ;
#1900=CYLINDRICAL_SURFACE ( 'NONE', #44, 0.9999999999999981126 ) ;
#1901=CARTESIAN_POINT ( 'NONE',  ( -62.86468353124999453, 15.95312499965860198, 1.500000000000002220 ) ) ;
#1902=CARTESIAN_POINT ( 'NONE',  ( -62.86468353124998032, 12.18229166632526805, 1.000774730468978246 ) ) ;
#1903=CARTESIAN_POINT ( 'NONE',  ( -62.86468353124999453, 9.203124999658600203, 1.500000000000002220 ) ) ;
#1906=CARTESIAN_POINT ( 'NONE',  ( -60.99999999999998579, 14.77083333333333570, 0.9226497308103762673 ) ) ;
#1907=CARTESIAN_POINT ( 'NONE',  ( -61.13531646874997705, 10.11979166632526805, 1.999225269531026417 ) ) ;
#1910=CARTESIAN_POINT ( 'NONE',  ( -61.56765823437498142, 15.36979166632526805, 0.7511620957034663704 ) ) ;
#1911=CARTESIAN_POINT ( 'NONE',  ( -62.99999999999998579, 12.61458333265053611, 2.077350269189627952 ) ) ;
#1915=CARTESIAN_POINT ( 'NONE',  ( -61.13531646874997705, 11.80729166632526805, 1.999225269531026417 ) ) ;
#1919=CARTESIAN_POINT ( 'NONE',  ( -61.49999999999998579, 11.20833333333333393, 2.366025403784441927 ) ) ;
#1920=DIRECTION ( 'NONE',  ( -0.000000000000000000, -1.000000000000000000, -0.000000000000000000 ) ) ;
#1921=CARTESIAN_POINT ( 'NONE',  ( -61.99999999999998579, 13.82812499965860198, 2.498450539062049724 ) ) ;
#1922=CARTESIAN_POINT ( 'NONE',  ( -61.49999999999998579, 10.29166666666666785, 0.6339745962155628467 ) ) ;
#1924=CARTESIAN_POINT ( 'NONE',  ( -61.49999999999998579, 9.427083332650536107, 2.366025403784441927 ) ) ;
#1925=VERTEX_POINT ( 'NONE', #1178 ) ;
#1926=CARTESIAN_POINT ( 'NONE',  ( -60.99999999999998579, 14.02083333333333215, 0.9226497308103762673 ) ) ;
#1930=CARTESIAN_POINT ( 'NONE',  ( -61.99999999999998579, 10.64062499965860376, 0.5015494609379544944 ) ) ;
#1931=AXIS2_PLACEMENT_3D ( 'NONE', #7, #8563, #10163 ) ;
#1933=CARTESIAN_POINT ( 'NONE',  ( -62.86468353124998032, 10.24479166632526983, 1.000774730468978246 ) ) ;
#1937=CARTESIAN_POINT ( 'NONE',  ( -61.13531646874998415, 14.14062499965860198, 1.500000000000002220 ) ) ;
#1941=( BOUNDED_CURVE ( )  B_SPLINE_CURVE ( 2, ( #1628, #7521, #7415, #6741, #1524 ),
 .UNSPECIFIED., .F., .T. ) 
 B_SPLINE_CURVE_WITH_KNOTS ( ( 3, 2, 3 ),
 ( 0.000000000000000000, 0.005208333333333333044, 0.007812499999999973112 ),
 .UNSPECIFIED. ) 
 CURVE ( )  GEOMETRIC_REPRESENTATION_ITEM ( )  RATIONAL_B_SPLINE_CURVE ( ( 1.000000000000000000, 0.8660254037844387076, 1.000000000000000000, 0.9330127018922200755, 0.9330127018922194093 ) ) 
 REPRESENTATION_ITEM ( '' )  );
#1943=LINE ( 'NONE', #3717, #5718 ) ;
#1944=CARTESIAN_POINT ( 'NONE',  ( -61.56765823437498142, 15.86979166632526628, 0.7511620957034663704 ) ) ;
#1949=CARTESIAN_POINT ( 'NONE',  ( -61.13531646874997705, 14.16145833299193413, 1.000774730468978468 ) ) ;
#1950=CARTESIAN_POINT ( 'NONE',  ( -62.86468353124998742, 8.223958332991934128, 1.999225269531025972 ) ) ;
#1954=CARTESIAN_POINT ( 'NONE',  ( -61.13531646874998415, 10.64062499965860198, 1.500000000000002220 ) ) ;
#1956=CARTESIAN_POINT ( 'NONE',  ( -61.06765823437498852, 8.039062499829300990, 1.500000000000002220 ) ) ;
#1958=CARTESIAN_POINT ( 'NONE',  ( -60.99999999999998579, 11.19791666598387003, 2.077350269189628840 ) ) ;
#1959=AXIS2_PLACEMENT_3D ( 'NONE', #975, #1818, #4248 ) ;
#1960=CARTESIAN_POINT ( 'NONE',  ( -61.49999999999998579, 10.04166666666666785, 0.6339745962155628467 ) ) ;
#1961=CARTESIAN_POINT ( 'NONE',  ( -62.86468353124999453, 12.20312499965860198, 1.500000000000002220 ) ) ;
#1962=CARTESIAN_POINT ( 'NONE',  ( -62.86468353124999453, 8.453124999658601979, 1.500000000000002220 ) ) ;
#1964=ORIENTED_EDGE ( 'NONE', *, *, #9119, .F. ) ;
#1966=CARTESIAN_POINT ( 'NONE',  ( -61.13531646874998415, 9.890624999658601979, 1.500000000000002220 ) ) ;
#1968=CARTESIAN_POINT ( 'NONE',  ( -61.13531646874998415, 14.80729166632526805, 1.999225269531026417 ) ) ;
#1969=CARTESIAN_POINT ( 'NONE',  ( -61.99999999999998579, 14.65624999931720218, 2.654700538379254571 ) ) ;
#1971=ORIENTED_EDGE ( 'NONE', *, *, #7541, .F. ) ;
#1973=ADVANCED_FACE ( 'NONE', ( #9068 ), #4833, .T. ) ;
#1974=CARTESIAN_POINT ( 'NONE',  ( -62.86468353124999453, 13.22395833299193235, 1.999225269531025750 ) ) ;
#1975=CARTESIAN_POINT ( 'NONE',  ( -62.86468353124999453, 8.453124999658601979, 1.500000000000002220 ) ) ;
#1976=CARTESIAN_POINT ( 'NONE',  ( -62.26794919243111082, 8.323664549684629321, 0.5000000000000025535 ) ) ;
#1978=CARTESIAN_POINT ( 'NONE',  ( -61.49999999999998579, 11.95833333333333215, 2.366025403784441927 ) ) ;
#1980=CARTESIAN_POINT ( 'NONE',  ( -62.43234176562498305, 13.97395833299193413, 0.7511620957034662593 ) ) ;
#1982=CARTESIAN_POINT ( 'NONE',  ( -62.99999999999998579, 13.87500000000000000, 1.500000000000001998 ) ) ;
#1983=CARTESIAN_POINT ( 'NONE',  ( -62.49999999999998579, 10.05208333265053611, 0.6339745962155627357 ) ) ;
#1985=CARTESIAN_POINT ( 'NONE',  ( -61.49999999999998579, 13.45833333333333215, 2.366025403784441927 ) ) ;
#1986=CARTESIAN_POINT ( 'NONE',  ( -61.99999999999998579, 9.906249999317202182, 2.500000000000002665 ) ) ;
#1988=CARTESIAN_POINT ( 'NONE',  ( -62.43234176562499016, 11.49479166632526805, 2.248837904296538071 ) ) ;
#1989=ORIENTED_EDGE ( 'NONE', *, *, #6880, .T. ) ;
#1990=AXIS2_PLACEMENT_3D ( 'NONE', #9562, #3499, #838 ) ;
#1991=CARTESIAN_POINT ( 'NONE',  ( -61.99999999999998579, 9.828124999658600203, 2.498450539062049724 ) ) ;
#1994=CARTESIAN_POINT ( 'NONE',  ( -62.43234176562498305, 13.97395833299193413, 0.7511620957034662593 ) ) ;
#1999=AXIS2_PLACEMENT_3D ( 'NONE', #9122, #4884, #8287 ) ;
#2000=ORIENTED_EDGE ( 'NONE', *, *, #3278, .T. ) ;
#2001=CARTESIAN_POINT ( 'NONE',  ( -62.99999999999998579, 15.11458333265053433, 2.077350269189627952 ) ) ;
#2002=CARTESIAN_POINT ( 'NONE',  ( -62.49999999999998579, 8.833333333333333925, 0.6339745962155627357 ) ) ;
#2003=CARTESIAN_POINT ( 'NONE',  ( -61.99999999999998579, 10.18750000000000000, 2.500000000000002665 ) ) ;
#2007=CARTESIAN_POINT ( 'NONE',  ( -61.99999999999999289, 14.45312499965860020, 0.5015494609379544944 ) ) ;
#2009=CARTESIAN_POINT ( 'NONE',  ( -62.43234176562498305, 9.911458332991934128, 0.7511620957034662593 ) ) ;
#2010=CARTESIAN_POINT ( 'NONE',  ( -61.99999999999998579, 11.40624999931720218, 2.500000000000002665 ) ) ;
#2012=CARTESIAN_POINT ( 'NONE',  ( -61.13531646874998415, 10.91145833299193590, 1.000774730468978468 ) ) ;
#2013=CARTESIAN_POINT ( 'NONE',  ( -62.99999999999998579, 12.12500000000000000, 1.500000000000001998 ) ) ;
#2016=CARTESIAN_POINT ( 'NONE',  ( -61.73205080756886076, 15.19866454968462932, 2.500000000000003109 ) ) ;
#2018=VERTEX_POINT ( 'NONE', #7805 ) ;
#2019=CARTESIAN_POINT ( 'NONE',  ( -61.49999999999998579, 9.958333333333332149, 2.366025403784441927 ) ) ;
#2020=CARTESIAN_POINT ( 'NONE',  ( -61.13531646874998415, 13.09895833299193413, 1.000774730468978468 ) ) ;
#2022=CARTESIAN_POINT ( 'NONE',  ( -61.99999999999999289, 9.390624999658600203, 0.5015494609379544944 ) ) ;
#2023=CARTESIAN_POINT ( 'NONE',  ( -62.49999999999998579, 8.666666666666666075, 2.366025403784441483 ) ) ;
#2024=ORIENTED_EDGE ( 'NONE', *, *, #4812, .F. ) ;
#2025=CARTESIAN_POINT ( 'NONE',  ( -61.49999999999998579, 8.427083332650536107, 2.366025403784441927 ) ) ;
#2026=CARTESIAN_POINT ( 'NONE',  ( -61.13531646874998415, 10.39062499965860198, 1.500000000000002220 ) ) ;
#2027=CARTESIAN_POINT ( 'NONE',  ( -62.86468353124999453, 15.95312499965860198, 1.500000000000002220 ) ) ;
#2029=CARTESIAN_POINT ( 'NONE',  ( -62.99999999999998579, 14.34374999931720041, 1.500000000000001998 ) ) ;
#2031=EDGE_LOOP ( 'NONE', ( #10627, #10777, #9434, #3454 ) ) ;
#2033=CARTESIAN_POINT ( 'NONE',  ( -62.43234176562499016, 13.24479166632526805, 2.248837904296538071 ) ) ;
#2034=CARTESIAN_POINT ( 'NONE',  ( -61.13531646874998415, 8.307291666325269830, 1.999225269531026417 ) ) ;
#2035=DIRECTION ( 'NONE',  ( -0.000000000000000000, -1.000000000000000000, -0.000000000000000000 ) ) ;
#2037=CARTESIAN_POINT ( 'NONE',  ( -60.99999999999998579, 12.02083333333333393, 0.9226497308103762673 ) ) ;
#2039=CARTESIAN_POINT ( 'NONE',  ( -62.43234176562498305, 14.22395833299193413, 0.7511620957034662593 ) ) ;
#2041=CARTESIAN_POINT ( 'NONE',  ( -61.49999999999998579, 10.95833333333333393, 2.366025403784441927 ) ) ;
#2043=CARTESIAN_POINT ( 'NONE',  ( -61.49999999999998579, 10.51041666598387003, 0.6339745962155628467 ) ) ;
#2048=CARTESIAN_POINT ( 'NONE',  ( -62.43234176562498305, 12.41145833299193413, 0.7511620957034662593 ) ) ;
#2049=ORIENTED_EDGE ( 'NONE', *, *, #7739, .T. ) ;
#2050=CARTESIAN_POINT ( 'NONE',  ( -61.99999999999998579, 9.953124999658601979, 0.5015494609379544944 ) ) ;
#2052=CARTESIAN_POINT ( 'NONE',  ( -61.99999999999998579, 13.95312499965860198, 0.5015494609379544944 ) ) ;
#2058=CARTESIAN_POINT ( 'NONE',  ( -60.99999999999998579, 8.729166666666666075, 2.077350269189628840 ) ) ;
#2059=CARTESIAN_POINT ( 'NONE',  ( -62.99999999999998579, 8.145833333333332149, 2.077350269189627952 ) ) ;
#2060=LINE ( 'NONE', #9889, #6469 ) ;
#2063=CARTESIAN_POINT ( 'NONE',  ( -61.13531646874997705, 14.91145833299193768, 1.000774730468978468 ) ) ;
#2064=CARTESIAN_POINT ( 'NONE',  ( -61.99999999999998579, 9.640624999658600203, 0.5015494609379544944 ) ) ;
#2066=CARTESIAN_POINT ( 'NONE',  ( -61.49999999999998579, 12.01041666598387003, 0.6339745962155628467 ) ) ;
#2068=CARTESIAN_POINT ( 'NONE',  ( -61.13531646874998415, 10.86979166632526805, 1.999225269531026417 ) ) ;
#2070=VERTEX_POINT ( 'NONE', #9406 ) ;
#2071=CARTESIAN_POINT ( 'NONE',  ( -62.49999999999998579, 14.41666666666666785, 2.366025403784441483 ) ) ;
#2074=ORIENTED_EDGE ( 'NONE', *, *, #388, .F. ) ;
#2075=CARTESIAN_POINT ( 'NONE',  ( -61.99999999999998579, 9.937500000000000000, 2.500000000000002665 ) ) ;
#2076=CARTESIAN_POINT ( 'NONE',  ( -61.13531646874998415, 12.57812499965860198, 1.500000000000002220 ) ) ;
#2077=CARTESIAN_POINT ( 'NONE',  ( -62.43234176562498305, 10.66145833299193413, 0.7511620957034662593 ) ) ;
#2078=ORIENTED_EDGE ( 'NONE', *, *, #7061, .F. ) ;
#2080=CARTESIAN_POINT ( 'NONE',  ( -61.56765823437498142, 10.68229166632526805, 0.7511620957034663704 ) ) ;
#2082=CARTESIAN_POINT ( 'NONE',  ( -61.56765823437498142, 15.86979166632526628, 0.7511620957034663704 ) ) ;
#2083=CARTESIAN_POINT ( 'NONE',  ( -61.99999999999998579, 14.53124999931720041, 0.3452994616207497591 ) ) ;
#2085=ORIENTED_EDGE ( 'NONE', *, *, #4471, .T. ) ;
#2087=ORIENTED_EDGE ( 'NONE', *, *, #4800, .F. ) ;
#2089=CARTESIAN_POINT ( 'NONE',  ( -62.86468353124999453, 13.20312499965860198, 1.500000000000002220 ) ) ;
#2093=CARTESIAN_POINT ( 'NONE',  ( -60.99999999999998579, 12.75000000000000178, 1.500000000000002220 ) ) ;
#2095=CARTESIAN_POINT ( 'NONE',  ( -62.43234176562499016, 14.80729166632526805, 2.248837904296538071 ) ) ;
#2096=EDGE_CURVE ( 'NONE', #5931, #918, #4917, .T. ) ;
#2097=CARTESIAN_POINT ( 'NONE',  ( -62.49999999999998579, 10.63541666598387003, 2.366025403784441483 ) ) ;
#2102=CARTESIAN_POINT ( 'NONE',  ( -62.86468353124998032, 12.68229166632526983, 1.000774730468978246 ) ) ;
#2104=ORIENTED_EDGE ( 'NONE', *, *, #9938, .F. ) ;
#2105=CARTESIAN_POINT ( 'NONE',  ( -61.13531646874998415, 10.86979166632526805, 1.999225269531026417 ) ) ;
#2106=CARTESIAN_POINT ( 'NONE',  ( -62.26794919243111082, 15.64508544963257108, 2.500000000000003109 ) ) ;
#2108=CARTESIAN_POINT ( 'NONE',  ( -62.43234176562499016, 14.30729166632526983, 2.248837904296538071 ) ) ;
#2111=( BOUNDED_CURVE ( )  B_SPLINE_CURVE ( 2, ( #4831, #5774, #10049, #4051, #9169, #4722, #8337, #4106, #9897 ),
 .UNSPECIFIED., .F., .T. ) 
 B_SPLINE_CURVE_WITH_KNOTS ( ( 3, 2, 2, 2, 3 ),
 ( 0.9140625000000000000, 0.9166666666666666297, 0.9218750000000000000, 0.9270833333333333703, 0.9296875000000000000 ),
 .UNSPECIFIED. ) 
 CURVE ( )  GEOMETRIC_REPRESENTATION_ITEM ( )  RATIONAL_B_SPLINE_CURVE ( ( 0.9330127018922194093, 0.9330127018922194093, 1.000000000000000000, 0.8660254037844387076, 1.000000000000000000, 0.8660254037844387076, 1.000000000000000000, 0.9330127018922194093, 0.9330127018922194093 ) ) 
 REPRESENTATION_ITEM ( '' )  );
#2112=CARTESIAN_POINT ( 'NONE',  ( -61.49999999999998579, 10.54166666666666607, 0.6339745962155628467 ) ) ;
#2113=AXIS2_PLACEMENT_3D ( 'NONE', #1593, #5867, #8534 ) ;
#2116=CARTESIAN_POINT ( 'NONE',  ( -61.49999999999998579, 8.958333333333333925, 2.366025403784441927 ) ) ;
#2117=CARTESIAN_POINT ( 'NONE',  ( -61.99999999999997868, 9.656249999317202182, 2.500000000000002665 ) ) ;
#2119=CARTESIAN_POINT ( 'NONE',  ( -62.26794919243111082, 8.926335450315370679, 2.500000000000004885 ) ) ;
#2121=CARTESIAN_POINT ( 'NONE',  ( -62.86468353124999453, 9.703124999658601979, 1.500000000000002220 ) ) ;
#2124=CARTESIAN_POINT ( 'NONE',  ( -62.86468353124999453, 10.51562499965860198, 1.500000000000002220 ) ) ;
#2133=ORIENTED_EDGE ( 'NONE', *, *, #1855, .T. ) ;
#2134=CARTESIAN_POINT ( 'NONE',  ( -62.99999999999998579, 10.11458333265053611, 2.077350269189627952 ) ) ;
#2135=CARTESIAN_POINT ( 'NONE',  ( -61.13531646874998415, 12.59895833299193590, 1.000774730468978468 ) ) ;
#2136=CARTESIAN_POINT ( 'NONE',  ( -61.56765823437498852, 10.78645833299193413, 2.248837904296538515 ) ) ;
#2138=CARTESIAN_POINT ( 'NONE',  ( -61.13531646874998415, 8.109374999658601979, 1.500000000000002220 ) ) ;
#2139=ORIENTED_EDGE ( 'NONE', *, *, #8375, .F. ) ;
#2141=CARTESIAN_POINT ( 'NONE',  ( -62.86468353124999453, 11.76562499965860198, 1.500000000000002220 ) ) ;
#2142=CARTESIAN_POINT ( 'NONE',  ( -62.86468353124999453, 15.20312499965860020, 1.500000000000002220 ) ) ;
#2145=CARTESIAN_POINT ( 'NONE',  ( -60.99999999999998579, 14.73958333265053433, 0.9226497308103762673 ) ) ;
#2146=CARTESIAN_POINT ( 'NONE',  ( -60.99999999999998579, 14.73958333265053433, 0.9226497308103762673 ) ) ;
#2147=ORIENTED_EDGE ( 'NONE', *, *, #4001, .T. ) ;
#2150=PRODUCT_DEFINITION_FORMATION_WITH_SPECIFIED_SOURCE ( 'ANY', '', #7593, .NOT_KNOWN. ) ;
#2151=CARTESIAN_POINT ( 'NONE',  ( -61.99999999999999289, 12.76562499965860198, 2.498450539062049724 ) ) ;
#2152=CARTESIAN_POINT ( 'NONE',  ( -61.56765823437498142, 8.369791666325268054, 0.7511620957034663704 ) ) ;
#2153=CARTESIAN_POINT ( 'NONE',  ( -62.49999999999998579, 10.55208333265053611, 0.6339745962155627357 ) ) ;
#2154=EDGE_LOOP ( 'NONE', ( #269, #8721, #5421, #5391 ) ) ;
#2155=CARTESIAN_POINT ( 'NONE',  ( -61.49999999999998579, 12.20833333333333393, 2.366025403784441927 ) ) ;
#2156=CARTESIAN_POINT ( 'NONE',  ( -61.73205080756886076, 9.051335450315368902, 0.5000000000000014433 ) ) ;
#2158=CARTESIAN_POINT ( 'NONE',  ( -62.99999999999998579, 10.57291666598387181, 0.9226497308103756012 ) ) ;
#2159=ORIENTED_EDGE ( 'NONE', *, *, #1003, .F. ) ;
#2160=CARTESIAN_POINT ( 'NONE',  ( -61.99999999999998579, 14.81250000000000000, 0.5000000000000013323 ) ) ;
#2161=CARTESIAN_POINT ( 'NONE',  ( -62.43234176562499016, 13.24479166632526805, 2.248837904296538071 ) ) ;
#2163=CARTESIAN_POINT ( 'NONE',  ( -61.73205080756886076, 15.94866454968462932, 2.500000000000003109 ) ) ;
#2165=EDGE_CURVE ( 'NONE', #8943, #4570, #7621, .T. ) ;
#2166=CARTESIAN_POINT ( 'NONE',  ( -61.56765823437498142, 9.682291666325268054, 0.7511620957034663704 ) ) ;
#2168=CARTESIAN_POINT ( 'NONE',  ( -61.56765823437498852, 15.84895833299193590, 2.248837904296538515 ) ) ;
#2169=CYLINDRICAL_SURFACE ( 'NONE', #5717, 0.9999999999999981126 ) ;
#2170=ORIENTED_EDGE ( 'NONE', *, *, #9568, .T. ) ;
#2173=CARTESIAN_POINT ( 'NONE',  ( -61.49999999999998579, 9.208333333333333925, 2.366025403784441927 ) ) ;
#2177=CARTESIAN_POINT ( 'NONE',  ( -61.13531646874998415, 9.807291666325268054, 1.999225269531026417 ) ) ;
#2178=( BOUNDED_CURVE ( )  B_SPLINE_CURVE ( 2, ( #10729, #4877, #5769, #6460, #6567, #8279, #1548, #2230, #10773 ),
 .UNSPECIFIED., .F., .F. ) 
 B_SPLINE_CURVE_WITH_KNOTS ( ( 3, 2, 2, 2, 3 ),
 ( 0.5234375000000000000, 0.5260416666666666297, 0.5312500000000000000, 0.5364583333333333703, 0.5390625000000000000 ),
 .UNSPECIFIED. ) 
 CURVE ( )  GEOMETRIC_REPRESENTATION_ITEM ( )  RATIONAL_B_SPLINE_CURVE ( ( 0.9330127018922194093, 0.9330127018922194093, 1.000000000000000000, 0.8660254037844387076, 1.000000000000000000, 0.8660254037844387076, 1.000000000000000000, 0.9330127018922194093, 0.9330127018922194093 ) ) 
 REPRESENTATION_ITEM ( '' )  );
#2179=CARTESIAN_POINT ( 'NONE',  ( -60.99999999999998579, 15.46874999931720218, 1.500000000000002220 ) ) ;
#2180=VECTOR ( 'NONE', #5441, 1000.000000000000000 ) ;
#2183=CARTESIAN_POINT ( 'NONE',  ( -61.56765823437498142, 12.18229166632526628, 0.7511620957034663704 ) ) ;
#2185=EDGE_LOOP ( 'NONE', ( #5410, #8896, #7323, #9641 ) ) ;
#2187=CARTESIAN_POINT ( 'NONE',  ( -61.99999999999998579, 12.68750000000000000, 2.500000000000002665 ) ) ;
#2190=CARTESIAN_POINT ( 'NONE',  ( -61.99999999999998579, 10.28124999931720218, 0.5000000000000013323 ) ) ;
#2191=CARTESIAN_POINT ( 'NONE',  ( -61.56765823437498852, 13.78645833299193413, 2.248837904296538515 ) ) ;
#2193=CARTESIAN_POINT ( 'NONE',  ( -62.86468353124999453, 9.973958332991932352, 1.999225269531025750 ) ) ;
#2194=CARTESIAN_POINT ( 'NONE',  ( -62.99999999999998579, 8.625000000000000000, 1.500000000000001998 ) ) ;
#2195=ORIENTED_EDGE ( 'NONE', *, *, #1204, .F. ) ;
#2197=CARTESIAN_POINT ( 'NONE',  ( -62.86468353124999453, 11.53645833299193413, 1.999225269531025750 ) ) ;
#2200=CARTESIAN_POINT ( 'NONE',  ( -61.49999999999998579, 14.92708333265053611, 2.366025403784441927 ) ) ;
#2202=VERTEX_POINT ( 'NONE', #3083 ) ;
#2203=CARTESIAN_POINT ( 'NONE',  ( -60.99999999999998579, 15.19791666598387359, 2.077350269189628840 ) ) ;
#2205=CARTESIAN_POINT ( 'NONE',  ( -62.86468353124999453, 13.47395833299193413, 1.999225269531025750 ) ) ;
#2206=CARTESIAN_POINT ( 'NONE',  ( -61.99999999999998579, 8.765624999658601979, 2.498450539062049724 ) ) ;
#2207=CARTESIAN_POINT ( 'NONE',  ( -61.99999999999998579, 8.000000000000000000, 1.500000000000002220 ) ) ;
#2209=CARTESIAN_POINT ( 'NONE',  ( -62.49999999999998579, 12.66666666666666607, 2.366025403784441483 ) ) ;
#2211=CARTESIAN_POINT ( 'NONE',  ( -62.26794919243110371, 8.542414549001833279, 0.5000000000000032196 ) ) ;
#2212=CARTESIAN_POINT ( 'NONE',  ( -60.99999999999998579, 15.02083333333333393, 0.9226497308103762673 ) ) ;
#2213=CARTESIAN_POINT ( 'NONE',  ( -60.99999999999998579, 10.73958333265053611, 0.9226497308103762673 ) ) ;
#2214=ORIENTED_EDGE ( 'NONE', *, *, #5371, .F. ) ;
#2216=CARTESIAN_POINT ( 'NONE',  ( -61.56765823437498852, 13.03645833299193413, 2.248837904296538515 ) ) ;
#2219=CARTESIAN_POINT ( 'NONE',  ( -61.13531646874998415, 11.64062499965860198, 1.500000000000002220 ) ) ;
#2220=DIRECTION ( 'NONE',  ( -0.000000000000000000, -1.000000000000000000, -0.000000000000000000 ) ) ;
#2221=CARTESIAN_POINT ( 'NONE',  ( -62.86468353124998742, 15.53645833299193590, 1.999225269531025972 ) ) ;
#2222=VERTEX_POINT ( 'NONE', #7250 ) ;
#2223=CARTESIAN_POINT ( 'NONE',  ( -61.99999999999998579, 16.00000000000000000, 1.500000000000002220 ) ) ;
#2226=FACE_OUTER_BOUND ( 'NONE', #4710, .T. ) ;
#2227=CARTESIAN_POINT ( 'NONE',  ( -62.49999999999998579, 10.33333333333333393, 0.6339745962155627357 ) ) ;
#2228=CARTESIAN_POINT ( 'NONE',  ( -61.99999999999998579, 9.531249999317202182, 0.5000000000000013323 ) ) ;
#2229=CARTESIAN_POINT ( 'NONE',  ( -60.99999999999998579, 8.500000000000000000, 1.500000000000002220 ) ) ;
#2230=CARTESIAN_POINT ( 'NONE',  ( -61.73205080756886076, 12.30133545031537068, 0.5000000000000014433 ) ) ;
#2232=CARTESIAN_POINT ( 'NONE',  ( -62.86468353124998032, 11.49479166632526805, 1.000774730468978246 ) ) ;
#2235=CARTESIAN_POINT ( 'NONE',  ( -61.99999999999998579, 16.00000000000000000, 0.5000000000000041078 ) ) ;
#2236=CARTESIAN_POINT ( 'NONE',  ( -60.99999999999998579, 15.27083333333333393, 0.9226497308103762673 ) ) ;
#2240=CARTESIAN_POINT ( 'NONE',  ( -61.99999999999998579, 14.14062499965860020, 0.5015494609379544944 ) ) ;
#2241=CARTESIAN_POINT ( 'NONE',  ( -62.86468353124998032, 10.43229166632526983, 1.000774730468978024 ) ) ;
#2243=( BOUNDED_CURVE ( )  B_SPLINE_CURVE ( 2, ( #8638, #4342, #5817, #9216, #2640, #2753, #305, #6977, #10041 ),
 .UNSPECIFIED., .F., .T. ) 
 B_SPLINE_CURVE_WITH_KNOTS ( ( 3, 2, 2, 2, 3 ),
 ( 0.9296875000000000000, 0.9322916666666666297, 0.9375000000000000000, 0.9427083333333333703, 0.9453125000000000000 ),
 .UNSPECIFIED. ) 
 CURVE ( )  GEOMETRIC_REPRESENTATION_ITEM ( )  RATIONAL_B_SPLINE_CURVE ( ( 0.9330127018922194093, 0.9330127018922194093, 1.000000000000000000, 0.8660254037844387076, 1.000000000000000000, 0.8660254037844387076, 1.000000000000000000, 0.9330127018922194093, 0.9330127018922194093 ) ) 
 REPRESENTATION_ITEM ( '' )  );
#2244=EDGE_LOOP ( 'NONE', ( #7454, #9194, #6845, #916 ) ) ;
#2246=CARTESIAN_POINT ( 'NONE',  ( -62.43234176562498305, 11.22395833299193590, 0.7511620957034662593 ) ) ;
#2249=CARTESIAN_POINT ( 'NONE',  ( -61.99999999999998579, 15.28124999931720218, 0.3452994616207497591 ) ) ;
#2251=VERTEX_POINT ( 'NONE', #2864 ) ;
#2253=CARTESIAN_POINT ( 'NONE',  ( -60.99999999999998579, 15.21874999931720218, 1.500000000000002220 ) ) ;
#2255=CARTESIAN_POINT ( 'NONE',  ( -62.43234176562499016, 14.49479166632526983, 2.248837904296538071 ) ) ;
#2256=CARTESIAN_POINT ( 'NONE',  ( -61.13531646874998415, 9.848958332991934128, 1.000774730468978468 ) ) ;
#2259=CARTESIAN_POINT ( 'NONE',  ( -61.99999999999998579, 14.18749999999999822, 2.654700538379254571 ) ) ;
#2260=DIRECTION ( 'NONE',  ( 0.000000000000000000, 0.000000000000000000, -1.000000000000000000 ) ) ;
#2261=CARTESIAN_POINT ( 'NONE',  ( -60.99999999999998579, 11.96874999931720218, 1.500000000000002220 ) ) ;
#2262=ADVANCED_FACE ( 'NONE', ( #7082 ), #360, .T. ) ;
#2264=CARTESIAN_POINT ( 'NONE',  ( -62.86468353124998032, 13.18229166632526805, 1.000774730468978246 ) ) ;
#2268=CARTESIAN_POINT ( 'NONE',  ( -62.43234176562499016, 11.80729166632526805, 2.248837904296538071 ) ) ;
#2269=LINE ( 'NONE', #7383, #8310 ) ;
#2272=CARTESIAN_POINT ( 'NONE',  ( -62.43234176562498305, 15.72395833299193590, 0.7511620957034662593 ) ) ;
#2274=CARTESIAN_POINT ( 'NONE',  ( -61.99999999999998579, 11.78124999931720218, 0.5000000000000013323 ) ) ;
#2276=ORIENTED_EDGE ( 'NONE', *, *, #9119, .T. ) ;
#2277=CARTESIAN_POINT ( 'NONE',  ( -61.99999999999998579, 9.906249999317202182, 2.500000000000002665 ) ) ;
#2278=CARTESIAN_POINT ( 'NONE',  ( -60.99999999999998579, 9.750000000000000000, 1.500000000000002220 ) ) ;
#2280=CARTESIAN_POINT ( 'NONE',  ( -61.73205080756886076, 14.91741454900183150, 2.500000000000003109 ) ) ;
#2281=CARTESIAN_POINT ( 'NONE',  ( -62.99999999999998579, 14.84374999931720218, 1.500000000000001998 ) ) ;
#2282=CARTESIAN_POINT ( 'NONE',  ( -62.99999999999998579, 15.84374999931720218, 1.500000000000001998 ) ) ;
#2284=CARTESIAN_POINT ( 'NONE',  ( -62.86468353124999453, 11.76562499965860198, 1.500000000000002220 ) ) ;
#2285=CARTESIAN_POINT ( 'NONE',  ( -62.99999999999998579, 14.61458333265053611, 2.077350269189627952 ) ) ;
#2288=DIRECTION ( 'NONE',  ( 0.000000000000000000, 0.000000000000000000, -1.000000000000000000 ) ) ;
#2293=CARTESIAN_POINT ( 'NONE',  ( -61.13531646874998415, 13.32812499965860020, 1.500000000000002220 ) ) ;
#2294=CARTESIAN_POINT ( 'NONE',  ( -62.86468353124999453, 10.45312499965860198, 1.500000000000002220 ) ) ;
#2295=CARTESIAN_POINT ( 'NONE',  ( -60.99999999999998579, 14.52083333333333393, 0.9226497308103762673 ) ) ;
#2296=CARTESIAN_POINT ( 'NONE',  ( -61.56765823437498852, 11.09895833299193590, 2.248837904296538515 ) ) ;
#2297=CARTESIAN_POINT ( 'NONE',  ( -61.56765823437498142, 15.43229166632526805, 0.7511620957034663704 ) ) ;
#2299=AXIS2_PLACEMENT_3D ( 'NONE', #10134, #84, #3415 ) ;
#2302=CARTESIAN_POINT ( 'NONE',  ( -61.13531646874998415, 8.369791666325268054, 1.999225269531026417 ) ) ;
#2303=CARTESIAN_POINT ( 'NONE',  ( -61.99999999999997868, 10.31250000000000000, 0.5000000000000013323 ) ) ;
#2304=ORIENTED_EDGE ( 'NONE', *, *, #4899, .T. ) ;
#2307=AXIS2_PLACEMENT_3D ( 'NONE', #5193, #3646, #1706 ) ;
#2308=( BOUNDED_CURVE ( )  B_SPLINE_CURVE ( 2, ( #4623, #9737, #2911, #9797, #3797, #3671, #8966, #8022, #3020 ),
 .UNSPECIFIED., .F., .T. ) 
 B_SPLINE_CURVE_WITH_KNOTS ( ( 3, 2, 2, 2, 3 ),
 ( 0.2578125000000000000, 0.2604166666666666852, 0.2656250000000000000, 0.2708333333333333148, 0.2734375000000000000 ),
 .UNSPECIFIED. ) 
 CURVE ( )  GEOMETRIC_REPRESENTATION_ITEM ( )  RATIONAL_B_SPLINE_CURVE ( ( 0.9330127018922194093, 0.9330127018922194093, 1.000000000000000000, 0.8660254037844387076, 1.000000000000000000, 0.8660254037844387076, 1.000000000000000000, 0.9330127018922194093, 0.9330127018922194093 ) ) 
 REPRESENTATION_ITEM ( '' )  );
#2309=CARTESIAN_POINT ( 'NONE',  ( -61.13531646874998415, 13.57812499965860198, 1.500000000000002220 ) ) ;
#2310=CARTESIAN_POINT ( 'NONE',  ( -62.86468353124998032, 9.432291666325268054, 1.000774730468978246 ) ) ;
#2312=ORIENTED_EDGE ( 'NONE', *, *, #5271, .F. ) ;
#2313=CARTESIAN_POINT ( 'NONE',  ( -61.49999999999998579, 13.95833333333333215, 2.366025403784441927 ) ) ;
#2315=CARTESIAN_POINT ( 'NONE',  ( -61.99999999999998579, 12.15624999931720396, 2.654700538379254571 ) ) ;
#2316=EDGE_CURVE ( 'NONE', #1066, #6626, #8807, .T. ) ;
#2317=CARTESIAN_POINT ( 'NONE',  ( -61.13531646874998415, 13.82812499965860198, 1.500000000000002220 ) ) ;
#2320=CARTESIAN_POINT ( 'NONE',  ( -62.86468353124998032, 10.99479166632526628, 1.000774730468978246 ) ) ;
#2322=CARTESIAN_POINT ( 'NONE',  ( -61.56765823437498142, 15.93229166632526628, 0.7511620957034663704 ) ) ;
#2324=EDGE_CURVE ( 'NONE', #8781, #10687, #6561, .T. ) ;
#2325=CYLINDRICAL_SURFACE ( 'NONE', #879, 0.9999999999999981126 ) ;
#2326=ORIENTED_EDGE ( 'NONE', *, *, #4725, .T. ) ;
#2327=CARTESIAN_POINT ( 'NONE',  ( -61.99999999999997868, 9.781249999317202182, 0.5000000000000013323 ) ) ;
#2329=CARTESIAN_POINT ( 'NONE',  ( -61.49999999999998579, 9.791666666666667851, 0.6339745962155628467 ) ) ;
#2331=CARTESIAN_POINT ( 'NONE',  ( -61.99999999999998579, 11.68749999999999822, 2.500000000000002665 ) ) ;
#2332=CARTESIAN_POINT ( 'NONE',  ( -61.73205080756886787, 8.301335450315370679, 0.5000000000000002220 ) ) ;
#2334=CARTESIAN_POINT ( 'NONE',  ( -62.86468353124998742, 12.28645833299193413, 1.999225269531025972 ) ) ;
#2336=ORIENTED_EDGE ( 'NONE', *, *, #2709, .T. ) ;
#2338=ORIENTED_EDGE ( 'NONE', *, *, #3145, .F. ) ;
#2339=CYLINDRICAL_SURFACE ( 'NONE', #1999, 0.9999999999999981126 ) ;
#2340=CARTESIAN_POINT ( 'NONE',  ( -62.86468353124999453, 13.70312499965860198, 1.500000000000002220 ) ) ;
#2342=DIRECTION ( 'NONE',  ( 0.000000000000000000, 0.000000000000000000, -1.000000000000000000 ) ) ;
#2344=CARTESIAN_POINT ( 'NONE',  ( -62.86468353124998032, 11.74479166632526628, 1.000774730468978024 ) ) ;
#2345=CARTESIAN_POINT ( 'NONE',  ( -62.86468353124998032, 15.49479166632526628, 1.000774730468978246 ) ) ;
#2348=CARTESIAN_POINT ( 'NONE',  ( -60.99999999999998579, 15.69791666598386648, 2.077350269189628840 ) ) ;
#2353=VECTOR ( 'NONE', #4603, 1000.000000000000000 ) ;
#2354=EDGE_CURVE ( 'NONE', #2668, #10100, #8829, .T. ) ;
#2355=CARTESIAN_POINT ( 'NONE',  ( -61.99999999999999289, 14.51562499965860020, 2.498450539062049724 ) ) ;
#2356=CARTESIAN_POINT ( 'NONE',  ( -61.99999999999998579, 10.39062499965860020, 0.5015494609379544944 ) ) ;
#2357=CARTESIAN_POINT ( 'NONE',  ( -61.56765823437498852, 16.09895833299193768, 2.248837904296538515 ) ) ;
#2359=VERTEX_POINT ( 'NONE', #4159 ) ;
#2360=CARTESIAN_POINT ( 'NONE',  ( -62.99999999999998579, 14.39583333333333570, 2.077350269189627952 ) ) ;
#2361=CARTESIAN_POINT ( 'NONE',  ( -61.99999999999998579, 11.15624999931720218, 2.500000000000002665 ) ) ;
#2362=( NAMED_UNIT ( * ) SI_UNIT ( $, .STERADIAN. ) SOLID_ANGLE_UNIT ( ) );
#2363=UNCERTAINTY_MEASURE_WITH_UNIT (LENGTH_MEASURE( 1.000000000000000082E-05 ), #1638, 'distance_accuracy_value', 'NONE');
#2365=CARTESIAN_POINT ( 'NONE',  ( -62.99999999999998579, 11.34374999931720218, 1.500000000000001998 ) ) ;
#2367=( BOUNDED_CURVE ( )  B_SPLINE_CURVE ( 2, ( #9224, #9115, #5772, #1607, #8183, #1504, #4153, #4778, #3168 ),
 .UNSPECIFIED., .F., .F. ) 
 B_SPLINE_CURVE_WITH_KNOTS ( ( 3, 2, 2, 2, 3 ),
 ( 0.1015624999999999722, 0.1041666666666666713, 0.1093750000000000000, 0.1145833333333333287, 0.1171875000000000278 ),
 .UNSPECIFIED. ) 
 CURVE ( )  GEOMETRIC_REPRESENTATION_ITEM ( )  RATIONAL_B_SPLINE_CURVE ( ( 0.9330127018922194093, 0.9330127018922186322, 1.000000000000000000, 0.8660254037844387076, 1.000000000000000000, 0.8660254037844387076, 1.000000000000000000, 0.9330127018922186322, 0.9330127018922194093 ) ) 
 REPRESENTATION_ITEM ( '' )  );
#2369=CARTESIAN_POINT ( 'NONE',  ( -61.13531646874998415, 13.59895833299193413, 1.000774730468978468 ) ) ;
#2370=ORIENTED_EDGE ( 'NONE', *, *, #3516, .F. ) ;
#2372=CARTESIAN_POINT ( 'NONE',  ( -62.86468353124998742, 11.53645833299193413, 1.999225269531025972 ) ) ;
#2373=CARTESIAN_POINT ( 'NONE',  ( -61.13531646874998415, 16.11979166632526628, 1.999225269531026417 ) ) ;
#2375=CARTESIAN_POINT ( 'NONE',  ( -61.99999999999998579, 8.937500000000001776, 2.500000000000002665 ) ) ;
#2377=CARTESIAN_POINT ( 'NONE',  ( -62.49999999999998579, 9.885416665983870033, 2.366025403784441483 ) ) ;
#2378=CARTESIAN_POINT ( 'NONE',  ( -60.99999999999998579, 10.00000000000000000, 1.500000000000002220 ) ) ;
#2380=CARTESIAN_POINT ( 'NONE',  ( -61.99999999999998579, 16.00000000000000000, 1.500000000000002220 ) ) ;
#2381=CARTESIAN_POINT ( 'NONE',  ( -62.99999999999998579, 9.343749999317202182, 1.500000000000001998 ) ) ;
#2382=CARTESIAN_POINT ( 'NONE',  ( -62.43234176562498305, 11.47395833299193590, 0.7511620957034662593 ) ) ;
#2384=VERTEX_POINT ( 'NONE', #9281 ) ;
#2388=CARTESIAN_POINT ( 'NONE',  ( -62.86468353124998032, 14.18229166632526983, 1.000774730468978246 ) ) ;
#2389=CARTESIAN_POINT ( 'NONE',  ( -61.99999999999998579, 13.81249999999999822, 0.5000000000000013323 ) ) ;
#2390=CARTESIAN_POINT ( 'NONE',  ( -62.26794919243110371, 8.176335450315370679, 2.500000000000000888 ) ) ;
#2392=CARTESIAN_POINT ( 'NONE',  ( -62.86468353124999453, 13.26562499965860198, 1.500000000000002220 ) ) ;
#2393=CARTESIAN_POINT ( 'NONE',  ( -61.99999999999998579, 15.95312499965860198, 0.5015494609379544944 ) ) ;
#2396=CARTESIAN_POINT ( 'NONE',  ( -62.26794919243111082, 13.64508544963257286, 2.500000000000003109 ) ) ;
#2397=CARTESIAN_POINT ( 'NONE',  ( -60.99999999999998579, 15.71874999931720218, 1.500000000000002220 ) ) ;
#2403=CARTESIAN_POINT ( 'NONE',  ( -61.13531646874997705, 13.59895833299193413, 1.000774730468978468 ) ) ;
#2404=CARTESIAN_POINT ( 'NONE',  ( -62.43234176562498305, 9.411458332991935904, 0.7511620957034662593 ) ) ;
#2405=CARTESIAN_POINT ( 'NONE',  ( -62.43234176562498305, 8.161458332991934128, 0.7511620957034662593 ) ) ;
#2406=CARTESIAN_POINT ( 'NONE',  ( -61.99999999999998579, 16.00000000000000000, 2.500000000000000444 ) ) ;
#2408=CARTESIAN_POINT ( 'NONE',  ( -62.99999999999998579, 13.64583333333333215, 2.077350269189627952 ) ) ;
#2409=CARTESIAN_POINT ( 'NONE',  ( -61.56765823437498852, 9.348958332991935904, 2.248837904296538515 ) ) ;
#2410=CARTESIAN_POINT ( 'NONE',  ( -60.99999999999998579, 11.71874999931720218, 1.500000000000002220 ) ) ;
#2413=CARTESIAN_POINT ( 'NONE',  ( -61.99999999999998579, 13.76562499965860020, 2.498450539062049724 ) ) ;
#2414=CARTESIAN_POINT ( 'NONE',  ( -61.99999999999998579, 16.00000000000000000, 2.500000000000000444 ) ) ;
#2416=ADVANCED_FACE ( 'NONE', ( #10891 ), #5779, .T. ) ;
#2417=CARTESIAN_POINT ( 'NONE',  ( -62.86468353124998742, 11.03645833299193413, 1.999225269531025972 ) ) ;
#2419=EDGE_CURVE ( 'NONE', #3958, #3072, #6057, .T. ) ;
#2423=EDGE_CURVE ( 'NONE', #9337, #5402, #10937, .T. ) ;
#2425=ORIENTED_EDGE ( 'NONE', *, *, #8312, .T. ) ;
#2427=CARTESIAN_POINT ( 'NONE',  ( -62.99999999999998579, 10.87500000000000000, 1.500000000000001998 ) ) ;
#2430=CARTESIAN_POINT ( 'NONE',  ( -61.99999999999998579, 14.90624999931720218, 2.500000000000002665 ) ) ;
#2431=CARTESIAN_POINT ( 'NONE',  ( -61.49999999999998579, 10.42708333265053611, 2.366025403784441927 ) ) ;
#2432=CARTESIAN_POINT ( 'NONE',  ( -62.86468353124998742, 13.78645833299193235, 1.999225269531025972 ) ) ;
#2434=ORIENTED_EDGE ( 'NONE', *, *, #3464, .T. ) ;
#2438=ORIENTED_EDGE ( 'NONE', *, *, #10418, .F. ) ;
#2440=CARTESIAN_POINT ( 'NONE',  ( -61.99999999999998579, 15.14062499965860198, 0.5015494609379544944 ) ) ;
#2443=LINE ( 'NONE', #10688, #10954 ) ;
#2444=CARTESIAN_POINT ( 'NONE',  ( -61.99999999999999289, 12.82812499965860198, 2.498450539062049724 ) ) ;
#2445=VECTOR ( 'NONE', #7190, 1000.000000000000000 ) ;
#2446=CARTESIAN_POINT ( 'NONE',  ( -62.86468353124998032, 15.24479166632526805, 1.000774730468978246 ) ) ;
#2448=EDGE_CURVE ( 'NONE', #2594, #10259, #8769, .T. ) ;
#2449=CARTESIAN_POINT ( 'NONE',  ( -61.49999999999998579, 13.42708333265053433, 2.366025403784441927 ) ) ;
#2450=CARTESIAN_POINT ( 'NONE',  ( -61.56765823437498852, 9.598958332991934128, 2.248837904296538515 ) ) ;
#2456=( BOUNDED_CURVE ( )  B_SPLINE_CURVE ( 2, ( #3426, #5821, #5197, #926, #9220, #8601, #8385, #6827, #4307 ),
 .UNSPECIFIED., .F., .F. ) 
 B_SPLINE_CURVE_WITH_KNOTS ( ( 3, 2, 2, 2, 3 ),
 ( 0.6953125000000000000, 0.6979166666666666297, 0.7031250000000000000, 0.7083333333333333703, 0.7109375000000000000 ),
 .UNSPECIFIED. ) 
 CURVE ( )  GEOMETRIC_REPRESENTATION_ITEM ( )  RATIONAL_B_SPLINE_CURVE ( ( 0.9330127018922194093, 0.9330127018922194093, 1.000000000000000000, 0.8660254037844387076, 1.000000000000000000, 0.8660254037844387076, 1.000000000000000000, 0.9330127018922194093, 0.9330127018922194093 ) ) 
 REPRESENTATION_ITEM ( '' )  );
#2459=CARTESIAN_POINT ( 'NONE',  ( -61.13531646874997705, 14.05729166632526805, 1.999225269531026417 ) ) ;
#2460=CARTESIAN_POINT ( 'NONE',  ( -62.43234176562498305, 11.16145833299193590, 0.7511620957034662593 ) ) ;
#2461=CARTESIAN_POINT ( 'NONE',  ( -61.56765823437498142, 8.119791666325268054, 0.7511620957034663704 ) ) ;
#2462=AXIS2_PLACEMENT_3D ( 'NONE', #7264, #4891, #10942 ) ;
#2465=CARTESIAN_POINT ( 'NONE',  ( -60.99999999999998579, 13.22916666666666607, 2.077350269189628840 ) ) ;
#2467=CARTESIAN_POINT ( 'NONE',  ( -61.99999999999999289, 8.203124999658601979, 0.5015494609379544944 ) ) ;
#2469=VECTOR ( 'NONE', #2735, 1000.000000000000000 ) ;
#2470=CARTESIAN_POINT ( 'NONE',  ( -60.99999999999998579, 12.44791666598386826, 2.077350269189628840 ) ) ;
#2471=VERTEX_POINT ( 'NONE', #830 ) ;
#2474=CARTESIAN_POINT ( 'NONE',  ( -61.99999999999998579, 13.64062499965860198, 0.5015494609379544944 ) ) ;
#2477=ORIENTED_EDGE ( 'NONE', *, *, #4906, .T. ) ;
#2479=CARTESIAN_POINT ( 'NONE',  ( -62.86468353124998742, 12.28645833299193413, 1.999225269531025972 ) ) ;
#2480=CARTESIAN_POINT ( 'NONE',  ( -61.99999999999998579, 16.15624999931720041, 2.500000000000002665 ) ) ;
#2489=CARTESIAN_POINT ( 'NONE',  ( -61.49999999999998579, 10.45833333333333393, 2.366025403784441927 ) ) ;
#2491=CARTESIAN_POINT ( 'NONE',  ( -62.86468353124998742, 8.536458332991934128, 1.999225269531025972 ) ) ;
#2493=CARTESIAN_POINT ( 'NONE',  ( -62.86468353124998742, 13.53645833299193413, 1.999225269531025972 ) ) ;
#2496=CARTESIAN_POINT ( 'NONE',  ( -61.99999999999998579, 9.312500000000000000, 0.5000000000000013323 ) ) ;
#2497=EDGE_LOOP ( 'NONE', ( #2139, #10675, #9720 ) ) ;
#2498=DIRECTION ( 'NONE',  ( 0.000000000000000000, 0.000000000000000000, -1.000000000000000000 ) ) ;
#2499=CARTESIAN_POINT ( 'NONE',  ( -61.13531646874998415, 14.57812499965860020, 1.500000000000002220 ) ) ;
#2500=CARTESIAN_POINT ( 'NONE',  ( -62.49999999999998579, 11.83333333333333215, 0.6339745962155627357 ) ) ;
#2503=CARTESIAN_POINT ( 'NONE',  ( -61.99999999999999289, 13.32812499965860020, 2.498450539062049724 ) ) ;
#2505=CARTESIAN_POINT ( 'NONE',  ( -61.13531646874998415, 15.91145833299193590, 1.000774730468978468 ) ) ;
#2506=DIRECTION ( 'NONE',  ( 0.000000000000000000, 0.000000000000000000, -1.000000000000000000 ) ) ;
#2509=CARTESIAN_POINT ( 'NONE',  ( -61.56765823437498852, 8.848958332991934128, 2.248837904296538515 ) ) ;
#2515=CARTESIAN_POINT ( 'NONE',  ( -61.56765823437498852, 15.03645833299193590, 2.248837904296538515 ) ) ;
#2516=CARTESIAN_POINT ( 'NONE',  ( -61.13531646874998415, 11.09895833299193413, 1.000774730468978468 ) ) ;
#2517=CARTESIAN_POINT ( 'NONE',  ( -61.56765823437498142, 15.68229166632526628, 0.7511620957034663704 ) ) ;
#2520=CARTESIAN_POINT ( 'NONE',  ( -61.99999999999998579, 14.81250000000000000, 0.3452994616207497591 ) ) ;
#2521=CARTESIAN_POINT ( 'NONE',  ( -62.43234176562499016, 8.807291666325268054, 2.248837904296538071 ) ) ;
#2522=CARTESIAN_POINT ( 'NONE',  ( -61.99999999999998579, 13.40624999931720041, 2.654700538379254571 ) ) ;
#2523=ORIENTED_EDGE ( 'NONE', *, *, #10862, .T. ) ;
#2524=( BOUNDED_CURVE ( )  B_SPLINE_CURVE ( 2, ( #2160, #3148, #491, #4647, #9042, #1433, #550, #6546, #10653 ),
 .UNSPECIFIED., .F., .F. ) 
 B_SPLINE_CURVE_WITH_KNOTS ( ( 3, 2, 2, 2, 3 ),
 ( 0.8515625000000000000, 0.8541666666666666297, 0.8593750000000000000, 0.8645833333333333703, 0.8671875000000000000 ),
 .UNSPECIFIED. ) 
 CURVE ( )  GEOMETRIC_REPRESENTATION_ITEM ( )  RATIONAL_B_SPLINE_CURVE ( ( 0.9330127018922194093, 0.9330127018922194093, 1.000000000000000000, 0.8660254037844387076, 1.000000000000000000, 0.8660254037844387076, 1.000000000000000000, 0.9330127018922194093, 0.9330127018922194093 ) ) 
 REPRESENTATION_ITEM ( '' )  );
#2526=VECTOR ( 'NONE', #9527, 1000.000000000000000 ) ;
#2528=CARTESIAN_POINT ( 'NONE',  ( -62.86468353124998742, 13.47395833299193413, 1.999225269531025972 ) ) ;
#2533=CARTESIAN_POINT ( 'NONE',  ( -61.13531646874998415, 13.11979166632526805, 1.999225269531026417 ) ) ;
#2534=DIRECTION ( 'NONE',  ( -0.000000000000000000, -1.000000000000000000, -0.000000000000000000 ) ) ;
#2539=CARTESIAN_POINT ( 'NONE',  ( -62.49999999999998579, 12.41666666666666607, 2.366025403784441483 ) ) ;
#2540=EDGE_CURVE ( 'NONE', #4509, #2018, #7211, .T. ) ;
#2542=ORIENTED_EDGE ( 'NONE', *, *, #5180, .F. ) ;
#2543=CARTESIAN_POINT ( 'NONE',  ( -61.99999999999998579, 8.953124999658601979, 0.5015494609379544944 ) ) ;
#2545=AXIS2_PLACEMENT_3D ( 'NONE', #1046, #9609, #5259 ) ;
#2546=CARTESIAN_POINT ( 'NONE',  ( -61.99999999999998579, 13.82812499965860198, 2.498450539062049724 ) ) ;
#2551=ORIENTED_EDGE ( 'NONE', *, *, #466, .T. ) ;
#2552=CARTESIAN_POINT ( 'NONE',  ( -61.99999999999997868, 11.65624999931720218, 2.500000000000002665 ) ) ;
#2553=CARTESIAN_POINT ( 'NONE',  ( -62.86468353124998032, 15.68229166632526628, 1.000774730468978246 ) ) ;
#2554=CARTESIAN_POINT ( 'NONE',  ( -60.99999999999998579, 13.77083333333333215, 0.9226497308103762673 ) ) ;
#2555=CARTESIAN_POINT ( 'NONE',  ( -61.99999999999998579, 12.56249999999999822, 0.5000000000000013323 ) ) ;
#2557=CARTESIAN_POINT ( 'NONE',  ( -62.43234176562498305, 12.47395833299193413, 0.7511620957034662593 ) ) ;
#2559=CARTESIAN_POINT ( 'NONE',  ( -62.43234176562498305, 8.411458332991934128, 0.7511620957034662593 ) ) ;
#2562=CARTESIAN_POINT ( 'NONE',  ( -61.13531646874998415, 8.890624999658601979, 1.500000000000002220 ) ) ;
#2564=ORIENTED_EDGE ( 'NONE', *, *, #7874, .F. ) ;
#2565=LINE ( 'NONE', #10273, #6018 ) ;
#2567=ADVANCED_FACE ( 'NONE', ( #104 ), #3489, .T. ) ;
#2568=CARTESIAN_POINT ( 'NONE',  ( -62.86468353124999453, 15.47395833299193590, 1.999225269531025750 ) ) ;
#2569=CARTESIAN_POINT ( 'NONE',  ( -61.56765823437498142, 10.86979166632526805, 0.7511620957034663704 ) ) ;
#2570=CARTESIAN_POINT ( 'NONE',  ( -61.99999999999999289, 15.70312499965860198, 0.5015494609379544944 ) ) ;
#2573=CARTESIAN_POINT ( 'NONE',  ( -61.49999999999998579, 14.54166666666666607, 0.6339745962155628467 ) ) ;
#2574=CARTESIAN_POINT ( 'NONE',  ( -61.13531646874998415, 9.140624999658601979, 1.500000000000002220 ) ) ;
#2575=CARTESIAN_POINT ( 'NONE',  ( -60.99999999999998579, 12.73958333265053611, 0.9226497308103762673 ) ) ;
#2576=CARTESIAN_POINT ( 'NONE',  ( -62.99999999999998579, 14.64583333333333393, 2.077350269189627952 ) ) ;
#2577=EDGE_LOOP ( 'NONE', ( #3816, #3576, #2818, #10901 ) ) ;
#2579=CARTESIAN_POINT ( 'NONE',  ( -61.56765823437498852, 12.03645833299193413, 2.248837904296538515 ) ) ;
#2581=VERTEX_POINT ( 'NONE', #2003 ) ;
#2582=LINE ( 'NONE', #7392, #1491 ) ;
#2583=CARTESIAN_POINT ( 'NONE',  ( -61.13531646874998415, 12.36979166632526628, 1.999225269531026417 ) ) ;
#2584=( BOUNDED_CURVE ( )  B_SPLINE_CURVE ( 2, ( #3846, #2908, #8737, #5505, #7236, #7961, #7013, #1176, #7183 ),
 .UNSPECIFIED., .F., .T. ) 
 B_SPLINE_CURVE_WITH_KNOTS ( ( 3, 2, 2, 2, 3 ),
 ( 0.7109375000000000000, 0.7135416666666666297, 0.7187500000000000000, 0.7239583333333333703, 0.7265625000000000000 ),
 .UNSPECIFIED. ) 
 CURVE ( )  GEOMETRIC_REPRESENTATION_ITEM ( )  RATIONAL_B_SPLINE_CURVE ( ( 0.9330127018922194093, 0.9330127018922194093, 1.000000000000000000, 0.8660254037844387076, 1.000000000000000000, 0.8660254037844387076, 1.000000000000000000, 0.9330127018922194093, 0.9330127018922194093 ) ) 
 REPRESENTATION_ITEM ( '' )  );
#2585=CYLINDRICAL_SURFACE ( 'NONE', #5657, 0.9999999999999981126 ) ;
#2586=CARTESIAN_POINT ( 'NONE',  ( -60.99999999999998579, 8.947916665983870033, 2.077350269189628840 ) ) ;
#2588=ORIENTED_EDGE ( 'NONE', *, *, #8038, .F. ) ;
#2590=ORIENTED_EDGE ( 'NONE', *, *, #7696, .T. ) ;
#2592=ADVANCED_FACE ( 'NONE', ( #4491 ), #9437, .T. ) ;
#2593=CARTESIAN_POINT ( 'NONE',  ( -61.13531646874998415, 11.84895833299193413, 1.000774730468978468 ) ) ;
#2594=VERTEX_POINT ( 'NONE', #219 ) ;
#2595=CARTESIAN_POINT ( 'NONE',  ( -61.56765823437498142, 8.432291666325268054, 0.7511620957034663704 ) ) ;
#2596=CARTESIAN_POINT ( 'NONE',  ( -60.99999999999998579, 10.46874999931720218, 1.500000000000002220 ) ) ;
#2597=EDGE_CURVE ( 'NONE', #5311, #3891, #7688, .T. ) ;
#2599=CARTESIAN_POINT ( 'NONE',  ( -61.13531646874998415, 12.64062499965860198, 1.500000000000002220 ) ) ;
#2600=CARTESIAN_POINT ( 'NONE',  ( -62.49999999999998579, 12.80208333265053611, 0.6339745962155627357 ) ) ;
#2601=ORIENTED_EDGE ( 'NONE', *, *, #2540, .T. ) ;
#2603=ORIENTED_EDGE ( 'NONE', *, *, #3545, .F. ) ;
#2604=DIRECTION ( 'NONE',  ( -0.000000000000000000, -1.000000000000000000, -0.000000000000000000 ) ) ;
#2605=CARTESIAN_POINT ( 'NONE',  ( -61.99999999999998579, 15.64062499965860198, 0.5015494609379544944 ) ) ;
#2607=CARTESIAN_POINT ( 'NONE',  ( -61.99999999999998579, 12.53124999931720396, 0.5000000000000013323 ) ) ;
#2608=CARTESIAN_POINT ( 'NONE',  ( -62.99999999999998579, 12.36458333265053611, 2.077350269189627952 ) ) ;
#2609=CARTESIAN_POINT ( 'NONE',  ( -61.56765823437498852, 14.59895833299193413, 2.248837904296538515 ) ) ;
#2610=CARTESIAN_POINT ( 'NONE',  ( -61.13531646874998415, 8.828124999658601979, 1.500000000000002220 ) ) ;
#2611=DIRECTION ( 'NONE',  ( -0.000000000000000000, -1.000000000000000000, -0.000000000000000000 ) ) ;
#2614=CARTESIAN_POINT ( 'NONE',  ( -61.56765823437498852, 9.348958332991935904, 2.248837904296538515 ) ) ;
#2615=CYLINDRICAL_SURFACE ( 'NONE', #1990, 0.9999999999999981126 ) ;
#2618=CARTESIAN_POINT ( 'NONE',  ( -60.99999999999998579, 12.94791666598386826, 2.077350269189628840 ) ) ;
#2620=CARTESIAN_POINT ( 'NONE',  ( -61.13531646874997705, 15.55729166632526272, 1.999225269531026417 ) ) ;
#2621=CARTESIAN_POINT ( 'NONE',  ( -62.43234176562498305, 10.91145833299193413, 0.7511620957034662593 ) ) ;
#2622=ADVANCED_FACE ( 'NONE', ( #5207 ), #2841, .T. ) ;
#2623=CARTESIAN_POINT ( 'NONE',  ( -61.13531646874998415, 9.328124999658600203, 1.500000000000002220 ) ) ;
#2624=CARTESIAN_POINT ( 'NONE',  ( -61.99999999999998579, 13.15624999931720218, 2.500000000000002665 ) ) ;
#2626=CARTESIAN_POINT ( 'NONE',  ( -62.99999999999998579, 15.39583333333333570, 2.077350269189627952 ) ) ;
#2628=CARTESIAN_POINT ( 'NONE',  ( -62.43234176562499016, 8.557291666325268054, 2.248837904296538071 ) ) ;
#2630=AXIS2_PLACEMENT_3D ( 'NONE', #6401, #3064, #5609 ) ;
#2632=CARTESIAN_POINT ( 'NONE',  ( -62.49999999999998579, 13.38541666598387003, 2.366025403784441483 ) ) ;
#2633=CARTESIAN_POINT ( 'NONE',  ( -62.49999999999998579, 14.66666666666666607, 2.366025403784441483 ) ) ;
#2635=CARTESIAN_POINT ( 'NONE',  ( -62.99999999999998579, 11.62500000000000000, 1.500000000000001998 ) ) ;
#2637=VECTOR ( 'NONE', #5500, 1000.000000000000000 ) ;
#2638=CARTESIAN_POINT ( 'NONE',  ( -61.56765823437498852, 11.78645833299193413, 2.248837904296538515 ) ) ;
#2640=CARTESIAN_POINT ( 'NONE',  ( -60.99999999999998579, 15.50000000000000000, 1.500000000000002220 ) ) ;
#2642=CARTESIAN_POINT ( 'NONE',  ( -62.49999999999998579, 12.83333333333333393, 0.6339745962155627357 ) ) ;
#2643=VECTOR ( 'NONE', #7060, 1000.000000000000000 ) ;
#2644=CARTESIAN_POINT ( 'NONE',  ( -62.86468353124999453, 12.26562499965860198, 1.500000000000002220 ) ) ;
#2646=LINE ( 'NONE', #6818, #1221 ) ;
#2648=CARTESIAN_POINT ( 'NONE',  ( -61.49999999999998579, 8.927083332650536107, 2.366025403784441927 ) ) ;
#2654=CARTESIAN_POINT ( 'NONE',  ( -62.99999999999998579, 12.39583333333333393, 2.077350269189627952 ) ) ;
#2656=CARTESIAN_POINT ( 'NONE',  ( -61.99999999999998579, 11.64062499965860198, 0.5015494609379544944 ) ) ;
#2658=CARTESIAN_POINT ( 'NONE',  ( -61.13531646874998415, 9.411458332991934128, 1.000774730468978468 ) ) ;
#2659=CARTESIAN_POINT ( 'NONE',  ( -62.26794919243111082, 15.82366454968462932, 0.5000000000000013323 ) ) ;
#2660=VECTOR ( 'NONE', #7626, 1000.000000000000000 ) ;
#2662=CARTESIAN_POINT ( 'NONE',  ( -61.99999999999998579, 13.32812499965860198, 2.498450539062049724 ) ) ;
#2666=CARTESIAN_POINT ( 'NONE',  ( -61.99999999999998579, 12.31249999999999822, 0.5000000000000013323 ) ) ;
#2668=VERTEX_POINT ( 'NONE', #3437 ) ;
#2669=CARTESIAN_POINT ( 'NONE',  ( -62.49999999999998579, 10.91666666666666607, 2.366025403784441483 ) ) ;
#2670=CARTESIAN_POINT ( 'NONE',  ( -62.86468353124998742, 14.97395833299193590, 1.999225269531025972 ) ) ;
#2671=CARTESIAN_POINT ( 'NONE',  ( -62.49999999999998579, 8.885416665983868256, 2.366025403784441483 ) ) ;
#2674=CARTESIAN_POINT ( 'NONE',  ( -61.56765823437498852, 14.09895833299193413, 2.248837904296538515 ) ) ;
#2675=CARTESIAN_POINT ( 'NONE',  ( -61.13531646874998415, 8.807291666325268054, 1.999225269531026417 ) ) ;
#2678=CARTESIAN_POINT ( 'NONE',  ( -61.99999999999998579, 8.703124999658601979, 0.5015494609379544944 ) ) ;
#2679=CARTESIAN_POINT ( 'NONE',  ( -61.99999999999998579, 15.78124999931720041, 0.5000000000000013323 ) ) ;
#2683=CARTESIAN_POINT ( 'NONE',  ( -61.56765823437498852, 15.53645833299193590, 2.248837904296538515 ) ) ;
#2684=CARTESIAN_POINT ( 'NONE',  ( -62.86468353124998742, 10.72395833299193413, 1.999225269531025972 ) ) ;
#2685=CARTESIAN_POINT ( 'NONE',  ( -62.86468353124999453, 8.703124999658601979, 1.500000000000002220 ) ) ;
#2687=CARTESIAN_POINT ( 'NONE',  ( -61.99999999999998579, 15.56250000000000000, 0.3452994616207497591 ) ) ;
#2688=CARTESIAN_POINT ( 'NONE',  ( -61.56765823437498142, 10.18229166632526805, 0.7511620957034663704 ) ) ;
#2689=CARTESIAN_POINT ( 'NONE',  ( -60.99999999999998579, 13.46874999931720218, 1.500000000000002220 ) ) ;
#2694=CARTESIAN_POINT ( 'NONE',  ( -61.99999999999999289, 12.01562499965860198, 2.498450539062049724 ) ) ;
#2696=CARTESIAN_POINT ( 'NONE',  ( -61.99999999999998579, 16.00000000000000000, 1.500000000000002220 ) ) ;
#2697=ORIENTED_EDGE ( 'NONE', *, *, #7200, .F. ) ;
#2698=CARTESIAN_POINT ( 'NONE',  ( -60.99999999999998579, 11.72916666666666607, 2.077350269189628840 ) ) ;
#2699=DIRECTION ( 'NONE',  ( -0.000000000000000000, -1.000000000000000000, -0.000000000000000000 ) ) ;
#2700=CARTESIAN_POINT ( 'NONE',  ( -61.13531646874998415, 14.89062499965860020, 1.500000000000002220 ) ) ;
#2701=CARTESIAN_POINT ( 'NONE',  ( -61.73205080756886076, 10.30133545031537068, 0.5000000000000044409 ) ) ;
#2702=VECTOR ( 'NONE', #385, 1000.000000000000000 ) ;
#2703=CARTESIAN_POINT ( 'NONE',  ( -62.99999999999998579, 9.322916665983870033, 0.9226497308103756012 ) ) ;
#2704=ORIENTED_EDGE ( 'NONE', *, *, #3929, .F. ) ;
#2708=CARTESIAN_POINT ( 'NONE',  ( -62.43234176562498305, 10.91145833299193413, 0.7511620957034662593 ) ) ;
#2709=EDGE_CURVE ( 'NONE', #5522, #10281, #7118, .T. ) ;
#2713=CARTESIAN_POINT ( 'NONE',  ( -61.99999999999998579, 8.828124999658601979, 2.498450539062049724 ) ) ;
#2716=CARTESIAN_POINT ( 'NONE',  ( -62.86468353124998742, 15.03645833299193590, 1.999225269531025972 ) ) ;
#2720=( BOUNDED_CURVE ( )  B_SPLINE_CURVE ( 2, ( #10047, #9847, #5879, #4427, #6101, #5086, #6882, #5145, #5252 ),
 .UNSPECIFIED., .F., .F. ) 
 B_SPLINE_CURVE_WITH_KNOTS ( ( 3, 2, 2, 2, 3 ),
 ( 0.4765625000000000000, 0.4791666666666666852, 0.4843750000000000000, 0.4895833333333333148, 0.4921875000000000000 ),
 .UNSPECIFIED. ) 
 CURVE ( )  GEOMETRIC_REPRESENTATION_ITEM ( )  RATIONAL_B_SPLINE_CURVE ( ( 0.9330127018922194093, 0.9330127018922194093, 1.000000000000000000, 0.8660254037844387076, 1.000000000000000000, 0.8660254037844387076, 1.000000000000000000, 0.9330127018922194093, 0.9330127018922194093 ) ) 
 REPRESENTATION_ITEM ( '' )  );
#2724=CARTESIAN_POINT ( 'NONE',  ( -61.99999999999998579, 8.687500000000001776, 2.654700538379254571 ) ) ;
#2727=CARTESIAN_POINT ( 'NONE',  ( -62.99999999999998579, 12.34374999931720218, 1.500000000000001998 ) ) ;
#2728=CARTESIAN_POINT ( 'NONE',  ( -61.13531646874997705, 13.86979166632526628, 1.999225269531026417 ) ) ;
#2729=CARTESIAN_POINT ( 'NONE',  ( -61.56765823437498852, 8.786458332991934128, 2.248837904296538515 ) ) ;
#2730=DIRECTION ( 'NONE',  ( 0.000000000000000000, 0.000000000000000000, -1.000000000000000000 ) ) ;
#2731=CARTESIAN_POINT ( 'NONE',  ( -62.49999999999998579, 9.666666666666667851, 2.366025403784441483 ) ) ;
#2732=CARTESIAN_POINT ( 'NONE',  ( -62.86468353124999453, 10.26562499965860198, 1.500000000000002220 ) ) ;
#2733=CARTESIAN_POINT ( 'NONE',  ( -61.99999999999998579, 16.00000000000000000, 1.500000000000002220 ) ) ;
#2735=DIRECTION ( 'NONE',  ( -0.000000000000000000, -1.000000000000000000, -0.000000000000000000 ) ) ;
#2736=FACE_OUTER_BOUND ( 'NONE', #8415, .T. ) ;
#2737=CARTESIAN_POINT ( 'NONE',  ( -61.13531646874997705, 15.34895833299193590, 1.000774730468978468 ) ) ;
#2738=CARTESIAN_POINT ( 'NONE',  ( -61.56765823437498852, 12.78645833299193413, 2.248837904296538515 ) ) ;
#2739=CARTESIAN_POINT ( 'NONE',  ( -62.86468353124998032, 9.182291666325268054, 1.000774730468978024 ) ) ;
#2740=CARTESIAN_POINT ( 'NONE',  ( -62.26794919243111082, 13.04241454900183328, 0.5000000000000013323 ) ) ;
#2742=CARTESIAN_POINT ( 'NONE',  ( -61.99999999999998579, 15.43750000000000000, 2.654700538379254571 ) ) ;
#2743=CARTESIAN_POINT ( 'NONE',  ( -61.99999999999999289, 9.828124999658601979, 2.498450539062049724 ) ) ;
#2744=CARTESIAN_POINT ( 'NONE',  ( -62.86468353124998742, 15.47395833299193413, 1.999225269531025972 ) ) ;
#2745=EDGE_CURVE ( 'NONE', #1260, #6260, #2060, .T. ) ;
#2746=CARTESIAN_POINT ( 'NONE',  ( -61.99999999999998579, 13.28124999931720396, 0.3452994616207497591 ) ) ;
#2750=CARTESIAN_POINT ( 'NONE',  ( -62.43234176562498305, 11.41145833299193590, 0.7511620957034662593 ) ) ;
#2753=CARTESIAN_POINT ( 'NONE',  ( -60.99999999999998579, 15.52083333333333215, 0.9226497308103762673 ) ) ;
#2754=VERTEX_POINT ( 'NONE', #565 ) ;
#2755=CARTESIAN_POINT ( 'NONE',  ( -61.99999999999998579, 10.43750000000000178, 2.654700538379254571 ) ) ;
#2756=CARTESIAN_POINT ( 'NONE',  ( -62.26794919243111082, 10.07366454968462932, 0.5000000000000013323 ) ) ;
#2757=CARTESIAN_POINT ( 'NONE',  ( -61.13531646874998415, 13.61979166632526983, 1.999225269531026417 ) ) ;
#2758=CARTESIAN_POINT ( 'NONE',  ( -61.99999999999998579, 11.06250000000000000, 0.5000000000000013323 ) ) ;
#2759=CARTESIAN_POINT ( 'NONE',  ( -62.49999999999998579, 8.802083332650536107, 0.6339745962155627357 ) ) ;
#2760=ORIENTED_EDGE ( 'NONE', *, *, #10476, .T. ) ;
#2762=CARTESIAN_POINT ( 'NONE',  ( -61.99999999999998579, 10.89062499965860020, 0.5015494609379544944 ) ) ;
#2763=EDGE_CURVE ( 'NONE', #2359, #4541, #1235, .T. ) ;
#2766=EDGE_CURVE ( 'NONE', #1066, #1268, #26, .T. ) ;
#2767=CARTESIAN_POINT ( 'NONE',  ( -61.56765823437498142, 9.932291666325268054, 0.7511620957034663704 ) ) ;
#2770=CARTESIAN_POINT ( 'NONE',  ( -61.13531646874998415, 15.14062499965860020, 1.500000000000002220 ) ) ;
#2771=DIRECTION ( 'NONE',  ( -0.000000000000000000, -1.000000000000000000, -0.000000000000000000 ) ) ;
#2772=ORIENTED_EDGE ( 'NONE', *, *, #10211, .F. ) ;
#2773=CARTESIAN_POINT ( 'NONE',  ( -61.99999999999998579, 16.00000000000000000, 2.500000000000000444 ) ) ;
#2775=CARTESIAN_POINT ( 'NONE',  ( -61.73205080756886076, 12.77008544963256931, 0.5000000000000014433 ) ) ;
#2776=CARTESIAN_POINT ( 'NONE',  ( -60.99999999999998579, 8.979166666666666075, 2.077350269189628840 ) ) ;
#2777=CARTESIAN_POINT ( 'NONE',  ( -62.99999999999998579, 9.895833333333333925, 2.077350269189627952 ) ) ;
#2779=CARTESIAN_POINT ( 'NONE',  ( -61.99999999999998579, 16.00000000000000000, 1.500000000000002220 ) ) ;
#2780=CARTESIAN_POINT ( 'NONE',  ( -61.13531646874997705, 14.61979166632526805, 1.999225269531026417 ) ) ;
#2781=CARTESIAN_POINT ( 'NONE',  ( -61.56765823437498142, 9.369791666325268054, 0.7511620957034663704 ) ) ;
#2783=CARTESIAN_POINT ( 'NONE',  ( -61.99999999999998579, 14.56249999999999822, 0.5000000000000013323 ) ) ;
#2785=CARTESIAN_POINT ( 'NONE',  ( -61.56765823437498852, 10.59895833299193413, 2.248837904296538515 ) ) ;
#2787=ORIENTED_EDGE ( 'NONE', *, *, #175, .T. ) ;
#2789=CARTESIAN_POINT ( 'NONE',  ( -62.99999999999998579, 11.35416666666666607, 0.9226497308103756012 ) ) ;
#2790=LINE ( 'NONE', #1123, #3238 ) ;
#2791=CARTESIAN_POINT ( 'NONE',  ( -61.56765823437498142, 12.36979166632526805, 0.7511620957034663704 ) ) ;
#2792=CARTESIAN_POINT ( 'NONE',  ( -62.43234176562498305, 8.411458332991934128, 0.7511620957034662593 ) ) ;
#2796=CARTESIAN_POINT ( 'NONE',  ( -62.99999999999998579, 10.84374999931720218, 1.500000000000001998 ) ) ;
#2797=CARTESIAN_POINT ( 'NONE',  ( -62.86468353124998032, 10.49479166632526983, 1.000774730468978024 ) ) ;
#2798=AXIS2_PLACEMENT_3D ( 'NONE', #8052, #8213, #603 ) ;
#2800=CARTESIAN_POINT ( 'NONE',  ( -61.99999999999998579, 15.64062499965860198, 0.5015494609379544944 ) ) ;
#2801=CARTESIAN_POINT ( 'NONE',  ( -61.49999999999998579, 14.42708333265053611, 2.366025403784441927 ) ) ;
#2803=ORIENTED_EDGE ( 'NONE', *, *, #3149, .F. ) ;
#2807=CARTESIAN_POINT ( 'NONE',  ( -62.86468353124999453, 11.47395833299193590, 1.999225269531025750 ) ) ;
#2809=CARTESIAN_POINT ( 'NONE',  ( -62.86468353124998742, 8.223958332991934128, 1.999225269531025972 ) ) ;
#2812=CARTESIAN_POINT ( 'NONE',  ( -62.49999999999998579, 12.58333333333333393, 0.6339745962155627357 ) ) ;
#2813=DIRECTION ( 'NONE',  ( -0.000000000000000000, -1.000000000000000000, -0.000000000000000000 ) ) ;
#2814=CARTESIAN_POINT ( 'NONE',  ( -62.86468353124998742, 13.78645833299193235, 1.999225269531025972 ) ) ;
#2815=DIRECTION ( 'NONE',  ( 0.000000000000000000, 0.000000000000000000, -1.000000000000000000 ) ) ;
#2817=CARTESIAN_POINT ( 'NONE',  ( -61.99999999999998579, 10.28124999931720218, 0.3452994616207497591 ) ) ;
#2818=ORIENTED_EDGE ( 'NONE', *, *, #3260, .T. ) ;
#2821=CARTESIAN_POINT ( 'NONE',  ( -61.99999999999998579, 13.31249999999999822, 0.5000000000000013323 ) ) ;
#2822=( BOUNDED_CURVE ( )  B_SPLINE_CURVE ( 2, ( #4759, #444, #3828, #8167, #7218, #557, #3102, #9259, #9309 ),
 .UNSPECIFIED., .F., .F. ) 
 B_SPLINE_CURVE_WITH_KNOTS ( ( 3, 2, 2, 2, 3 ),
 ( 0.5390625000000000000, 0.5416666666666666297, 0.5468750000000000000, 0.5520833333333333703, 0.5546875000000000000 ),
 .UNSPECIFIED. ) 
 CURVE ( )  GEOMETRIC_REPRESENTATION_ITEM ( )  RATIONAL_B_SPLINE_CURVE ( ( 0.9330127018922194093, 0.9330127018922194093, 1.000000000000000000, 0.8660254037844387076, 1.000000000000000000, 0.8660254037844387076, 1.000000000000000000, 0.9330127018922194093, 0.9330127018922194093 ) ) 
 REPRESENTATION_ITEM ( '' )  );
#2823=CARTESIAN_POINT ( 'NONE',  ( -62.86468353124998742, 11.47395833299193590, 1.999225269531025972 ) ) ;
#2828=CARTESIAN_POINT ( 'NONE',  ( -62.43234176562499016, 10.30729166632526983, 2.248837904296538071 ) ) ;
#2832=CARTESIAN_POINT ( 'NONE',  ( -61.99999999999998579, 14.57812499965860198, 2.498450539062049724 ) ) ;
#2835=CARTESIAN_POINT ( 'NONE',  ( -61.99999999999998579, 9.437499999999998224, 2.500000000000002665 ) ) ;
#2838=CARTESIAN_POINT ( 'NONE',  ( -61.99999999999998579, 16.00000000000000000, 1.500000000000002220 ) ) ;
#2839=CARTESIAN_POINT ( 'NONE',  ( -61.99999999999998579, 9.062500000000000000, 0.3452994616207497591 ) ) ;
#2841=CYLINDRICAL_SURFACE ( 'NONE', #9291, 0.9999999999999981126 ) ;
#2843=CARTESIAN_POINT ( 'NONE',  ( -61.73205080756886076, 10.77008544963257286, 0.5000000000000014433 ) ) ;
#2844=CARTESIAN_POINT ( 'NONE',  ( -61.56765823437498142, 13.68229166632526805, 0.7511620957034663704 ) ) ;
#2845=CARTESIAN_POINT ( 'NONE',  ( -61.56765823437498852, 9.786458332991934128, 2.248837904296538515 ) ) ;
#2847=CARTESIAN_POINT ( 'NONE',  ( -61.99999999999998579, 9.953124999658601979, 0.5015494609379544944 ) ) ;
#2849=ORIENTED_EDGE ( 'NONE', *, *, #1281, .F. ) ;
#2851=CARTESIAN_POINT ( 'NONE',  ( -61.99999999999998579, 15.31250000000000000, 0.5000000000000013323 ) ) ;
#2853=CARTESIAN_POINT ( 'NONE',  ( -61.49999999999998579, 15.79166666666666607, 0.6339745962155628467 ) ) ;
#2855=CARTESIAN_POINT ( 'NONE',  ( -61.99999999999998579, 13.01562499965860198, 2.498450539062049724 ) ) ;
#2856=CARTESIAN_POINT ( 'NONE',  ( -61.99999999999999289, 9.015624999658601979, 2.498450539062049724 ) ) ;
#2857=CARTESIAN_POINT ( 'NONE',  ( -62.26794919243110371, 8.573664549684629321, 0.4999999999999990563 ) ) ;
#2859=CARTESIAN_POINT ( 'NONE',  ( -60.99999999999998579, 16.00000000000000000, 1.500000000000002220 ) ) ;
#2860=CARTESIAN_POINT ( 'NONE',  ( -61.56765823437498852, 9.848958332991934128, 2.248837904296538515 ) ) ;
#2862=CARTESIAN_POINT ( 'NONE',  ( -61.99999999999998579, 15.26562499965860020, 2.498450539062049724 ) ) ;
#2863=CARTESIAN_POINT ( 'NONE',  ( -61.49999999999998579, 14.01041666598387003, 0.6339745962155628467 ) ) ;
#2864=CARTESIAN_POINT ( 'NONE',  ( -61.99999999999998579, 8.187500000000001776, 2.500000000000003109 ) ) ;
#2866=CARTESIAN_POINT ( 'NONE',  ( -62.99999999999998579, 11.64583333333333748, 2.077350269189627952 ) ) ;
#2867=ORIENTED_EDGE ( 'NONE', *, *, #2540, .F. ) ;
#2868=CARTESIAN_POINT ( 'NONE',  ( -62.43234176562499016, 12.99479166632526805, 2.248837904296538071 ) ) ;
#2869=CARTESIAN_POINT ( 'NONE',  ( -62.86468353124999453, 8.953124999658601979, 1.500000000000002220 ) ) ;
#2871=ORIENTED_EDGE ( 'NONE', *, *, #2763, .F. ) ;
#2872=CARTESIAN_POINT ( 'NONE',  ( -61.49999999999998579, 12.54166666666666607, 0.6339745962155628467 ) ) ;
#2873=CARTESIAN_POINT ( 'NONE',  ( -61.99999999999998579, 16.00000000000000000, 2.500000000000000444 ) ) ;
#2874=CARTESIAN_POINT ( 'NONE',  ( -61.13531646874998415, 14.86979166632526805, 1.999225269531026417 ) ) ;
#2875=CARTESIAN_POINT ( 'NONE',  ( -61.99999999999997868, 10.31250000000000000, 0.5000000000000013323 ) ) ;
#2876=CARTESIAN_POINT ( 'NONE',  ( -62.99999999999998579, 10.59374999931720396, 1.500000000000001998 ) ) ;
#2877=ORIENTED_EDGE ( 'NONE', *, *, #10783, .T. ) ;
#2878=VECTOR ( 'NONE', #10856, 1000.000000000000000 ) ;
#2881=CARTESIAN_POINT ( 'NONE',  ( -61.13531646874998415, 12.32812499965860198, 1.500000000000002220 ) ) ;
#2883=ORIENTED_EDGE ( 'NONE', *, *, #3905, .T. ) ;
#2885=CARTESIAN_POINT ( 'NONE',  ( -62.86468353124999453, 10.76562499965860020, 1.500000000000002220 ) ) ;
#2886=FACE_OUTER_BOUND ( 'NONE', #10491, .T. ) ;
#2888=CARTESIAN_POINT ( 'NONE',  ( -61.56765823437498142, 14.18229166632526805, 0.7511620957034663704 ) ) ;
#2889=DIRECTION ( 'NONE',  ( 0.000000000000000000, 0.000000000000000000, -1.000000000000000000 ) ) ;
#2890=ORIENTED_EDGE ( 'NONE', *, *, #4244, .F. ) ;
#2891=( BOUNDED_SURFACE ( )  B_SPLINE_SURFACE ( 1, 2, ( 
 ( #4823, #619, #3163, #5713, #4044, #7446, #5035, #10928, #4199, #3479, #4252, #10093, #7657, #151, #2595, #6717, #3318, #6877, #10144, #2491, #871, #10251, #9772, #7548, #6826, #819, #1767, #42, #6041, #6936, #7603, #7714, #9427, #2713, #7769, #10311, #9317, #1710, #6098, #2543, #9483, #3425, #5196, #10198, #94, #5980, #5875, #5141, #1880, #1823, #5248, #9269, #8652, #8487, #978, #8600, #4356, #9371, #5083, #3371, #3536, #2658, #8544, #925, #4306, #4150, #1662, #8434, #6773, #5932, #10546, #7999, #3707, #1094, #2166, #6217, #1034, #6330, #2942, #9659, #6387, #1991, #4481, #7887, #9713, #3827, #2767, #2050, #3593, #6992, #1155, #5364, #265, #4535, #4652, #6154, #382, #1274, #3648, #321, #5423, #1933, #9598, #10596, #2828, #8890, #5306, #2997, #4421, #10370, #5481, #1212, #8828, #9775, #7045, #8716, #8058, #9539, #4595, #7107, #10425, #7824, #443, #8775, #7939, #10487, #2885, #6272, #7216, #3769, #7162, #2105, #5541, #207, #1382, #1489, #10034, #2320, #3883, #2417, #5650, #7326, #10718, #3153, #5701, #5758, #5598, #3101, #6449, #4089, #9100, #4865, #8944, #8993, #1336, #9046, #9881, #9988, #6659, #652, #9152, #4705, #7275, #2372, #8269, #4031, #8111, #4758, #2219, #4916, #10660, #7436, #3989, #8166, #496, #1538, #2268, #556, #3051, #3934, #6553, #8315, #9828, #6499, #1437, #10816, #9936, #4813, #3204, #8220, #6607, #608, #7382, #10762, #708, #7486, #10869, #3258, #2644, #2479, #4187, #3308, #969, #2583, #10187, #5808, #5866, #9206, #5922, #6760, #6865, #3526, #8533, #6031, #1592, #9415, #8590, #10971, #3360, #4345, #809, #7757, #5074, #10238, #8475, #9357, #7647, #4142, #3414, #136, #7703, #6926, #4972, #10298, #10133, #1809, #5181, #8373, #1700, #2533, #5026, #82, #912, #9308, #5969, #1754, #3468, #31, #7539, #760, #10918, #4294, #5128, #860, #9258, #6705, #4242, #10082, #1651, #8426, #6817, #7589, #3638, #2757, #9528, #1200, #5468, #4407, #3694, #5238, #8642, #2814, #7035, #1921, #6201, #6319, #7816, #9650, #2934, #6142, #1980, #309, #3580, #7875, #1264, #4469, #10535, #6982, #4643, #6086, #1022, #9473, #2039, #8706, #195, #10413, #5413, #5295, #1867, #5350, #10360, #7096, #9588, #4580, #8877, #1081, #6263, #7988, #8045, #254, #10474, #8817, #373, #8764, #1144, #7153, #582, #9703, #3756, #7929, #2095, #3967, #7356, #2874, #2700, #4526, #10941, #4947, #6527, #784, #733, #6734, #7464, #9177, #633, #1677, #4890, #8292, #679, #9964, #1619, #2446, #7408, #7564, #4116, #4012, #833, #4841, #10057, #10842, #2297, #5838, #5783, #2345, #9236, #3286, #3330, #10790, #5734, #9910, #4214, #4163, #8350, #5683, #3179, #4062, #6585, #5049, #4998, #8449, #10108, #3227, #9128, #2505, #6634, #2393, #10011, #1515, #10744, #8400, #9076, #3131, #7513, #6681, #10896 ),
 ( #1564, #1467, #5894, #8249, #9285, #6112, #5211, #1950, #8561, #7676, #3441, #9497, #10385, #9332, #8615, #10161, #2559, #7730, #941, #6839, #109, #225, #10210, #1893, #10329, #4266, #4438, #993, #887, #8730, #1724, #6949, #4321, #5945, #2729, #2675, #2610, #5263, #167, #3610, #8504, #5998, #6791, #1115, #8669, #1840, #5099, #58, #3493, #9387, #9557, #1050, #5319, #7007, #6896, #1782, #7839, #10267, #6055, #9443, #5154, #7619, #2781, #4373, #4, #7785, #3552, #6169, #3384, #4495, #6232, #10442, #1229, #5498, #10611, #2064, #9673, #7176, #2121, #278, #8958, #8074, #2845, #2177, #3663, #8902, #456, #3010, #2009, #4610, #2901, #8014, #5382, #7059, #1169, #1289, #5437, #9613, #8842, #9788, #398, #8788, #4548, #4667, #3725, #7954, #3786, #3840, #336, #7122, #10559, #10502, #2956, #6341, #7231, #5560, #6288, #9727, #6402, #1349, #4717, #8124, #7900, #1930, #920, #9479, #7883, #6213, #262, #5303, #8650, #8714, #9595, #10367, #4418, #2762, #2708, #3645, #1031, #10195, #4478, #7822, #10420, #147, #1875, #4303, #5360, #8597, #976, #4354, #6150, #6095, #3477, #4532, #7765, #3422, #1089, #7041, #203, #8772, #3532, #6874, #10247, #2823, #1988, #5137, #3589, #5977, #9367, #6934, #10307, #2656, #5245, #1151, #8541, #9535, #7937, #6038, #6989, #6824, #7711, #2593, #1764, #5191, #92, #9422, #1820, #3702, #6270, #4754, #493, #4703, #9043, #7159, #4589, #7321, #9656, #8109, #6381, #7995, #7104, #552, #1270, #379, #2881, #2940, #5536, #10713, #2048, #5419, #3765, #3879, #8941, #10542, #7270, #1435, #10655, #8824, #4809, #8055, #9710, #2102, #1333, #3048, #8162, #6327, #5476, #1209, #6496, #6442, #9825, #315, #8884, #10484, #440, #4648, #1379, #3825, #2216, #3931, #7213, #3099, #9878, #10593, #2993, #2264, #9770, #5647, #2161, #5595, #8989, #755, #10031, #6547, #5804, #6756, #10077, #10128, #3986, #2528, #1534, #5023, #9255, #1645, #4086, #2369, #7431, #2474, #3306, #8311, #4969, #8369, #5861, #2413, #9932, #4182, #2317, #6701, #4028, #605, #10864, #4863, #9202, #4913, #8422, #10965, #649, #4139, #806, #5917, #10810, #1586, #7586, #3354, #5699, #3255, #9304, #1696, #8214, #7379, #7536, #10758, #3150, #10914, #9094, #1487, #7483, #8266, #3201, #6604, #9983, #5755, #9148, #704, #6654, #8921, #3627, #3806, #5338, #8805, #357, #421, #241, #1968, #1069, #9747, #3744, #7974, #3567, #7022, #6967, #3680, #4513, #4629, #1310, #6307, #7196, #10347, #10577, #6359, #8750, #1131, #2142, #9574, #5517, #2862, #8031, #6249, #7141, #5399, #1910, #1187, #4685, #5455, #8092, #2744, #6131, #7916, #2973, #9514, #5281, #10460, #296, #2800, #8862, #9689, #7080, #10521, #2920, #1249, #4566, #8690, #4457, #7859, #2082, #10401, #9634, #6188, #2027, #5627, #475, #5736, #9965, #9078, #5786 ) ),
 .UNSPECIFIED., .F., .F., .F. ) 
 B_SPLINE_SURFACE_WITH_KNOTS ( ( 2, 2 ),
 ( 3, 2, 2, 2, 2, 2, 2, 2, 2, 2, 2, 2, 2, 2, 2, 2, 2, 2, 2, 2, 2, 2, 2, 2, 2, 2, 2, 2, 2, 2, 2, 2, 2, 2, 2, 2, 2, 2, 2, 2, 2, 2, 2, 2, 2, 2, 2, 2, 2, 2, 2, 2, 2, 2, 2, 2, 2, 2, 2, 2, 2, 2, 2, 2, 2, 2, 2, 2, 2, 2, 2, 2, 2, 2, 2, 2, 2, 2, 2, 2, 2, 2, 2, 2, 2, 2, 2, 2, 2, 2, 2, 2, 2, 2, 2, 2, 2, 2, 2, 2, 2, 2, 2, 2, 2, 2, 2, 2, 2, 2, 2, 2, 2, 2, 2, 2, 2, 2, 2, 2, 2, 2, 2, 2, 2, 2, 2, 2, 2, 2, 2, 2, 2, 2, 2, 2, 2, 2, 2, 2, 2, 2, 2, 2, 2, 2, 2, 2, 2, 2, 2, 2, 2, 2, 2, 2, 2, 2, 2, 2, 2, 2, 2, 2, 2, 2, 2, 2, 2, 2, 2, 2, 2, 2, 2, 2, 2, 2, 2, 2, 2, 2, 2, 2, 2, 2, 2, 2, 2, 2, 2, 2, 3 ),
 ( 0.000000000000000000, 1.000000000000000000 ),
 ( 0.000000000000000000, 0.005208333333333333044, 0.01041666666666666609, 0.01562500000000000000, 0.02083333333333333218, 0.02604166666666666782, 0.03125000000000000000, 0.03645833333333333565, 0.04166666666666666435, 0.04687500000000000000, 0.05208333333333333565, 0.05729166666666666435, 0.06250000000000000000, 0.06770833333333332871, 0.07291666666666667129, 0.07812500000000000000, 0.08333333333333332871, 0.08854166666666667129, 0.09375000000000000000, 0.09895833333333332871, 0.1041666666666666713, 0.1093750000000000000, 0.1145833333333333287, 0.1197916666666666713, 0.1250000000000000000, 0.1302083333333333426, 0.1354166666666666574, 0.1406250000000000000, 0.1458333333333333426, 0.1510416666666666574, 0.1562500000000000000, 0.1614583333333333426, 0.1666666666666666574, 0.1718750000000000000, 0.1770833333333333426, 0.1822916666666666574, 0.1875000000000000000, 0.1927083333333333426, 0.1979166666666666574, 0.2031250000000000000, 0.2083333333333333426, 0.2135416666666666574, 0.2187500000000000000, 0.2239583333333333426, 0.2291666666666666574, 0.2343750000000000000, 0.2395833333333333426, 0.2447916666666666574, 0.2500000000000000000, 0.2552083333333333148, 0.2604166666666666852, 0.2656250000000000000, 0.2708333333333333148, 0.2760416666666666852, 0.2812500000000000000, 0.2864583333333333148, 0.2916666666666666852, 0.2968750000000000000, 0.3020833333333333148, 0.3072916666666666852, 0.3125000000000000000, 0.3177083333333333148, 0.3229166666666666852, 0.3281250000000000000, 0.3333333333333333148, 0.3385416666666666852, 0.3437500000000000000, 0.3489583333333333148, 0.3541666666666666852, 0.3593750000000000000, 0.3645833333333333148, 0.3697916666666666852, 0.3750000000000000000, 0.3802083333333333148, 0.3854166666666666852, 0.3906250000000000000, 0.3958333333333333148, 0.4010416666666666852, 0.4062500000000000000, 0.4114583333333333148, 0.4166666666666666852, 0.4218750000000000000, 0.4270833333333333148, 0.4322916666666666852, 0.4375000000000000000, 0.4427083333333333148, 0.4479166666666666852, 0.4531250000000000000, 0.4583333333333333148, 0.4635416666666666852, 0.4687500000000000000, 0.4739583333333333148, 0.4791666666666666852, 0.4843750000000000000, 0.4895833333333333148, 0.4947916666666666852, 0.5000000000000000000, 0.5052083333333333703, 0.5104166666666666297, 0.5156250000000000000, 0.5208333333333333703, 0.5260416666666666297, 0.5312500000000000000, 0.5364583333333333703, 0.5416666666666666297, 0.5468750000000000000, 0.5520833333333333703, 0.5572916666666666297, 0.5625000000000000000, 0.5677083333333333703, 0.5729166666666666297, 0.5781250000000000000, 0.5833333333333333703, 0.5885416666666666297, 0.5937500000000000000, 0.5989583333333333703, 0.6041666666666666297, 0.6093750000000000000, 0.6145833333333333703, 0.6197916666666666297, 0.6250000000000000000, 0.6302083333333333703, 0.6354166666666666297, 0.6406250000000000000, 0.6458333333333333703, 0.6510416666666666297, 0.6562500000000000000, 0.6614583333333333703, 0.6666666666666666297, 0.6718750000000000000, 0.6770833333333333703, 0.6822916666666666297, 0.6875000000000000000, 0.6927083333333333703, 0.6979166666666666297, 0.7031250000000000000, 0.7083333333333333703, 0.7135416666666666297, 0.7187500000000000000, 0.7239583333333333703, 0.7291666666666666297, 0.7343750000000000000, 0.7395833333333333703, 0.7447916666666666297, 0.7500000000000000000, 0.7552083333333333703, 0.7604166666666666297, 0.7656250000000000000, 0.7708333333333333703, 0.7760416666666666297, 0.7812500000000000000, 0.7864583333333333703, 0.7916666666666666297, 0.7968750000000000000, 0.8020833333333333703, 0.8072916666666666297, 0.8125000000000000000, 0.8177083333333333703, 0.8229166666666666297, 0.8281250000000000000, 0.8333333333333333703, 0.8385416666666666297, 0.8437500000000000000, 0.8489583333333333703, 0.8541666666666666297, 0.8593750000000000000, 0.8645833333333333703, 0.8697916666666666297, 0.8750000000000000000, 0.8802083333333333703, 0.8854166666666666297, 0.8906250000000000000, 0.8958333333333333703, 0.9010416666666666297, 0.9062500000000000000, 0.9114583333333333703, 0.9166666666666666297, 0.9218750000000000000, 0.9270833333333333703, 0.9322916666666666297, 0.9375000000000000000, 0.9427083333333333703, 0.9479166666666666297, 0.9531250000000000000, 0.9583333333333333703, 0.9635416666666666297, 0.9687500000000000000, 0.9739583333333333703, 0.9791666666666666297, 0.9843750000000000000, 0.9895833333333333703, 0.9947916666666666297, 1.000000000000000000 ),
 .UNSPECIFIED. ) 
 GEOMETRIC_REPRESENTATION_ITEM ( )  RATIONAL_B_SPLINE_SURFACE ( (
 ( 1.000000000000000000, 0.8660254037844387076, 1.000000000000000000, 0.8660254037844387076, 1.000000000000000000, 0.8660254037844387076, 1.000000000000000000, 0.8660254037844387076, 1.000000000000000000, 0.8660254037844387076, 1.000000000000000000, 0.8660254037844387076, 1.000000000000000000, 0.8660254037844387076, 1.000000000000000000, 0.8660254037844387076, 1.000000000000000000, 0.8660254037844387076, 1.000000000000000000, 0.8660254037844387076, 1.000000000000000000, 0.8660254037844387076, 1.000000000000000000, 0.8660254037844387076, 1.000000000000000000, 0.8660254037844387076, 1.000000000000000000, 0.8660254037844387076, 1.000000000000000000, 0.8660254037844387076, 1.000000000000000000, 0.8660254037844387076, 1.000000000000000000, 0.8660254037844387076, 1.000000000000000000, 0.8660254037844387076, 1.000000000000000000, 0.8660254037844387076, 1.000000000000000000, 0.8660254037844387076, 1.000000000000000000, 0.8660254037844387076, 1.000000000000000000, 0.8660254037844387076, 1.000000000000000000, 0.8660254037844387076, 1.000000000000000000, 0.8660254037844387076, 1.000000000000000000, 0.8660254037844387076, 1.000000000000000000, 0.8660254037844387076, 1.000000000000000000, 0.8660254037844387076, 1.000000000000000000, 0.8660254037844387076, 1.000000000000000000, 0.8660254037844387076, 1.000000000000000000, 0.8660254037844387076, 1.000000000000000000, 0.8660254037844387076, 1.000000000000000000, 0.8660254037844387076, 1.000000000000000000, 0.8660254037844387076, 1.000000000000000000, 0.8660254037844387076, 1.000000000000000000, 0.8660254037844387076, 1.000000000000000000, 0.8660254037844387076, 1.000000000000000000, 0.8660254037844387076, 1.000000000000000000, 0.8660254037844387076, 1.000000000000000000, 0.8660254037844387076, 1.000000000000000000, 0.8660254037844387076, 1.000000000000000000, 0.8660254037844387076, 1.000000000000000000, 0.8660254037844387076, 1.000000000000000000, 0.8660254037844387076, 1.000000000000000000, 0.8660254037844387076, 1.000000000000000000, 0.8660254037844387076, 1.000000000000000000, 0.8660254037844387076, 1.000000000000000000, 0.8660254037844387076, 1.000000000000000000, 0.8660254037844387076, 1.000000000000000000, 0.8660254037844387076, 1.000000000000000000, 0.8660254037844387076, 1.000000000000000000, 0.8660254037844387076, 1.000000000000000000, 0.8660254037844387076, 1.000000000000000000, 0.8660254037844387076, 1.000000000000000000, 0.8660254037844387076, 1.000000000000000000, 0.8660254037844387076, 1.000000000000000000, 0.8660254037844387076, 1.000000000000000000, 0.8660254037844387076, 1.000000000000000000, 0.8660254037844387076, 1.000000000000000000, 0.8660254037844387076, 1.000000000000000000, 0.8660254037844387076, 1.000000000000000000, 0.8660254037844387076, 1.000000000000000000, 0.8660254037844387076, 1.000000000000000000, 0.8660254037844387076, 1.000000000000000000, 0.8660254037844387076, 1.000000000000000000, 0.8660254037844387076, 1.000000000000000000, 0.8660254037844387076, 1.000000000000000000, 0.8660254037844387076, 1.000000000000000000, 0.8660254037844387076, 1.000000000000000000, 0.8660254037844387076, 1.000000000000000000, 0.8660254037844387076, 1.000000000000000000, 0.8660254037844387076, 1.000000000000000000, 0.8660254037844387076, 1.000000000000000000, 0.8660254037844387076, 1.000000000000000000, 0.8660254037844387076, 1.000000000000000000, 0.8660254037844387076, 1.000000000000000000, 0.8660254037844387076, 1.000000000000000000, 0.8660254037844387076, 1.000000000000000000, 0.8660254037844387076, 1.000000000000000000, 0.8660254037844387076, 1.000000000000000000, 0.8660254037844387076, 1.000000000000000000, 0.8660254037844387076, 1.000000000000000000, 0.8660254037844387076, 1.000000000000000000, 0.8660254037844387076, 1.000000000000000000, 0.8660254037844387076, 1.000000000000000000, 0.8660254037844387076, 1.000000000000000000, 0.8660254037844387076, 1.000000000000000000, 0.8660254037844387076, 1.000000000000000000, 0.8660254037844387076, 1.000000000000000000, 0.8660254037844387076, 1.000000000000000000, 0.8660254037844387076, 1.000000000000000000, 0.8660254037844387076, 1.000000000000000000, 0.8660254037844387076, 1.000000000000000000, 0.8660254037844387076, 1.000000000000000000, 0.8660254037844387076, 1.000000000000000000, 0.8660254037844387076, 1.000000000000000000, 0.8660254037844387076, 1.000000000000000000, 0.8660254037844387076, 1.000000000000000000, 0.8660254037844387076, 1.000000000000000000, 0.8660254037844387076, 1.000000000000000000, 0.8660254037844387076, 1.000000000000000000, 0.8660254037844387076, 1.000000000000000000, 0.8660254037844387076, 1.000000000000000000, 0.8660254037844387076, 1.000000000000000000, 0.8660254037844387076, 1.000000000000000000, 0.8660254037844387076, 1.000000000000000000, 0.8660254037844387076, 1.000000000000000000, 0.8660254037844387076, 1.000000000000000000, 0.8660254037844387076, 1.000000000000000000, 0.8660254037844387076, 1.000000000000000000, 0.8660254037844387076, 1.000000000000000000, 0.8660254037844387076, 1.000000000000000000, 0.8660254037844387076, 1.000000000000000000, 0.8660254037844387076, 1.000000000000000000, 0.8660254037844387076, 1.000000000000000000, 0.8660254037844387076, 1.000000000000000000, 0.8660254037844387076, 1.000000000000000000, 0.8660254037844387076, 1.000000000000000000, 0.8660254037844387076, 1.000000000000000000, 0.8660254037844387076, 1.000000000000000000, 0.8660254037844387076, 1.000000000000000000, 0.8660254037844387076, 1.000000000000000000, 0.8660254037844387076, 1.000000000000000000, 0.8660254037844387076, 1.000000000000000000, 0.8660254037844387076, 1.000000000000000000, 0.8660254037844387076, 1.000000000000000000, 0.8660254037844387076, 1.000000000000000000, 0.8660254037844387076, 1.000000000000000000, 0.8660254037844387076, 1.000000000000000000, 0.8660254037844387076, 1.000000000000000000, 0.8660254037844387076, 1.000000000000000000, 0.8660254037844387076, 1.000000000000000000, 0.8660254037844387076, 1.000000000000000000, 0.8660254037844387076, 1.000000000000000000, 0.8660254037844387076, 1.000000000000000000, 0.8660254037844387076, 1.000000000000000000, 0.8660254037844387076, 1.000000000000000000, 0.8660254037844387076, 1.000000000000000000, 0.8660254037844387076, 1.000000000000000000, 0.8660254037844387076, 1.000000000000000000, 0.8660254037844387076, 1.000000000000000000, 0.8660254037844387076, 1.000000000000000000, 0.8660254037844387076, 1.000000000000000000, 0.8660254037844387076, 1.000000000000000000, 0.8660254037844387076, 1.000000000000000000, 0.8660254037844387076, 1.000000000000000000, 0.8660254037844387076, 1.000000000000000000, 0.8660254037844387076, 1.000000000000000000, 0.8660254037844387076, 1.000000000000000000, 0.8660254037844387076, 1.000000000000000000, 0.8660254037844387076, 1.000000000000000000, 0.8660254037844387076, 1.000000000000000000, 0.8660254037844387076, 1.000000000000000000, 0.8660254037844387076, 1.000000000000000000, 0.8660254037844387076, 1.000000000000000000, 0.8660254037844387076, 1.000000000000000000, 0.8660254037844387076, 1.000000000000000000, 0.8660254037844387076, 1.000000000000000000, 0.8660254037844387076, 1.000000000000000000, 0.8660254037844387076, 1.000000000000000000, 0.8660254037844387076, 1.000000000000000000, 0.8660254037844387076, 1.000000000000000000, 0.8660254037844387076, 1.000000000000000000, 0.8660254037844387076, 1.000000000000000000, 0.8660254037844387076, 1.000000000000000000, 0.8660254037844387076, 1.000000000000000000, 0.8660254037844387076, 1.000000000000000000, 0.8660254037844387076, 1.000000000000000000, 0.8660254037844387076, 1.000000000000000000, 0.8660254037844387076, 1.000000000000000000, 0.8660254037844387076, 1.000000000000000000, 0.8660254037844387076, 1.000000000000000000, 0.8660254037844387076, 1.000000000000000000, 0.8660254037844387076, 1.000000000000000000, 0.8660254037844387076, 1.000000000000000000, 0.8660254037844387076, 1.000000000000000000, 0.8660254037844387076, 1.000000000000000000, 0.8660254037844387076, 1.000000000000000000, 0.8660254037844387076, 1.000000000000000000, 0.8660254037844387076, 1.000000000000000000, 0.8660254037844387076, 1.000000000000000000, 0.8660254037844387076, 1.000000000000000000, 0.8660254037844387076, 1.000000000000000000, 0.8660254037844387076, 1.000000000000000000, 0.8660254037844387076, 1.000000000000000000, 0.8660254037844387076, 1.000000000000000000, 0.8660254037844387076, 1.000000000000000000, 0.8660254037844387076, 1.000000000000000000, 0.8660254037844387076, 1.000000000000000000, 0.8660254037844387076, 1.000000000000000000, 0.8660254037844387076, 1.000000000000000000, 0.8660254037844387076, 1.000000000000000000, 0.8660254037844387076, 1.000000000000000000),
 ( 1.000000000000000000, 0.8660254037844387076, 1.000000000000000000, 0.8660254037844387076, 1.000000000000000000, 0.8660254037844387076, 1.000000000000000000, 0.8660254037844387076, 1.000000000000000000, 0.8660254037844387076, 1.000000000000000000, 0.8660254037844387076, 1.000000000000000000, 0.8660254037844387076, 1.000000000000000000, 0.8660254037844387076, 1.000000000000000000, 0.8660254037844387076, 1.000000000000000000, 0.8660254037844387076, 1.000000000000000000, 0.8660254037844387076, 1.000000000000000000, 0.8660254037844387076, 1.000000000000000000, 0.8660254037844387076, 1.000000000000000000, 0.8660254037844387076, 1.000000000000000000, 0.8660254037844387076, 1.000000000000000000, 0.8660254037844387076, 1.000000000000000000, 0.8660254037844387076, 1.000000000000000000, 0.8660254037844387076, 1.000000000000000000, 0.8660254037844387076, 1.000000000000000000, 0.8660254037844387076, 1.000000000000000000, 0.8660254037844387076, 1.000000000000000000, 0.8660254037844387076, 1.000000000000000000, 0.8660254037844387076, 1.000000000000000000, 0.8660254037844387076, 1.000000000000000000, 0.8660254037844387076, 1.000000000000000000, 0.8660254037844387076, 1.000000000000000000, 0.8660254037844387076, 1.000000000000000000, 0.8660254037844387076, 1.000000000000000000, 0.8660254037844387076, 1.000000000000000000, 0.8660254037844387076, 1.000000000000000000, 0.8660254037844387076, 1.000000000000000000, 0.8660254037844387076, 1.000000000000000000, 0.8660254037844387076, 1.000000000000000000, 0.8660254037844387076, 1.000000000000000000, 0.8660254037844387076, 1.000000000000000000, 0.8660254037844387076, 1.000000000000000000, 0.8660254037844387076, 1.000000000000000000, 0.8660254037844387076, 1.000000000000000000, 0.8660254037844387076, 1.000000000000000000, 0.8660254037844387076, 1.000000000000000000, 0.8660254037844387076, 1.000000000000000000, 0.8660254037844387076, 1.000000000000000000, 0.8660254037844387076, 1.000000000000000000, 0.8660254037844387076, 1.000000000000000000, 0.8660254037844387076, 1.000000000000000000, 0.8660254037844387076, 1.000000000000000000, 0.8660254037844387076, 1.000000000000000000, 0.8660254037844387076, 1.000000000000000000, 0.8660254037844387076, 1.000000000000000000, 0.8660254037844387076, 1.000000000000000000, 0.8660254037844387076, 1.000000000000000000, 0.8660254037844387076, 1.000000000000000000, 0.8660254037844387076, 1.000000000000000000, 0.8660254037844387076, 1.000000000000000000, 0.8660254037844387076, 1.000000000000000000, 0.8660254037844387076, 1.000000000000000000, 0.8660254037844387076, 1.000000000000000000, 0.8660254037844387076, 1.000000000000000000, 0.8660254037844387076, 1.000000000000000000, 0.8660254037844387076, 1.000000000000000000, 0.8660254037844387076, 1.000000000000000000, 0.8660254037844387076, 1.000000000000000000, 0.8660254037844387076, 1.000000000000000000, 0.8660254037844387076, 1.000000000000000000, 0.8660254037844387076, 1.000000000000000000, 0.8660254037844387076, 1.000000000000000000, 0.8660254037844387076, 1.000000000000000000, 0.8660254037844387076, 1.000000000000000000, 0.8660254037844387076, 1.000000000000000000, 0.8660254037844387076, 1.000000000000000000, 0.8660254037844387076, 1.000000000000000000, 0.8660254037844387076, 1.000000000000000000, 0.8660254037844387076, 1.000000000000000000, 0.8660254037844387076, 1.000000000000000000, 0.8660254037844387076, 1.000000000000000000, 0.8660254037844387076, 1.000000000000000000, 0.8660254037844387076, 1.000000000000000000, 0.8660254037844387076, 1.000000000000000000, 0.8660254037844387076, 1.000000000000000000, 0.8660254037844387076, 1.000000000000000000, 0.8660254037844387076, 1.000000000000000000, 0.8660254037844387076, 1.000000000000000000, 0.8660254037844387076, 1.000000000000000000, 0.8660254037844387076, 1.000000000000000000, 0.8660254037844387076, 1.000000000000000000, 0.8660254037844387076, 1.000000000000000000, 0.8660254037844387076, 1.000000000000000000, 0.8660254037844387076, 1.000000000000000000, 0.8660254037844387076, 1.000000000000000000, 0.8660254037844387076, 1.000000000000000000, 0.8660254037844387076, 1.000000000000000000, 0.8660254037844387076, 1.000000000000000000, 0.8660254037844387076, 1.000000000000000000, 0.8660254037844387076, 1.000000000000000000, 0.8660254037844387076, 1.000000000000000000, 0.8660254037844387076, 1.000000000000000000, 0.8660254037844387076, 1.000000000000000000, 0.8660254037844387076, 1.000000000000000000, 0.8660254037844387076, 1.000000000000000000, 0.8660254037844387076, 1.000000000000000000, 0.8660254037844387076, 1.000000000000000000, 0.8660254037844387076, 1.000000000000000000, 0.8660254037844387076, 1.000000000000000000, 0.8660254037844387076, 1.000000000000000000, 0.8660254037844387076, 1.000000000000000000, 0.8660254037844387076, 1.000000000000000000, 0.8660254037844387076, 1.000000000000000000, 0.8660254037844387076, 1.000000000000000000, 0.8660254037844387076, 1.000000000000000000, 0.8660254037844387076, 1.000000000000000000, 0.8660254037844387076, 1.000000000000000000, 0.8660254037844387076, 1.000000000000000000, 0.8660254037844387076, 1.000000000000000000, 0.8660254037844387076, 1.000000000000000000, 0.8660254037844387076, 1.000000000000000000, 0.8660254037844387076, 1.000000000000000000, 0.8660254037844387076, 1.000000000000000000, 0.8660254037844387076, 1.000000000000000000, 0.8660254037844387076, 1.000000000000000000, 0.8660254037844387076, 1.000000000000000000, 0.8660254037844387076, 1.000000000000000000, 0.8660254037844387076, 1.000000000000000000, 0.8660254037844387076, 1.000000000000000000, 0.8660254037844387076, 1.000000000000000000, 0.8660254037844387076, 1.000000000000000000, 0.8660254037844387076, 1.000000000000000000, 0.8660254037844387076, 1.000000000000000000, 0.8660254037844387076, 1.000000000000000000, 0.8660254037844387076, 1.000000000000000000, 0.8660254037844387076, 1.000000000000000000, 0.8660254037844387076, 1.000000000000000000, 0.8660254037844387076, 1.000000000000000000, 0.8660254037844387076, 1.000000000000000000, 0.8660254037844387076, 1.000000000000000000, 0.8660254037844387076, 1.000000000000000000, 0.8660254037844387076, 1.000000000000000000, 0.8660254037844387076, 1.000000000000000000, 0.8660254037844387076, 1.000000000000000000, 0.8660254037844387076, 1.000000000000000000, 0.8660254037844387076, 1.000000000000000000, 0.8660254037844387076, 1.000000000000000000, 0.8660254037844387076, 1.000000000000000000, 0.8660254037844387076, 1.000000000000000000, 0.8660254037844387076, 1.000000000000000000, 0.8660254037844387076, 1.000000000000000000, 0.8660254037844387076, 1.000000000000000000, 0.8660254037844387076, 1.000000000000000000, 0.8660254037844387076, 1.000000000000000000, 0.8660254037844387076, 1.000000000000000000, 0.8660254037844387076, 1.000000000000000000, 0.8660254037844387076, 1.000000000000000000, 0.8660254037844387076, 1.000000000000000000, 0.8660254037844387076, 1.000000000000000000, 0.8660254037844387076, 1.000000000000000000, 0.8660254037844387076, 1.000000000000000000, 0.8660254037844387076, 1.000000000000000000, 0.8660254037844387076, 1.000000000000000000, 0.8660254037844387076, 1.000000000000000000, 0.8660254037844387076, 1.000000000000000000, 0.8660254037844387076, 1.000000000000000000, 0.8660254037844387076, 1.000000000000000000, 0.8660254037844387076, 1.000000000000000000, 0.8660254037844387076, 1.000000000000000000, 0.8660254037844387076, 1.000000000000000000, 0.8660254037844387076, 1.000000000000000000, 0.8660254037844387076, 1.000000000000000000, 0.8660254037844387076, 1.000000000000000000, 0.8660254037844387076, 1.000000000000000000, 0.8660254037844387076, 1.000000000000000000, 0.8660254037844387076, 1.000000000000000000, 0.8660254037844387076, 1.000000000000000000, 0.8660254037844387076, 1.000000000000000000, 0.8660254037844387076, 1.000000000000000000, 0.8660254037844387076, 1.000000000000000000, 0.8660254037844387076, 1.000000000000000000, 0.8660254037844387076, 1.000000000000000000, 0.8660254037844387076, 1.000000000000000000, 0.8660254037844387076, 1.000000000000000000, 0.8660254037844387076, 1.000000000000000000, 0.8660254037844387076, 1.000000000000000000, 0.8660254037844387076, 1.000000000000000000, 0.8660254037844387076, 1.000000000000000000, 0.8660254037844387076, 1.000000000000000000, 0.8660254037844387076, 1.000000000000000000, 0.8660254037844387076, 1.000000000000000000, 0.8660254037844387076, 1.000000000000000000, 0.8660254037844387076, 1.000000000000000000, 0.8660254037844387076, 1.000000000000000000, 0.8660254037844387076, 1.000000000000000000, 0.8660254037844387076, 1.000000000000000000, 0.8660254037844387076, 1.000000000000000000, 0.8660254037844387076, 1.000000000000000000) ) ) 
 REPRESENTATION_ITEM ( '' )  SURFACE ( )  );
#2892=LINE ( 'NONE', #1885, #358 ) ;
#2894=ORIENTED_EDGE ( 'NONE', *, *, #10862, .F. ) ;
#2895=CARTESIAN_POINT ( 'NONE',  ( -61.13531646874998415, 16.07812499965860198, 1.500000000000002220 ) ) ;
#2896=CARTESIAN_POINT ( 'NONE',  ( -62.49999999999998579, 9.635416665983870033, 2.366025403784441483 ) ) ;
#2900=CARTESIAN_POINT ( 'NONE',  ( -61.99999999999999289, 14.82812499965860020, 2.498450539062049724 ) ) ;
#2901=CARTESIAN_POINT ( 'NONE',  ( -62.86468353124999453, 9.953124999658601979, 1.500000000000002220 ) ) ;
#2903=CARTESIAN_POINT ( 'NONE',  ( -62.49999999999998579, 11.38541666598387003, 2.366025403784441483 ) ) ;
#2905=CARTESIAN_POINT ( 'NONE',  ( -62.86468353124999453, 10.76562499965860020, 1.500000000000002220 ) ) ;
#2908=CARTESIAN_POINT ( 'NONE',  ( -61.73205080756886076, 13.91741454900183150, 2.500000000000003109 ) ) ;
#2911=CARTESIAN_POINT ( 'NONE',  ( -62.49999999999998579, 10.30208333265053611, 0.6339745962155627357 ) ) ;
#2912=CARTESIAN_POINT ( 'NONE',  ( -61.13531646874998415, 12.32812499965860198, 1.500000000000002220 ) ) ;
#2913=CARTESIAN_POINT ( 'NONE',  ( -61.56765823437498142, 10.11979166632526805, 0.7511620957034663704 ) ) ;
#2914=DIRECTION ( 'NONE',  ( 0.000000000000000000, 1.000000000000000000, 0.000000000000000000 ) ) ;
#2917=CARTESIAN_POINT ( 'NONE',  ( -62.86468353124999453, 10.26562499965860198, 1.500000000000002220 ) ) ;
#2920=CARTESIAN_POINT ( 'NONE',  ( -62.43234176562499016, 15.74479166632526628, 2.248837904296538071 ) ) ;
#2922=CARTESIAN_POINT ( 'NONE',  ( -61.49999999999998579, 15.17708333265053611, 2.366025403784441927 ) ) ;
#2923=DIRECTION ( 'NONE',  ( -0.000000000000000000, -1.000000000000000000, -0.000000000000000000 ) ) ;
#2924=ORIENTED_EDGE ( 'NONE', *, *, #2766, .F. ) ;
#2926=CARTESIAN_POINT ( 'NONE',  ( -61.49999999999998579, 15.26041666598387003, 0.6339745962155628467 ) ) ;
#2927=ORIENTED_EDGE ( 'NONE', *, *, #1789, .F. ) ;
#2928=CARTESIAN_POINT ( 'NONE',  ( -61.56765823437498852, 13.03645833299193413, 2.248837904296538515 ) ) ;
#2929=FACE_OUTER_BOUND ( 'NONE', #9248, .T. ) ;
#2932=CARTESIAN_POINT ( 'NONE',  ( -60.99999999999998579, 12.22916666666666607, 2.077350269189628840 ) ) ;
#2933=CARTESIAN_POINT ( 'NONE',  ( -61.99999999999998579, 10.18750000000000000, 2.500000000000002665 ) ) ;
#2934=CARTESIAN_POINT ( 'NONE',  ( -61.56765823437498142, 13.93229166632526805, 0.7511620957034663704 ) ) ;
#2936=CARTESIAN_POINT ( 'NONE',  ( -60.99999999999998579, 10.69791666598386826, 2.077350269189628840 ) ) ;
#2938=CARTESIAN_POINT ( 'NONE',  ( -61.99999999999998579, 9.031249999317202182, 0.5000000000000013323 ) ) ;
#2940=CARTESIAN_POINT ( 'NONE',  ( -61.13531646874998415, 12.34895833299193413, 1.000774730468978468 ) ) ;
#2942=CARTESIAN_POINT ( 'NONE',  ( -62.86468353124999453, 9.765624999658601979, 1.500000000000002220 ) ) ;
#2943=DIRECTION ( 'NONE',  ( 0.000000000000000000, 1.000000000000000000, 0.000000000000000000 ) ) ;
#2944=CARTESIAN_POINT ( 'NONE',  ( -61.13531646874998415, 14.89062499965860020, 1.500000000000002220 ) ) ;
#2945=DIRECTION ( 'NONE',  ( -0.000000000000000000, -1.000000000000000000, -0.000000000000000000 ) ) ;
#2946=ORIENTED_EDGE ( 'NONE', *, *, #9058, .F. ) ;
#2948=CARTESIAN_POINT ( 'NONE',  ( -60.99999999999998579, 10.50000000000000000, 1.500000000000002220 ) ) ;
#2949=EDGE_LOOP ( 'NONE', ( #9711, #5951, #8530, #9448, #4313, #264, #9290, #9116, #7777, #10190, #6222, #9896, #9511, #2704, #4881, #245, #6159, #5797, #5538, #10580, #10595, #2074, #2078, #6081, #80, #9141, #5924, #5134, #9365, #1884, #3601, #7168, #6310, #1099, #10456, #1964, #2104, #4176, #8340, #8102, #748, #10526, #2772, #10101, #1305, #9150, #1971, #3834, #8363, #7644, #6940, #2370, #3390, #2603, #10154, #5055, #8593, #2871, #8588, #8429, #10090, #7862, #5333, #2867, #4189, #10423, #5514, #8080, #9278 ) ) ;
#2950=CARTESIAN_POINT ( 'NONE',  ( -61.99999999999998579, 11.81250000000000000, 0.5000000000000013323 ) ) ;
#2951=EDGE_CURVE ( 'NONE', #10259, #6433, #2582, .T. ) ;
#2952=CARTESIAN_POINT ( 'NONE',  ( -61.56765823437498852, 16.03645833299193768, 2.248837904296538515 ) ) ;
#2956=CARTESIAN_POINT ( 'NONE',  ( -62.43234176562498305, 10.41145833299193413, 0.7511620957034662593 ) ) ;
#2957=CARTESIAN_POINT ( 'NONE',  ( -60.99999999999998579, 11.98958333265053611, 0.9226497308103762673 ) ) ;
#2958=( BOUNDED_CURVE ( )  B_SPLINE_CURVE ( 2, ( #5097, #165, #7617, #2, #8502, #6947, #10939, #885, #1675 ),
 .UNSPECIFIED., .F., .F. ) 
 B_SPLINE_CURVE_WITH_KNOTS ( ( 3, 2, 2, 2, 3 ),
 ( 0.3359374999999999445, 0.3385416666666666852, 0.3437500000000000000, 0.3489583333333333148, 0.3515625000000000000 ),
 .UNSPECIFIED. ) 
 CURVE ( )  GEOMETRIC_REPRESENTATION_ITEM ( )  RATIONAL_B_SPLINE_CURVE ( ( 0.9330127018922192983, 0.9330127018922178550, 1.000000000000000000, 0.8660254037844387076, 1.000000000000000000, 0.8660254037844387076, 1.000000000000000000, 0.9330127018922194093, 0.9330127018922194093 ) ) 
 REPRESENTATION_ITEM ( '' )  );
#2960=CARTESIAN_POINT ( 'NONE',  ( -62.43234176562498305, 9.973958332991934128, 0.7511620957034662593 ) ) ;
#2964=CARTESIAN_POINT ( 'NONE',  ( -61.73205080756886076, 15.30133545031537068, 0.5000000000000014433 ) ) ;
#2966=CARTESIAN_POINT ( 'NONE',  ( -60.99999999999998579, 15.72916666666666430, 2.077350269189628840 ) ) ;
#2967=CARTESIAN_POINT ( 'NONE',  ( -61.56765823437498142, 12.11979166632526628, 0.7511620957034663704 ) ) ;
#2968=CARTESIAN_POINT ( 'NONE',  ( -61.13531646874997705, 10.34895833299193413, 1.000774730468978468 ) ) ;
#2969=ORIENTED_EDGE ( 'NONE', *, *, #5488, .F. ) ;
#2970=DIRECTION ( 'NONE',  ( -0.000000000000000000, -1.000000000000000000, -0.000000000000000000 ) ) ;
#2971=CARTESIAN_POINT ( 'NONE',  ( -61.99999999999999289, 10.95312499965860020, 0.5015494609379544944 ) ) ;
#2973=CARTESIAN_POINT ( 'NONE',  ( -61.56765823437498852, 15.53645833299193590, 2.248837904296538515 ) ) ;
#2974=CARTESIAN_POINT ( 'NONE',  ( -62.49999999999998579, 14.05208333265053611, 0.6339745962155627357 ) ) ;
#2976=ORIENTED_EDGE ( 'NONE', *, *, #10172, .T. ) ;
#2979=VERTEX_POINT ( 'NONE', #8532 ) ;
#2981=CARTESIAN_POINT ( 'NONE',  ( -61.13531646874997705, 13.34895833299193413, 1.000774730468978468 ) ) ;
#2983=CARTESIAN_POINT ( 'NONE',  ( -60.99999999999998579, 11.77083333333333393, 0.9226497308103762673 ) ) ;
#2985=CARTESIAN_POINT ( 'NONE',  ( -61.49999999999998579, 12.95833333333333215, 2.366025403784441927 ) ) ;
#2986=CARTESIAN_POINT ( 'NONE',  ( -62.99999999999998579, 8.614583332650536107, 2.077350269189627952 ) ) ;
#2989=CARTESIAN_POINT ( 'NONE',  ( -62.99999999999998579, 10.11458333265053611, 2.077350269189627952 ) ) ;
#2993=CARTESIAN_POINT ( 'NONE',  ( -62.43234176562498305, 13.16145833299193413, 0.7511620957034662593 ) ) ;
#2996=VECTOR ( 'NONE', #5662, 1000.000000000000000 ) ;
#2997=CARTESIAN_POINT ( 'NONE',  ( -61.13531646874998415, 10.36979166632526805, 1.999225269531026417 ) ) ;
#3000=CARTESIAN_POINT ( 'NONE',  ( -61.13531646874998415, 15.61979166632526628, 1.999225269531026417 ) ) ;
#3002=VERTEX_POINT ( 'NONE', #81 ) ;
#3008=CARTESIAN_POINT ( 'NONE',  ( -61.99999999999998579, 9.312500000000001776, 0.3452994616207497591 ) ) ;
#3010=CARTESIAN_POINT ( 'NONE',  ( -61.99999999999998579, 9.890624999658601979, 0.5015494609379544944 ) ) ;
#3011=CARTESIAN_POINT ( 'NONE',  ( -62.99999999999998579, 8.322916665983870033, 0.9226497308103756012 ) ) ;
#3012=CARTESIAN_POINT ( 'NONE',  ( -61.13531646874998415, 11.36979166632526628, 1.999225269531026417 ) ) ;
#3016=EDGE_CURVE ( 'NONE', #6871, #1245, #1161, .T. ) ;
#3017=LINE ( 'NONE', #1299, #934 ) ;
#3019=ORIENTED_EDGE ( 'NONE', *, *, #2951, .F. ) ;
#3020=CARTESIAN_POINT ( 'NONE',  ( -61.99999999999998579, 10.40624999931720218, 2.500000000000002665 ) ) ;
#3021=CARTESIAN_POINT ( 'NONE',  ( -62.43234176562499016, 14.49479166632526983, 2.248837904296538071 ) ) ;
#3022=CARTESIAN_POINT ( 'NONE',  ( -61.13531646874998415, 10.32812499965860198, 1.500000000000002220 ) ) ;
#3023=MECHANICAL_DESIGN_GEOMETRIC_PRESENTATION_REPRESENTATION('',(#8172),#6581);
#3025=( BOUNDED_CURVE ( )  B_SPLINE_CURVE ( 2, ( #8341, #5619, #3219, #6628, #9957, #9852, #7401, #3280, #10782 ),
 .UNSPECIFIED., .F., .T. ) 
 B_SPLINE_CURVE_WITH_KNOTS ( ( 3, 2, 2, 2, 3 ),
 ( 0.6796875000000000000, 0.6822916666666666297, 0.6875000000000000000, 0.6927083333333333703, 0.6953125000000000000 ),
 .UNSPECIFIED. ) 
 CURVE ( )  GEOMETRIC_REPRESENTATION_ITEM ( )  RATIONAL_B_SPLINE_CURVE ( ( 0.9330127018922194093, 0.9330127018922194093, 1.000000000000000000, 0.8660254037844387076, 1.000000000000000000, 0.8660254037844387076, 1.000000000000000000, 0.9330127018922194093, 0.9330127018922194093 ) ) 
 REPRESENTATION_ITEM ( '' )  );
#3027=CARTESIAN_POINT ( 'NONE',  ( -61.99999999999998579, 14.81250000000000000, 0.5000000000000013323 ) ) ;
#3028=CARTESIAN_POINT ( 'NONE',  ( -62.86468353124999453, 10.78645833299193413, 1.999225269531025750 ) ) ;
#3030=CARTESIAN_POINT ( 'NONE',  ( -62.49999999999998579, 15.08333333333333393, 0.6339745962155627357 ) ) ;
#3031=AXIS2_PLACEMENT_3D ( 'NONE', #9664, #9718, #6998 ) ;
#3032=CARTESIAN_POINT ( 'NONE',  ( -62.99999999999998579, 14.11458333265053433, 2.077350269189627952 ) ) ;
#3033=CARTESIAN_POINT ( 'NONE',  ( -61.99999999999998579, 16.00000000000000000, 2.500000000000000444 ) ) ;
#3037=VERTEX_POINT ( 'NONE', #5321 ) ;
#3038=CARTESIAN_POINT ( 'NONE',  ( -61.56765823437498142, 12.61979166632526805, 0.7511620957034663704 ) ) ;
#3039=CARTESIAN_POINT ( 'NONE',  ( -61.56765823437498142, 9.119791666325268054, 0.7511620957034663704 ) ) ;
#3040=LINE ( 'NONE', #9033, #9793 ) ;
#3041=ORIENTED_EDGE ( 'NONE', *, *, #3250, .T. ) ;
#3042=CARTESIAN_POINT ( 'NONE',  ( -60.99999999999998579, 12.72916666666666785, 2.077350269189628840 ) ) ;
#3044=CARTESIAN_POINT ( 'NONE',  ( -61.99999999999998579, 10.40624999931720396, 2.654700538379254571 ) ) ;
#3048=CARTESIAN_POINT ( 'NONE',  ( -62.86468353124998742, 12.72395833299193413, 1.999225269531025972 ) ) ;
#3051=CARTESIAN_POINT ( 'NONE',  ( -61.56765823437498852, 11.84895833299193413, 2.248837904296538515 ) ) ;
#3054=CARTESIAN_POINT ( 'NONE',  ( -61.99999999999998579, 15.20312499965860020, 0.5015494609379544944 ) ) ;
#3055=VERTEX_POINT ( 'NONE', #9414 ) ;
#3056=DIRECTION ( 'NONE',  ( -0.000000000000000000, -1.000000000000000000, -0.000000000000000000 ) ) ;
#3059=ORIENTED_EDGE ( 'NONE', *, *, #3852, .F. ) ;
#3061=CARTESIAN_POINT ( 'NONE',  ( -62.99999999999998579, 9.104166666666666075, 0.9226497308103756012 ) ) ;
#3063=CARTESIAN_POINT ( 'NONE',  ( -61.99999999999998579, 16.00000000000000000, 2.500000000000000444 ) ) ;
#3064=DIRECTION ( 'NONE',  ( -0.000000000000000000, -1.000000000000000000, -0.000000000000000000 ) ) ;
#3065=CARTESIAN_POINT ( 'NONE',  ( -60.99999999999998579, 15.44791666598387003, 2.077350269189628840 ) ) ;
#3067=CARTESIAN_POINT ( 'NONE',  ( -62.86468353124998032, 12.24479166632526805, 1.000774730468978246 ) ) ;
#3068=CARTESIAN_POINT ( 'NONE',  ( -62.49999999999998579, 13.66666666666666785, 2.366025403784441483 ) ) ;
#3072=VERTEX_POINT ( 'NONE', #5661 ) ;
#3074=CARTESIAN_POINT ( 'NONE',  ( -61.56765823437498852, 13.53645833299193413, 2.248837904296538515 ) ) ;
#3075=CARTESIAN_POINT ( 'NONE',  ( -62.86468353124999453, 9.703124999658601979, 1.500000000000002220 ) ) ;
#3076=LINE ( 'NONE', #416, #2445 ) ;
#3079=CARTESIAN_POINT ( 'NONE',  ( -61.13531646874997705, 11.86979166632526805, 1.999225269531026417 ) ) ;
#3082=CARTESIAN_POINT ( 'NONE',  ( -61.99999999999998579, 15.78124999931720218, 0.3452994616207497591 ) ) ;
#3083=CARTESIAN_POINT ( 'NONE',  ( -61.28647452029539267, 16.00000000000000000, 0.7993707187018740390 ) ) ;
#3084=ORIENTED_EDGE ( 'NONE', *, *, #4899, .F. ) ;
#3088=( BOUNDED_CURVE ( )  B_SPLINE_CURVE ( 2, ( #9450, #3618, #7014, #2789, #1847, #1121, #6177, #10218, #4503 ),
 .UNSPECIFIED., .F., .T. ) 
 B_SPLINE_CURVE_WITH_KNOTS ( ( 3, 2, 2, 2, 3 ),
 ( 0.4140625000000000000, 0.4166666666666666852, 0.4218750000000000000, 0.4270833333333333148, 0.4296875000000000555 ),
 .UNSPECIFIED. ) 
 CURVE ( )  GEOMETRIC_REPRESENTATION_ITEM ( )  RATIONAL_B_SPLINE_CURVE ( ( 0.9330127018922194093, 0.9330127018922194093, 1.000000000000000000, 0.8660254037844387076, 1.000000000000000000, 0.8660254037844387076, 1.000000000000000000, 0.9330127018922178550, 0.9330127018922192983 ) ) 
 REPRESENTATION_ITEM ( '' )  );
#3089=CARTESIAN_POINT ( 'NONE',  ( -62.43234176562499016, 12.74479166632526805, 2.248837904296538071 ) ) ;
#3090=CARTESIAN_POINT ( 'NONE',  ( -61.13531646874998415, 10.30729166632526805, 1.999225269531026417 ) ) ;
#3091=CARTESIAN_POINT ( 'NONE',  ( -61.49999999999998579, 11.79166666666666785, 0.6339745962155628467 ) ) ;
#3092=ORIENTED_EDGE ( 'NONE', *, *, #6873, .F. ) ;
#3093=CARTESIAN_POINT ( 'NONE',  ( -62.99999999999998579, 14.14583333333333215, 2.077350269189627952 ) ) ;
#3097=CARTESIAN_POINT ( 'NONE',  ( -61.99999999999998579, 11.40624999931720218, 2.654700538379254571 ) ) ;
#3099=CARTESIAN_POINT ( 'NONE',  ( -61.13531646874998415, 13.09895833299193413, 1.000774730468978468 ) ) ;
#3101=CARTESIAN_POINT ( 'NONE',  ( -61.99999999999998579, 11.20312499965860198, 0.5015494609379544944 ) ) ;
#3102=CARTESIAN_POINT ( 'NONE',  ( -62.49999999999998579, 12.63541666598386826, 2.366025403784441483 ) ) ;
#3109=CARTESIAN_POINT ( 'NONE',  ( -61.73205080756885366, 9.520085449632571084, 0.5000000000000028866 ) ) ;
#3110=CARTESIAN_POINT ( 'NONE',  ( -61.99999999999998579, 9.937500000000001776, 2.654700538379254571 ) ) ;
#3111=CARTESIAN_POINT ( 'NONE',  ( -60.99999999999998579, 11.25000000000000000, 1.500000000000002220 ) ) ;
#3112=CARTESIAN_POINT ( 'NONE',  ( -60.99999999999998579, 16.21874999931720396, 1.500000000000002220 ) ) ;
#3113=( BOUNDED_CURVE ( )  B_SPLINE_CURVE ( 2, ( #6042, #3372, #2431, #9232, #2596, #6718, #9270, #4200, #10252 ),
 .UNSPECIFIED., .F., .F. ) 
 B_SPLINE_CURVE_WITH_KNOTS ( ( 3, 2, 2, 2, 3 ),
 ( 0.2734375000000000000, 0.2760416666666666852, 0.2812500000000000000, 0.2864583333333333148, 0.2890624999999999445 ),
 .UNSPECIFIED. ) 
 CURVE ( )  GEOMETRIC_REPRESENTATION_ITEM ( )  RATIONAL_B_SPLINE_CURVE ( ( 0.9330127018922194093, 0.9330127018922194093, 1.000000000000000000, 0.8660254037844387076, 1.000000000000000000, 0.8660254037844387076, 1.000000000000000000, 0.9330127018922207416, 0.9330127018922192983 ) ) 
 REPRESENTATION_ITEM ( '' )  );
#3115=CARTESIAN_POINT ( 'NONE',  ( -61.49999999999998579, 8.260416665983870033, 0.6339745962155628467 ) ) ;
#3116=CARTESIAN_POINT ( 'NONE',  ( -61.13531646874998415, 11.86979166632526805, 1.999225269531026417 ) ) ;
#3117=DIRECTION ( 'NONE',  ( 0.8660254037844418162, -0.4999999999999947264, 0.000000000000000000 ) ) ;
#3124=CARTESIAN_POINT ( 'NONE',  ( -62.86468353124998032, 13.43229166632526628, 1.000774730468978246 ) ) ;
#3125=CARTESIAN_POINT ( 'NONE',  ( -62.86468353124998032, 10.18229166632526805, 1.000774730468978024 ) ) ;
#3127=VERTEX_POINT ( 'NONE', #10473 ) ;
#3128=CARTESIAN_POINT ( 'NONE',  ( -61.99999999999998579, 12.28124999931720041, 0.5000000000000013323 ) ) ;
#3129=CARTESIAN_POINT ( 'NONE',  ( -61.13531646874997705, 11.16145833299193413, 1.000774730468978468 ) ) ;
#3131=CARTESIAN_POINT ( 'NONE',  ( -61.99999999999998579, 16.07812499965860198, 2.498450539062049724 ) ) ;
#3133=CARTESIAN_POINT ( 'NONE',  ( -62.99999999999998579, 15.12500000000000000, 1.500000000000001998 ) ) ;
#3134=CARTESIAN_POINT ( 'NONE',  ( -62.49999999999998579, 15.63541666598386826, 2.366025403784441483 ) ) ;
#3137=CARTESIAN_POINT ( 'NONE',  ( -62.99999999999998579, 11.82291666598387003, 0.9226497308103756012 ) ) ;
#3139=CARTESIAN_POINT ( 'NONE',  ( -61.56765823437498852, 14.28645833299193413, 2.248837904296538515 ) ) ;
#3140=CARTESIAN_POINT ( 'NONE',  ( -62.86468353124998032, 10.43229166632526983, 1.000774730468978246 ) ) ;
#3142=ORIENTED_EDGE ( 'NONE', *, *, #4091, .T. ) ;
#3143=CARTESIAN_POINT ( 'NONE',  ( -60.99999999999998579, 13.25000000000000000, 1.500000000000002220 ) ) ;
#3144=CARTESIAN_POINT ( 'NONE',  ( -61.99999999999998579, 8.656249999317202182, 2.500000000000002665 ) ) ;
#3145=EDGE_CURVE ( 'NONE', #6502, #4541, #308, .T. ) ;
#3146=FILL_AREA_STYLE_COLOUR ( '', #7452 ) ;
#3147=CARTESIAN_POINT ( 'NONE',  ( -60.99999999999998579, 11.46874999931720218, 1.500000000000002220 ) ) ;
#3148=CARTESIAN_POINT ( 'NONE',  ( -62.26794919243111082, 14.82366454968463287, 0.5000000000000013323 ) ) ;
#3149=EDGE_CURVE ( 'NONE', #10303, #7043, #5412, .T. ) ;
#3150=CARTESIAN_POINT ( 'NONE',  ( -61.56765823437498142, 14.36979166632526983, 0.7511620957034663704 ) ) ;
#3153=CARTESIAN_POINT ( 'NONE',  ( -61.13531646874998415, 11.11979166632526805, 1.999225269531026417 ) ) ;
#3155=CARTESIAN_POINT ( 'NONE',  ( -62.86468353124998032, 15.24479166632526805, 1.000774730468978246 ) ) ;
#3158=VERTEX_POINT ( 'NONE', #3693 ) ;
#3160=CARTESIAN_POINT ( 'NONE',  ( -62.99999999999998579, 9.604166666666667851, 0.9226497308103756012 ) ) ;
#3161=CARTESIAN_POINT ( 'NONE',  ( -62.26794919243111082, 12.92633545031537068, 2.500000000000003109 ) ) ;
#3162=AXIS2_PLACEMENT_3D ( 'NONE', #7005, #3782, #8011 ) ;
#3163=CARTESIAN_POINT ( 'NONE',  ( -61.56765823437498142, 8.182291666325268054, 0.7511620957034663704 ) ) ;
#3164=CARTESIAN_POINT ( 'NONE',  ( -62.49999999999998579, 15.80208333265053788, 0.6339745962155627357 ) ) ;
#3166=CARTESIAN_POINT ( 'NONE',  ( -61.56765823437498852, 12.09895833299193413, 2.248837904296538515 ) ) ;
#3168=CARTESIAN_POINT ( 'NONE',  ( -61.99999999999998579, 9.156249999317203958, 2.500000000000002665 ) ) ;
#3169=ORIENTED_EDGE ( 'NONE', *, *, #5271, .T. ) ;
#3170=CARTESIAN_POINT ( 'NONE',  ( -60.99999999999998579, 9.218749999317203958, 1.500000000000002220 ) ) ;
#3171=AXIS2_PLACEMENT_3D ( 'NONE', #861, #10972, #4243 ) ;
#3173=FACE_OUTER_BOUND ( 'NONE', #1689, .T. ) ;
#3174=CARTESIAN_POINT ( 'NONE',  ( -61.99999999999998579, 14.26562499965860020, 2.498450539062049724 ) ) ;
#3178=CARTESIAN_POINT ( 'NONE',  ( -62.86468353124998032, 10.99479166632526628, 1.000774730468978024 ) ) ;
#3179=CARTESIAN_POINT ( 'NONE',  ( -62.43234176562498305, 15.72395833299193590, 0.7511620957034662593 ) ) ;
#3182=FACE_OUTER_BOUND ( 'NONE', #5830, .T. ) ;
#3183=CARTESIAN_POINT ( 'NONE',  ( -60.99999999999998579, 15.46874999931720218, 1.500000000000002220 ) ) ;
#3185=ORIENTED_EDGE ( 'NONE', *, *, #5664, .T. ) ;
#3186=CARTESIAN_POINT ( 'NONE',  ( -61.99999999999997868, 8.281249999317202182, 0.5000000000000013323 ) ) ;
#3187=CARTESIAN_POINT ( 'NONE',  ( -62.49999999999998579, 12.66666666666666607, 2.366025403784441483 ) ) ;
#3191=CARTESIAN_POINT ( 'NONE',  ( -61.13531646874997705, 14.30729166632526983, 1.999225269531026417 ) ) ;
#3192=CARTESIAN_POINT ( 'NONE',  ( -61.99999999999998579, 9.265624999658600203, 2.498450539062049724 ) ) ;
#3193=CARTESIAN_POINT ( 'NONE',  ( -60.99999999999998579, 14.44791666598387003, 2.077350269189628840 ) ) ;
#3195=CARTESIAN_POINT ( 'NONE',  ( -61.99999999999998579, 13.81249999999999822, 0.3452994616207497591 ) ) ;
#3196=CARTESIAN_POINT ( 'NONE',  ( -60.99999999999998579, 8.979166666666666075, 2.077350269189628840 ) ) ;
#3197=VECTOR ( 'NONE', #5882, 1000.000000000000000 ) ;
#3198=SURFACE_STYLE_FILL_AREA ( #7579 ) ;
#3199=CARTESIAN_POINT ( 'NONE',  ( -62.99999999999998579, 12.34374999931720218, 1.500000000000001998 ) ) ;
#3200=CARTESIAN_POINT ( 'NONE',  ( -60.99999999999998579, 9.520833333333333925, 0.9226497308103762673 ) ) ;
#3201=CARTESIAN_POINT ( 'NONE',  ( -62.43234176562499016, 14.49479166632526983, 2.248837904296538071 ) ) ;
#3202=CARTESIAN_POINT ( 'NONE',  ( -61.49999999999998579, 11.45833333333333393, 2.366025403784441927 ) ) ;
#3204=CARTESIAN_POINT ( 'NONE',  ( -62.43234176562499016, 12.05729166632526628, 2.248837904296538071 ) ) ;
#3205=DIRECTION ( 'NONE',  ( 0.000000000000000000, 0.000000000000000000, -1.000000000000000000 ) ) ;
#3206=CARTESIAN_POINT ( 'NONE',  ( -62.43234176562499016, 15.30729166632526805, 2.248837904296538071 ) ) ;
#3207=ORIENTED_EDGE ( 'NONE', *, *, #3571, .T. ) ;
#3208=DIRECTION ( 'NONE',  ( -0.000000000000000000, -1.000000000000000000, -0.000000000000000000 ) ) ;
#3210=CARTESIAN_POINT ( 'NONE',  ( -61.49999999999998579, 9.708333333333332149, 2.366025403784441927 ) ) ;
#3211=CARTESIAN_POINT ( 'NONE',  ( -61.73205080756886787, 8.551335450315370679, 0.5000000000000036637 ) ) ;
#3212=CYLINDRICAL_SURFACE ( 'NONE', #6186, 0.9999999999999981126 ) ;
#3213=ADVANCED_FACE ( 'NONE', ( #9587 ), #4525, .T. ) ;
#3215=CARTESIAN_POINT ( 'NONE',  ( -61.99999999999998579, 11.82812499965860198, 2.498450539062049724 ) ) ;
#3219=CARTESIAN_POINT ( 'NONE',  ( -61.49999999999998579, 13.67708333265053433, 2.366025403784441927 ) ) ;
#3220=CARTESIAN_POINT ( 'NONE',  ( -62.86468353124998032, 13.93229166632526805, 1.000774730468978246 ) ) ;
#3221=EDGE_CURVE ( 'NONE', #381, #2581, #8403, .T. ) ;
#3222=DIRECTION ( 'NONE',  ( -0.000000000000000000, -1.000000000000000000, -0.000000000000000000 ) ) ;
#3223=CARTESIAN_POINT ( 'NONE',  ( -61.49999999999998579, 14.54166666666666607, 0.6339745962155628467 ) ) ;
#3226=CARTESIAN_POINT ( 'NONE',  ( -62.43234176562498305, 13.22395833299193413, 0.7511620957034662593 ) ) ;
#3227=CARTESIAN_POINT ( 'NONE',  ( -61.13531646874998415, 15.86979166632526628, 1.999225269531026417 ) ) ;
#3228=CARTESIAN_POINT ( 'NONE',  ( -61.99999999999997868, 8.062500000000000000, 0.5000000000000013323 ) ) ;
#3230=CARTESIAN_POINT ( 'NONE',  ( -62.49999999999998579, 15.16666666666666607, 2.366025403784441483 ) ) ;
#3231=CARTESIAN_POINT ( 'NONE',  ( -62.43234176562499016, 8.307291666325268054, 2.248837904296538071 ) ) ;
#3235=( BOUNDED_CURVE ( )  B_SPLINE_CURVE ( 2, ( #6354, #2857, #6243, #3800, #2194, #6417, #2023, #5572, #9741 ),
 .UNSPECIFIED., .F., .T. ) 
 B_SPLINE_CURVE_WITH_KNOTS ( ( 3, 2, 2, 2, 3 ),
 ( 0.07031249999999995837, 0.07291666666666667129, 0.07812500000000000000, 0.08333333333333332871, 0.08593750000000000000 ),
 .UNSPECIFIED. ) 
 CURVE ( )  GEOMETRIC_REPRESENTATION_ITEM ( )  RATIONAL_B_SPLINE_CURVE ( ( 0.9330127018922194093, 0.9330127018922182991, 1.000000000000000000, 0.8660254037844387076, 1.000000000000000000, 0.8660254037844387076, 1.000000000000000000, 0.9330127018922194093, 0.9330127018922194093 ) ) 
 REPRESENTATION_ITEM ( '' )  );
#3236=AXIS2_PLACEMENT_3D ( 'NONE', #3517, #1860, #8635 ) ;
#3238=VECTOR ( 'NONE', #9626, 1000.000000000000000 ) ;
#3239=CARTESIAN_POINT ( 'NONE',  ( -61.99999999999999289, 13.64062499965860198, 0.5015494609379544944 ) ) ;
#3240=CARTESIAN_POINT ( 'NONE',  ( -61.56765823437498852, 9.286458332991935904, 2.248837904296538515 ) ) ;
#3242=CARTESIAN_POINT ( 'NONE',  ( -62.86468353124999453, 16.01562499965860198, 1.500000000000002220 ) ) ;
#3245=CARTESIAN_POINT ( 'NONE',  ( -60.99999999999998579, 13.27083333333333215, 0.9226497308103762673 ) ) ;
#3247=CARTESIAN_POINT ( 'NONE',  ( -62.86468353124999453, 9.286458332991934128, 1.999225269531025750 ) ) ;
#3250=EDGE_CURVE ( 'NONE', #9814, #2202, #8336, .T. ) ;
#3251=CARTESIAN_POINT ( 'NONE',  ( -61.99999999999998579, 11.65624999931720218, 2.654700538379254571 ) ) ;
#3255=CARTESIAN_POINT ( 'NONE',  ( -62.86468353124998742, 14.22395833299193590, 1.999225269531025972 ) ) ;
#3258=CARTESIAN_POINT ( 'NONE',  ( -62.86468353124998032, 12.24479166632526805, 1.000774730468978246 ) ) ;
#3259=CYLINDRICAL_SURFACE ( 'NONE', #2299, 0.9999999999999981126 ) ;
#3260=EDGE_CURVE ( 'NONE', #381, #3952, #10359, .T. ) ;
#3263=CARTESIAN_POINT ( 'NONE',  ( -61.99999999999998579, 14.68750000000000000, 2.500000000000002665 ) ) ;
#3265=EDGE_CURVE ( 'NONE', #4030, #6875, #8059, .T. ) ;
#3267=CARTESIAN_POINT ( 'NONE',  ( -61.73205080756884655, 8.667414549001829727, 2.500000000000004885 ) ) ;
#3268=CARTESIAN_POINT ( 'NONE',  ( -60.99999999999998579, 11.47916666666666607, 2.077350269189628840 ) ) ;
#3269=DIRECTION ( 'NONE',  ( -0.000000000000000000, -1.000000000000000000, -0.000000000000000000 ) ) ;
#3270=LINE ( 'NONE', #4151, #4043 ) ;
#3272=EDGE_CURVE ( 'NONE', #7919, #7344, #9179, .T. ) ;
#3273=CARTESIAN_POINT ( 'NONE',  ( -61.49999999999998579, 8.677083332650536107, 2.366025403784441927 ) ) ;
#3274=CARTESIAN_POINT ( 'NONE',  ( -62.86468353124999453, 13.76562499965860198, 1.500000000000002220 ) ) ;
#3277=CARTESIAN_POINT ( 'NONE',  ( -61.99999999999998579, 16.00000000000000000, 2.500000000000000444 ) ) ;
#3278=EDGE_CURVE ( 'NONE', #10979, #7075, #10304, .T. ) ;
#3279=EDGE_LOOP ( 'NONE', ( #2969, #10216, #1655, #1072 ) ) ;
#3280=CARTESIAN_POINT ( 'NONE',  ( -61.73205080756886076, 13.77008544963257464, 0.5000000000000014433 ) ) ;
#3281=CARTESIAN_POINT ( 'NONE',  ( -61.13531646874998415, 15.59895833299193590, 1.000774730468978468 ) ) ;
#3282=CARTESIAN_POINT ( 'NONE',  ( -62.99999999999998579, 11.89583333333333215, 2.077350269189627952 ) ) ;
#3283=CARTESIAN_POINT ( 'NONE',  ( -61.49999999999998579, 11.76041666598387003, 0.6339745962155628467 ) ) ;
#3285=CARTESIAN_POINT ( 'NONE',  ( -61.99999999999999289, 12.32812499965860198, 2.498450539062049724 ) ) ;
#3286=CARTESIAN_POINT ( 'NONE',  ( -62.86468353124998742, 15.53645833299193590, 1.999225269531025972 ) ) ;
#3287=CARTESIAN_POINT ( 'NONE',  ( -62.26794919243111082, 14.29241454900183328, 0.5000000000000013323 ) ) ;
#3288=LINE ( 'NONE', #10269, #3704 ) ;
#3289=CARTESIAN_POINT ( 'NONE',  ( -60.99999999999998579, 15.98958333265053433, 0.9226497308103762673 ) ) ;
#3292=CARTESIAN_POINT ( 'NONE',  ( -62.26794919243111082, 11.79241454900183328, 0.5000000000000013323 ) ) ;
#3294=CARTESIAN_POINT ( 'NONE',  ( -61.99999999999999289, 13.89062499965860198, 0.5015494609379544944 ) ) ;
#3295=CARTESIAN_POINT ( 'NONE',  ( -62.86468353124999453, 10.20312499965860198, 1.500000000000002220 ) ) ;
#3296=CARTESIAN_POINT ( 'NONE',  ( -61.56765823437498142, 15.43229166632526805, 0.7511620957034663704 ) ) ;
#3299=CARTESIAN_POINT ( 'NONE',  ( -62.49999999999998579, 13.16666666666666607, 2.366025403784441483 ) ) ;
#3300=CARTESIAN_POINT ( 'NONE',  ( -61.99999999999999289, 8.953124999658601979, 0.5015494609379544944 ) ) ;
#3302=CARTESIAN_POINT ( 'NONE',  ( -62.99999999999998579, 12.11458333265053611, 2.077350269189627952 ) ) ;
#3303=( BOUNDED_CURVE ( )  B_SPLINE_CURVE ( 2, ( #4545, #7951, #3721, #7119, #3112 ),
 .UNSPECIFIED., .F., .T. ) 
 B_SPLINE_CURVE_WITH_KNOTS ( ( 3, 2, 3 ),
 ( 0.9921875000000000000, 0.9947916666666666297, 1.000000000000000000 ),
 .UNSPECIFIED. ) 
 CURVE ( )  GEOMETRIC_REPRESENTATION_ITEM ( )  RATIONAL_B_SPLINE_CURVE ( ( 0.9330127018922194093, 0.9330127018922194093, 1.000000000000000000, 0.8660254037844387076, 1.000000000000000000 ) ) 
 REPRESENTATION_ITEM ( '' )  );
#3306=CARTESIAN_POINT ( 'NONE',  ( -62.43234176562498305, 13.66145833299193413, 0.7511620957034662593 ) ) ;
#3307=ORIENTED_EDGE ( 'NONE', *, *, #8457, .T. ) ;
#3308=CARTESIAN_POINT ( 'NONE',  ( -61.99999999999998579, 12.32812499965860376, 2.498450539062049724 ) ) ;
#3311=ORIENTED_EDGE ( 'NONE', *, *, #2165, .T. ) ;
#3312=CARTESIAN_POINT ( 'NONE',  ( -61.99999999999998579, 12.31249999999999822, 0.5000000000000013323 ) ) ;
#3313=EDGE_CURVE ( 'NONE', #4238, #6626, #742, .T. ) ;
#3315=CARTESIAN_POINT ( 'NONE',  ( -62.99999999999998579, 11.64583333333333748, 2.077350269189627952 ) ) ;
#3318=CARTESIAN_POINT ( 'NONE',  ( -62.43234176562498305, 8.473958332991934128, 0.7511620957034662593 ) ) ;
#3320=CARTESIAN_POINT ( 'NONE',  ( -61.56765823437498852, 13.09895833299193413, 2.248837904296538515 ) ) ;
#3323=CARTESIAN_POINT ( 'NONE',  ( -61.73205080756886076, 11.02008544963257108, 0.5000000000000014433 ) ) ;
#3324=VECTOR ( 'NONE', #6525, 1000.000000000000000 ) ;
#3325=ORIENTED_EDGE ( 'NONE', *, *, #4423, .T. ) ;
#3326=CARTESIAN_POINT ( 'NONE',  ( -60.99999999999998579, 12.72916666666666607, 2.077350269189628840 ) ) ;
#3327=CARTESIAN_POINT ( 'NONE',  ( -62.43234176562498305, 15.41145833299193590, 0.7511620957034662593 ) ) ;
#3329=CARTESIAN_POINT ( 'NONE',  ( -61.99999999999999289, 12.95312499965860020, 0.5015494609379544944 ) ) ;
#3330=CARTESIAN_POINT ( 'NONE',  ( -62.43234176562499016, 15.55729166632526628, 2.248837904296538071 ) ) ;
#3331=CARTESIAN_POINT ( 'NONE',  ( -61.73205080756885366, 9.301335450315368902, 0.5000000000000028866 ) ) ;
#3332=DIRECTION ( 'NONE',  ( -0.000000000000000000, -1.000000000000000000, -0.000000000000000000 ) ) ;
#3333=ADVANCED_FACE ( 'NONE', ( #6435 ), #7316, .F. ) ;
#3334=CARTESIAN_POINT ( 'NONE',  ( -62.43234176562498305, 8.723958332991934128, 0.7511620957034662593 ) ) ;
#3341=CARTESIAN_POINT ( 'NONE',  ( -62.86468353124998032, 13.68229166632526805, 1.000774730468978024 ) ) ;
#3342=CARTESIAN_POINT ( 'NONE',  ( -62.86468353124998032, 11.68229166632526805, 1.000774730468978246 ) ) ;
#3343=CARTESIAN_POINT ( 'NONE',  ( -61.56765823437498852, 15.84895833299193590, 2.248837904296538515 ) ) ;
#3345=CARTESIAN_POINT ( 'NONE',  ( -61.99999999999998579, 13.18750000000000000, 2.500000000000002665 ) ) ;
#3346=EDGE_LOOP ( 'NONE', ( #8949, #6351, #6657, #9985 ) ) ;
#3347=CARTESIAN_POINT ( 'NONE',  ( -62.99999999999998579, 15.14583333333333215, 2.077350269189627952 ) ) ;
#3348=CARTESIAN_POINT ( 'NONE',  ( -62.43234176562498305, 8.223958332991934128, 0.7511620957034662593 ) ) ;
#3349=( NAMED_UNIT ( * ) PLANE_ANGLE_UNIT ( ) SI_UNIT ( $, .RADIAN. ) );
#3350=CARTESIAN_POINT ( 'NONE',  ( -61.99999999999998579, 13.53124999931720218, 0.3452994616207497591 ) ) ;
#3351=ORIENTED_EDGE ( 'NONE', *, *, #1326, .F. ) ;
#3354=CARTESIAN_POINT ( 'NONE',  ( -62.86468353124998032, 14.18229166632526983, 1.000774730468978246 ) ) ;
#3360=CARTESIAN_POINT ( 'NONE',  ( -61.56765823437498142, 12.68229166632526805, 0.7511620957034663704 ) ) ;
#3361=( BOUNDED_CURVE ( )  B_SPLINE_CURVE ( 2, ( #7632, #10343, #17, #4387, #4451, #3622, #6013, #9400, #7017 ),
 .UNSPECIFIED., .F., .T. ) 
 B_SPLINE_CURVE_WITH_KNOTS ( ( 3, 2, 2, 2, 3 ),
 ( 0.1796875000000000555, 0.1822916666666666574, 0.1875000000000000000, 0.1927083333333333426, 0.1953124999999999445 ),
 .UNSPECIFIED. ) 
 CURVE ( )  GEOMETRIC_REPRESENTATION_ITEM ( )  RATIONAL_B_SPLINE_CURVE ( ( 0.9330127018922192983, 0.9330127018922207416, 1.000000000000000000, 0.8660254037844387076, 1.000000000000000000, 0.8660254037844387076, 1.000000000000000000, 0.9330127018922207416, 0.9330127018922192983 ) ) 
 REPRESENTATION_ITEM ( '' )  );
#3363=VERTEX_POINT ( 'NONE', #1531 ) ;
#3367=CARTESIAN_POINT ( 'NONE',  ( -61.73205080756886076, 14.69866454968463110, 2.500000000000003109 ) ) ;
#3369=CARTESIAN_POINT ( 'NONE',  ( -62.99999999999998579, 11.60416666666666785, 0.9226497308103756012 ) ) ;
#3371=CARTESIAN_POINT ( 'NONE',  ( -61.13531646874998415, 9.369791666325268054, 1.999225269531026417 ) ) ;
#3372=CARTESIAN_POINT ( 'NONE',  ( -61.73205080756886076, 10.41741454900183328, 2.500000000000003109 ) ) ;
#3374=CARTESIAN_POINT ( 'NONE',  ( -62.86468353124998032, 13.24479166632526983, 1.000774730468978246 ) ) ;
#3378=EDGE_LOOP ( 'NONE', ( #6303, #2085, #4168, #1806 ) ) ;
#3380=CARTESIAN_POINT ( 'NONE',  ( -61.56765823437498852, 15.03645833299193590, 2.248837904296538515 ) ) ;
#3382=DIRECTION ( 'NONE',  ( 0.000000000000000000, 1.000000000000000000, 0.000000000000000000 ) ) ;
#3383=CARTESIAN_POINT ( 'NONE',  ( -61.99999999999999289, 12.07812499965860198, 2.498450539062049724 ) ) ;
#3384=CARTESIAN_POINT ( 'NONE',  ( -62.43234176562499016, 9.494791666325268054, 2.248837904296538071 ) ) ;
#3387=AXIS2_PLACEMENT_3D ( 'NONE', #6862, #1140, #5290 ) ;
#3388=CARTESIAN_POINT ( 'NONE',  ( -61.99999999999998579, 9.578124999658601979, 2.498450539062049724 ) ) ;
#3389=CYLINDRICAL_SURFACE ( 'NONE', #8028, 0.9999999999999981126 ) ;
#3390=ORIENTED_EDGE ( 'NONE', *, *, #3571, .F. ) ;
#3391=CARTESIAN_POINT ( 'NONE',  ( -61.99999999999998579, 8.656249999317202182, 2.500000000000002665 ) ) ;
#3393=CARTESIAN_POINT ( 'NONE',  ( -61.99999999999998579, 11.26562499965860198, 2.498450539062049724 ) ) ;
#3394=CARTESIAN_POINT ( 'NONE',  ( -62.86468353124998032, 15.99479166632526628, 1.000774730468978024 ) ) ;
#3397=CARTESIAN_POINT ( 'NONE',  ( -62.49999999999998579, 15.41666666666666607, 2.366025403784441483 ) ) ;
#3398=CARTESIAN_POINT ( 'NONE',  ( -62.86468353124999453, 8.515624999658601979, 1.500000000000002220 ) ) ;
#3400=CARTESIAN_POINT ( 'NONE',  ( -61.49999999999998579, 13.92708333265053611, 2.366025403784441927 ) ) ;
#3401=CARTESIAN_POINT ( 'NONE',  ( -62.99999999999998579, 13.10416666666666607, 0.9226497308103756012 ) ) ;
#3403=EDGE_CURVE ( 'NONE', #3446, #470, #6124, .T. ) ;
#3406=DIRECTION ( 'NONE',  ( -0.000000000000000000, -1.000000000000000000, -0.000000000000000000 ) ) ;
#3407=CARTESIAN_POINT ( 'NONE',  ( -61.13531646874997705, 11.55729166632526628, 1.999225269531026417 ) ) ;
#3408=EDGE_CURVE ( 'NONE', #607, #9265, #10677, .T. ) ;
#3414=CARTESIAN_POINT ( 'NONE',  ( -61.13531646874998415, 12.89062499965860198, 1.500000000000002220 ) ) ;
#3415=DIRECTION ( 'NONE',  ( 0.000000000000000000, 0.000000000000000000, -1.000000000000000000 ) ) ;
#3416=ORIENTED_EDGE ( 'NONE', *, *, #7660, .T. ) ;
#3420=AXIS2_PLACEMENT_3D ( 'NONE', #6348, #8910, #1403 ) ;
#3422=CARTESIAN_POINT ( 'NONE',  ( -61.13531646874998415, 11.30729166632526805, 1.999225269531026417 ) ) ;
#3423=( BOUNDED_CURVE ( )  B_SPLINE_CURVE ( 2, ( #9013, #1406, #4784, #8189, #575, #6782, #4314, #102, #778 ),
 .UNSPECIFIED., .F., .T. ) 
 B_SPLINE_CURVE_WITH_KNOTS ( ( 3, 2, 2, 2, 3 ),
 ( 0.7421875000000000000, 0.7447916666666666297, 0.7500000000000000000, 0.7552083333333333703, 0.7578125000000000000 ),
 .UNSPECIFIED. ) 
 CURVE ( )  GEOMETRIC_REPRESENTATION_ITEM ( )  RATIONAL_B_SPLINE_CURVE ( ( 0.9330127018922194093, 0.9330127018922194093, 1.000000000000000000, 0.8660254037844387076, 1.000000000000000000, 0.8660254037844387076, 1.000000000000000000, 0.9330127018922194093, 0.9330127018922194093 ) ) 
 REPRESENTATION_ITEM ( '' )  );
#3424=ORIENTED_EDGE ( 'NONE', *, *, #4417, .T. ) ;
#3425=CARTESIAN_POINT ( 'NONE',  ( -62.86468353124998032, 8.994791666325268054, 1.000774730468978246 ) ) ;
#3426=CARTESIAN_POINT ( 'NONE',  ( -61.99999999999998579, 13.78124999931720218, 0.5000000000000013323 ) ) ;
#3428=EDGE_CURVE ( 'NONE', #9081, #4762, #10340, .T. ) ;
#3429=CARTESIAN_POINT ( 'NONE',  ( -61.56765823437498142, 13.18229166632526805, 0.7511620957034663704 ) ) ;
#3432=CARTESIAN_POINT ( 'NONE',  ( -60.99999999999998579, 10.98958333265053611, 0.9226497308103762673 ) ) ;
#3433=EDGE_CURVE ( 'NONE', #9779, #869, #4977, .T. ) ;
#3435=CARTESIAN_POINT ( 'NONE',  ( -62.99999999999998579, 11.61458333265053611, 2.077350269189627952 ) ) ;
#3436=CARTESIAN_POINT ( 'NONE',  ( -61.13531646874998415, 15.84895833299193413, 1.000774730468978468 ) ) ;
#3437=CARTESIAN_POINT ( 'NONE',  ( -61.99999999999998579, 16.03124999931720041, 0.5000000000000013323 ) ) ;
#3438=CARTESIAN_POINT ( 'NONE',  ( -61.73205080756886076, 12.52008544963257464, 0.5000000000000014433 ) ) ;
#3440=CARTESIAN_POINT ( 'NONE',  ( -62.86468353124998032, 12.49479166632526628, 1.000774730468978024 ) ) ;
#3441=CARTESIAN_POINT ( 'NONE',  ( -61.56765823437498852, 8.286458332991934128, 2.248837904296538515 ) ) ;
#3442=CARTESIAN_POINT ( 'NONE',  ( -60.99999999999998579, 9.229166666666667851, 2.077350269189628840 ) ) ;
#3444=CARTESIAN_POINT ( 'NONE',  ( -62.86468353124998032, 9.744791666325268054, 1.000774730468978246 ) ) ;
#3445=CYLINDRICAL_SURFACE ( 'NONE', #8211, 0.9999999999999981126 ) ;
#3446=VERTEX_POINT ( 'NONE', #348 ) ;
#3447=CARTESIAN_POINT ( 'NONE',  ( -61.13531646874998415, 16.10937499965860198, 1.500000000000002220 ) ) ;
#3449=CARTESIAN_POINT ( 'NONE',  ( -61.13531646874998415, 15.32812499965860020, 1.500000000000002220 ) ) ;
#3451=CARTESIAN_POINT ( 'NONE',  ( -62.43234176562498305, 10.66145833299193413, 0.7511620957034662593 ) ) ;
#3452=CARTESIAN_POINT ( 'NONE',  ( -61.56765823437498142, 15.93229166632526628, 0.7511620957034663704 ) ) ;
#3453=FACE_OUTER_BOUND ( 'NONE', #2497, .T. ) ;
#3454=ORIENTED_EDGE ( 'NONE', *, *, #722, .T. ) ;
#3455=CARTESIAN_POINT ( 'NONE',  ( -60.99999999999998579, 15.00000000000000000, 1.500000000000002220 ) ) ;
#3456=CARTESIAN_POINT ( 'NONE',  ( -62.43234176562499016, 8.307291666325268054, 2.248837904296538071 ) ) ;
#3457=( BOUNDED_CURVE ( )  B_SPLINE_CURVE ( 2, ( #5703, #3935, #4706, #8994, #653, #9989, #6554, #10597, #9153 ),
 .UNSPECIFIED., .F., .F. ) 
 B_SPLINE_CURVE_WITH_KNOTS ( ( 3, 2, 2, 2, 3 ),
 ( 0.4921875000000000000, 0.4947916666666666852, 0.5000000000000000000, 0.5052083333333333703, 0.5078125000000000000 ),
 .UNSPECIFIED. ) 
 CURVE ( )  GEOMETRIC_REPRESENTATION_ITEM ( )  RATIONAL_B_SPLINE_CURVE ( ( 0.9330127018922194093, 0.9330127018922194093, 1.000000000000000000, 0.8660254037844387076, 1.000000000000000000, 0.8660254037844387076, 1.000000000000000000, 0.9330127018922194093, 0.9330127018922194093 ) ) 
 REPRESENTATION_ITEM ( '' )  );
#3459=CARTESIAN_POINT ( 'NONE',  ( -62.99999999999998579, 13.34374999931720396, 1.500000000000001998 ) ) ;
#3461=CARTESIAN_POINT ( 'NONE',  ( -61.99999999999998579, 9.312500000000000000, 0.5000000000000013323 ) ) ;
#3462=CARTESIAN_POINT ( 'NONE',  ( -61.13531646874997705, 11.59895833299193590, 1.000774730468978468 ) ) ;
#3464=EDGE_CURVE ( 'NONE', #10295, #7075, #8798, .T. ) ;
#3465=CARTESIAN_POINT ( 'NONE',  ( -62.99999999999998579, 8.354166666666666075, 0.9226497308103756012 ) ) ;
#3466=ORIENTED_EDGE ( 'NONE', *, *, #10336, .T. ) ;
#3468=CARTESIAN_POINT ( 'NONE',  ( -62.86468353124999453, 13.26562499965860198, 1.500000000000002220 ) ) ;
#3470=CARTESIAN_POINT ( 'NONE',  ( -60.99999999999998579, 11.44791666598387003, 2.077350269189628840 ) ) ;
#3471=CARTESIAN_POINT ( 'NONE',  ( -62.99999999999998579, 8.822916665983868256, 0.9226497308103756012 ) ) ;
#3476=CARTESIAN_POINT ( 'NONE',  ( -61.99999999999998579, 14.81250000000000000, 0.5000000000000013323 ) ) ;
#3477=CARTESIAN_POINT ( 'NONE',  ( -62.43234176562499016, 11.24479166632526805, 2.248837904296538071 ) ) ;
#3478=VERTEX_POINT ( 'NONE', #1180 ) ;
#3479=CARTESIAN_POINT ( 'NONE',  ( -61.99999999999998579, 8.328124999658601979, 2.498450539062049724 ) ) ;
#3480=CARTESIAN_POINT ( 'NONE',  ( -62.99999999999998579, 15.87500000000000000, 1.500000000000001998 ) ) ;
#3482=CARTESIAN_POINT ( 'NONE',  ( -61.56765823437498852, 13.34895833299193413, 2.248837904296538515 ) ) ;
#3483=CARTESIAN_POINT ( 'NONE',  ( -62.49999999999998579, 9.385416665983870033, 2.366025403784441483 ) ) ;
#3486=ORIENTED_EDGE ( 'NONE', *, *, #8180, .T. ) ;
#3487=CARTESIAN_POINT ( 'NONE',  ( -60.99999999999998579, 12.77083333333333393, 0.9226497308103762673 ) ) ;
#3488=CARTESIAN_POINT ( 'NONE',  ( -61.13531646874998415, 15.34895833299193590, 1.000774730468978468 ) ) ;
#3489=CYLINDRICAL_SURFACE ( 'NONE', #7347, 0.9999999999999981126 ) ;
#3490=CARTESIAN_POINT ( 'NONE',  ( -60.99999999999998579, 8.218749999317202182, 1.500000000000002220 ) ) ;
#3492=CARTESIAN_POINT ( 'NONE',  ( -62.43234176562499016, 14.05729166632526805, 2.248837904296538071 ) ) ;
#3493=CARTESIAN_POINT ( 'NONE',  ( -61.13531646874998415, 9.078124999658601979, 1.500000000000002220 ) ) ;
#3494=EDGE_CURVE ( 'NONE', #3891, #381, #7276, .T. ) ;
#3498=CARTESIAN_POINT ( 'NONE',  ( -62.86468353124999453, 9.265624999658600203, 1.500000000000002220 ) ) ;
#3499=DIRECTION ( 'NONE',  ( -0.000000000000000000, -1.000000000000000000, -0.000000000000000000 ) ) ;
#3502=DIRECTION ( 'NONE',  ( 0.000000000000000000, 0.000000000000000000, -1.000000000000000000 ) ) ;
#3503=CARTESIAN_POINT ( 'NONE',  ( -62.86468353124999453, 15.20312499965860020, 1.500000000000002220 ) ) ;
#3504=CARTESIAN_POINT ( 'NONE',  ( -61.56765823437498852, 11.03645833299193590, 2.248837904296538515 ) ) ;
#3506=CARTESIAN_POINT ( 'NONE',  ( -61.13531646874997705, 8.848958332991934128, 1.000774730468978468 ) ) ;
#3509=CARTESIAN_POINT ( 'NONE',  ( -62.99999999999998579, 14.87500000000000000, 1.500000000000001998 ) ) ;
#3511=CARTESIAN_POINT ( 'NONE',  ( -62.43234176562498305, 9.723958332991934128, 0.7511620957034662593 ) ) ;
#3513=CARTESIAN_POINT ( 'NONE',  ( -62.99999999999998579, 13.09374999931720396, 1.500000000000001998 ) ) ;
#3516=EDGE_CURVE ( 'NONE', #5370, #8255, #2308, .T. ) ;
#3517=CARTESIAN_POINT ( 'NONE',  ( -61.99999999999998579, 16.00000000000000000, 1.500000000000002220 ) ) ;
#3519=AXIS2_PLACEMENT_3D ( 'NONE', #834, #6792, #2506 ) ;
#3520=CARTESIAN_POINT ( 'NONE',  ( -62.43234176562499016, 10.99479166632526805, 2.248837904296538071 ) ) ;
#3521=CARTESIAN_POINT ( 'NONE',  ( -62.49999999999998579, 15.58333333333333393, 0.6339745962155627357 ) ) ;
#3522=CARTESIAN_POINT ( 'NONE',  ( -60.99999999999998579, 13.02083333333333215, 0.9226497308103762673 ) ) ;
#3526=CARTESIAN_POINT ( 'NONE',  ( -62.86468353124998742, 12.53645833299193590, 1.999225269531025972 ) ) ;
#3528=CARTESIAN_POINT ( 'NONE',  ( -62.49999999999998579, 9.052083332650536107, 0.6339745962155627357 ) ) ;
#3532=CARTESIAN_POINT ( 'NONE',  ( -62.43234176562498305, 11.41145833299193590, 0.7511620957034662593 ) ) ;
#3535=EDGE_LOOP ( 'NONE', ( #7254, #4443, #5739, #2946 ) ) ;
#3536=CARTESIAN_POINT ( 'NONE',  ( -61.13531646874998415, 9.390624999658600203, 1.500000000000002220 ) ) ;
#3537=CARTESIAN_POINT ( 'NONE',  ( -61.99999999999998579, 15.68749999999999645, 2.500000000000002665 ) ) ;
#3538=CARTESIAN_POINT ( 'NONE',  ( -61.13531646874998415, 14.39062499965860020, 1.500000000000002220 ) ) ;
#3540=CARTESIAN_POINT ( 'NONE',  ( -61.99999999999998579, 9.406249999317202182, 2.500000000000002665 ) ) ;
#3542=LINE ( 'NONE', #1773, #9395 ) ;
#3543=ORIENTED_EDGE ( 'NONE', *, *, #9712, .T. ) ;
#3544=CARTESIAN_POINT ( 'NONE',  ( -62.99999999999998579, 10.89583333333333393, 2.077350269189627952 ) ) ;
#3545=EDGE_CURVE ( 'NONE', #3952, #6912, #9532, .T. ) ;
#3546=EDGE_CURVE ( 'NONE', #10509, #4846, #2790, .T. ) ;
#3547=CARTESIAN_POINT ( 'NONE',  ( -61.99999999999998579, 8.187500000000001776, 2.654700538379254571 ) ) ;
#3548=CARTESIAN_POINT ( 'NONE',  ( -61.99999999999998579, 9.937500000000000000, 2.500000000000002665 ) ) ;
#3550=CARTESIAN_POINT ( 'NONE',  ( -62.26794919243111082, 12.29241454900182973, 0.5000000000000013323 ) ) ;
#3551=CARTESIAN_POINT ( 'NONE',  ( -62.43234176562498305, 13.72395833299193413, 0.7511620957034662593 ) ) ;
#3552=CARTESIAN_POINT ( 'NONE',  ( -62.86468353124999453, 9.453124999658600203, 1.500000000000002220 ) ) ;
#3553=FACE_OUTER_BOUND ( 'NONE', #4990, .T. ) ;
#3555=CARTESIAN_POINT ( 'NONE',  ( -62.43234176562499016, 9.557291666325268054, 2.248837904296538071 ) ) ;
#3556=DIRECTION ( 'NONE',  ( -0.000000000000000000, -1.000000000000000000, -0.000000000000000000 ) ) ;
#3559=DIRECTION ( 'NONE',  ( -0.000000000000000000, -1.000000000000000000, -0.000000000000000000 ) ) ;
#3560=CARTESIAN_POINT ( 'NONE',  ( -61.13531646874998415, 16.07812499965860198, 1.500000000000002220 ) ) ;
#3561=CARTESIAN_POINT ( 'NONE',  ( -61.56765823437498142, 11.11979166632526805, 0.7511620957034663704 ) ) ;
#3562=CARTESIAN_POINT ( 'NONE',  ( -62.86468353124998032, 8.932291666325268054, 1.000774730468978024 ) ) ;
#3564=CARTESIAN_POINT ( 'NONE',  ( -60.99999999999998579, 14.75000000000000000, 1.500000000000002220 ) ) ;
#3565=CARTESIAN_POINT ( 'NONE',  ( -62.86468353124999453, 10.51562499965860198, 1.500000000000002220 ) ) ;
#3567=CARTESIAN_POINT ( 'NONE',  ( -62.43234176562498305, 14.91145833299193590, 0.7511620957034662593 ) ) ;
#3568=CARTESIAN_POINT ( 'NONE',  ( -61.49999999999998579, 13.17708333265053433, 2.366025403784441927 ) ) ;
#3571=EDGE_CURVE ( 'NONE', #6912, #5370, #1878, .T. ) ;
#3574=CARTESIAN_POINT ( 'NONE',  ( -61.56765823437498142, 11.36979166632526805, 0.7511620957034663704 ) ) ;
#3575=CARTESIAN_POINT ( 'NONE',  ( -62.49999999999998579, 15.66666666666666607, 2.366025403784441483 ) ) ;
#3576=ORIENTED_EDGE ( 'NONE', *, *, #3221, .F. ) ;
#3577=CARTESIAN_POINT ( 'NONE',  ( -61.99999999999998579, 10.68750000000000000, 2.654700538379254571 ) ) ;
#3579=CARTESIAN_POINT ( 'NONE',  ( -60.99999999999997868, 15.98350424826734262, 1.091118259053310835 ) ) ;
#3580=CARTESIAN_POINT ( 'NONE',  ( -62.86468353124999453, 14.01562499965860198, 1.500000000000002220 ) ) ;
#3584=CARTESIAN_POINT ( 'NONE',  ( -62.99999999999998579, 8.864583332650536107, 2.077350269189627952 ) ) ;
#3589=CARTESIAN_POINT ( 'NONE',  ( -61.56765823437498852, 11.53645833299193590, 2.248837904296538515 ) ) ;
#3590=CIRCLE ( 'NONE', #6455, 0.9999999999999983347 ) ;
#3591=ORIENTED_EDGE ( 'NONE', *, *, #4946, .T. ) ;
#3593=CARTESIAN_POINT ( 'NONE',  ( -62.43234176562498305, 9.973958332991934128, 0.7511620957034662593 ) ) ;
#3596=CARTESIAN_POINT ( 'NONE',  ( -61.99999999999998579, 14.45312499965860020, 0.5015494609379544944 ) ) ;
#3598=EDGE_LOOP ( 'NONE', ( #7092, #9956, #4864, #5844 ) ) ;
#3600=ADVANCED_FACE ( 'NONE', ( #6519 ), #9171, .T. ) ;
#3601=ORIENTED_EDGE ( 'NONE', *, *, #1718, .F. ) ;
#3603=CARTESIAN_POINT ( 'NONE',  ( -61.73205080756886076, 12.66741454900183150, 2.500000000000003109 ) ) ;
#3604=CARTESIAN_POINT ( 'NONE',  ( -61.99999999999998579, 8.937500000000001776, 2.654700538379254571 ) ) ;
#3605=CARTESIAN_POINT ( 'NONE',  ( -62.99999999999998579, 9.854166666666669627, 0.9226497308103756012 ) ) ;
#3609=CARTESIAN_POINT ( 'NONE',  ( -62.86468353124999453, 14.53645833299193413, 1.999225269531025750 ) ) ;
#3610=CARTESIAN_POINT ( 'NONE',  ( -61.99999999999998579, 8.890624999658601979, 0.5015494609379544944 ) ) ;
#3611=CARTESIAN_POINT ( 'NONE',  ( -61.73205080756886076, 11.91741454900183150, 2.500000000000003109 ) ) ;
#3613=CARTESIAN_POINT ( 'NONE',  ( -62.43234176562498305, 10.22395833299193413, 0.7511620957034662593 ) ) ;
#3614=CARTESIAN_POINT ( 'NONE',  ( -62.99999999999998579, 14.11458333265053611, 2.077350269189627952 ) ) ;
#3615=VERTEX_POINT ( 'NONE', #4836 ) ;
#3616=CARTESIAN_POINT ( 'NONE',  ( -61.99999999999998579, 14.31250000000000000, 0.5000000000000013323 ) ) ;
#3618=CARTESIAN_POINT ( 'NONE',  ( -62.26794919243111082, 11.32366454968462932, 0.5000000000000013323 ) ) ;
#3619=CARTESIAN_POINT ( 'NONE',  ( -61.99999999999998579, 15.81250000000000000, 0.5000000000000013323 ) ) ;
#3620=CARTESIAN_POINT ( 'NONE',  ( -62.86468353124998742, 11.97395833299193590, 1.999225269531025972 ) ) ;
#3621=CARTESIAN_POINT ( 'NONE',  ( -62.86468353124999453, 8.473958332991934128, 1.999225269531025750 ) ) ;
#3622=CARTESIAN_POINT ( 'NONE',  ( -60.99999999999998579, 9.739583332650536107, 0.9226497308103762673 ) ) ;
#3624=CARTESIAN_POINT ( 'NONE',  ( -62.49999999999998579, 14.08333333333333393, 0.6339745962155627357 ) ) ;
#3625=CARTESIAN_POINT ( 'NONE',  ( -62.86468353124999453, 9.765624999658601979, 1.500000000000002220 ) ) ;
#3627=CARTESIAN_POINT ( 'NONE',  ( -62.43234176562498305, 14.66145833299193413, 0.7511620957034662593 ) ) ;
#3628=CARTESIAN_POINT ( 'NONE',  ( -62.49999999999998579, 14.30208333265053611, 0.6339745962155627357 ) ) ;
#3632=CARTESIAN_POINT ( 'NONE',  ( -61.56765823437498142, 12.11979166632526628, 0.7511620957034663704 ) ) ;
#3633=CARTESIAN_POINT ( 'NONE',  ( -61.13531646874998415, 8.557291666325268054, 1.999225269531026417 ) ) ;
#3635=CARTESIAN_POINT ( 'NONE',  ( -61.49999999999998579, 11.29166666666666607, 0.6339745962155628467 ) ) ;
#3638=CARTESIAN_POINT ( 'NONE',  ( -61.56765823437498852, 13.59895833299193413, 2.248837904296538515 ) ) ;
#3640=CARTESIAN_POINT ( 'NONE',  ( -61.99999999999998579, 9.031249999317202182, 0.3452994616207497591 ) ) ;
#3644=CARTESIAN_POINT ( 'NONE',  ( -62.26794919243111082, 15.39508544963257108, 2.500000000000003109 ) ) ;
#3645=CARTESIAN_POINT ( 'NONE',  ( -62.86468353124998032, 10.93229166632526805, 1.000774730468978246 ) ) ;
#3646=DIRECTION ( 'NONE',  ( 0.000000000000000000, 0.000000000000000000, 1.000000000000000000 ) ) ;
#3647=ORIENTED_EDGE ( 'NONE', *, *, #10211, .T. ) ;
#3648=CARTESIAN_POINT ( 'NONE',  ( -61.56765823437498142, 10.18229166632526805, 0.7511620957034663704 ) ) ;
#3650=CARTESIAN_POINT ( 'NONE',  ( -62.86468353124998742, 14.53645833299193413, 1.999225269531025972 ) ) ;
#3651=LINE ( 'NONE', #10373, #2702 ) ;
#3652=ORIENTED_EDGE ( 'NONE', *, *, #1281, .T. ) ;
#3653=( BOUNDED_CURVE ( )  B_SPLINE_CURVE ( 2, ( #7341, #8076, #9789, #3065, #2179, #4045, #8234, #7449, #5716 ),
 .UNSPECIFIED., .F., .T. ) 
 B_SPLINE_CURVE_WITH_KNOTS ( ( 3, 2, 2, 2, 3 ),
 ( 0.8984375000000000000, 0.9010416666666666297, 0.9062500000000000000, 0.9114583333333333703, 0.9140625000000000000 ),
 .UNSPECIFIED. ) 
 CURVE ( )  GEOMETRIC_REPRESENTATION_ITEM ( )  RATIONAL_B_SPLINE_CURVE ( ( 0.9330127018922194093, 0.9330127018922194093, 1.000000000000000000, 0.8660254037844387076, 1.000000000000000000, 0.8660254037844387076, 1.000000000000000000, 0.9330127018922194093, 0.9330127018922194093 ) ) 
 REPRESENTATION_ITEM ( '' )  );
#3654=CARTESIAN_POINT ( 'NONE',  ( -61.99999999999998579, 16.00000000000000000, 0.5000000000000041078 ) ) ;
#3657=CARTESIAN_POINT ( 'NONE',  ( -62.49999999999998579, 15.05208333265053611, 0.6339745962155627357 ) ) ;
#3658=CARTESIAN_POINT ( 'NONE',  ( -61.99999999999998579, 8.812500000000000000, 0.3452994616207497591 ) ) ;
#3659=CARTESIAN_POINT ( 'NONE',  ( -62.49999999999998579, 9.833333333333332149, 0.6339745962155627357 ) ) ;
#3662=CARTESIAN_POINT ( 'NONE',  ( -61.56765823437498142, 14.18229166632526805, 0.7511620957034663704 ) ) ;
#3663=CARTESIAN_POINT ( 'NONE',  ( -61.13531646874998415, 9.828124999658601979, 1.500000000000002220 ) ) ;
#3666=CARTESIAN_POINT ( 'NONE',  ( -61.99999999999998579, 10.57812499965860198, 2.498450539062049724 ) ) ;
#3671=CARTESIAN_POINT ( 'NONE',  ( -62.99999999999998579, 10.36458333265053611, 2.077350269189627952 ) ) ;
#3672=CARTESIAN_POINT ( 'NONE',  ( -61.13531646874998415, 12.82812499965860198, 1.500000000000002220 ) ) ;
#3673=CARTESIAN_POINT ( 'NONE',  ( -61.56765823437498142, 9.119791666325268054, 0.7511620957034663704 ) ) ;
#3674=DIRECTION ( 'NONE',  ( 0.000000000000000000, -0.000000000000000000, 1.000000000000000000 ) ) ;
#3675=ORIENTED_EDGE ( 'NONE', *, *, #9938, .T. ) ;
#3677=CARTESIAN_POINT ( 'NONE',  ( -61.13531646874998415, 10.64062499965860198, 1.500000000000002220 ) ) ;
#3678=AXIS2_PLACEMENT_3D ( 'NONE', #439, #6441, #1331 ) ;
#3680=CARTESIAN_POINT ( 'NONE',  ( -62.86468353124998742, 14.97395833299193590, 1.999225269531025972 ) ) ;
#3681=CARTESIAN_POINT ( 'NONE',  ( -62.99999999999998579, 14.82291666598386826, 0.9226497308103756012 ) ) ;
#3682=CARTESIAN_POINT ( 'NONE',  ( -62.26794919243111082, 16.14508544963257464, 2.500000000000003109 ) ) ;
#3683=ORIENTED_EDGE ( 'NONE', *, *, #7739, .F. ) ;
#3685=ORIENTED_EDGE ( 'NONE', *, *, #8342, .F. ) ;
#3686=( GEOMETRIC_REPRESENTATION_CONTEXT ( 3 ) GLOBAL_UNCERTAINTY_ASSIGNED_CONTEXT ( ( #9614 ) ) GLOBAL_UNIT_ASSIGNED_CONTEXT ( ( #1804, #132, #78 ) ) REPRESENTATION_CONTEXT ( 'NONE', 'WORKASPACE' ) );
#3687=CARTESIAN_POINT ( 'NONE',  ( -61.13531646874998415, 12.32812499965860198, 1.500000000000002220 ) ) ;
#3688=CARTESIAN_POINT ( 'NONE',  ( -62.86468353124998742, 8.723958332991934128, 1.999225269531025972 ) ) ;
#3691=CARTESIAN_POINT ( 'NONE',  ( -62.99999999999998579, 12.39583333333333393, 2.077350269189627952 ) ) ;
#3693=CARTESIAN_POINT ( 'NONE',  ( -60.99999999999998579, 8.000000000000000000, 1.500000000000002220 ) ) ;
#3694=CARTESIAN_POINT ( 'NONE',  ( -62.43234176562498305, 13.72395833299193413, 0.7511620957034662593 ) ) ;
#3697=CARTESIAN_POINT ( 'NONE',  ( -61.99999999999998579, 10.65624999931720218, 2.654700538379254571 ) ) ;
#3699=CARTESIAN_POINT ( 'NONE',  ( -61.49999999999998579, 13.95833333333333215, 2.366025403784441927 ) ) ;
#3701=CARTESIAN_POINT ( 'NONE',  ( -61.99999999999998579, 10.03124999931720218, 0.5000000000000013323 ) ) ;
#3702=CARTESIAN_POINT ( 'NONE',  ( -62.86468353124998742, 11.97395833299193590, 1.999225269531025972 ) ) ;
#3704=VECTOR ( 'NONE', #9287, 1000.000000000000000 ) ;
#3705=EDGE_CURVE ( 'NONE', #3363, #6433, #3025, .T. ) ;
#3707=CARTESIAN_POINT ( 'NONE',  ( -61.13531646874998415, 9.640624999658601979, 1.500000000000002220 ) ) ;
#3710=CARTESIAN_POINT ( 'NONE',  ( -61.99999999999998579, 14.20312499965860198, 0.5015494609379544944 ) ) ;
#3712=ORIENTED_EDGE ( 'NONE', *, *, #3145, .T. ) ;
#3717=CARTESIAN_POINT ( 'NONE',  ( -61.99999999999998579, 16.00000000000000000, 0.5000000000000041078 ) ) ;
#3718=CARTESIAN_POINT ( 'NONE',  ( -60.99999999999998579, 8.750000000000000000, 1.500000000000002220 ) ) ;
#3721=CARTESIAN_POINT ( 'NONE',  ( -61.49999999999998579, 16.17708333265053255, 2.366025403784441927 ) ) ;
#3723=CARTESIAN_POINT ( 'NONE',  ( -61.13531646874998415, 14.39062499965860020, 1.500000000000002220 ) ) ;
#3724=ADVANCED_FACE ( 'NONE', ( #3173 ), #2339, .T. ) ;
#3725=CARTESIAN_POINT ( 'NONE',  ( -62.43234176562499016, 10.24479166632526805, 2.248837904296538071 ) ) ;
#3728=( BOUNDED_CURVE ( )  B_SPLINE_CURVE ( 2, ( #4510, #5396, #4453, #6245, #2796, #7913, #471, #8803, #7076 ),
 .UNSPECIFIED., .F., .F. ) 
 B_SPLINE_CURVE_WITH_KNOTS ( ( 3, 2, 2, 2, 3 ),
 ( 0.3203125000000000000, 0.3229166666666666852, 0.3281250000000000000, 0.3333333333333333148, 0.3359374999999999445 ),
 .UNSPECIFIED. ) 
 CURVE ( )  GEOMETRIC_REPRESENTATION_ITEM ( )  RATIONAL_B_SPLINE_CURVE ( ( 0.9330127018922194093, 0.9330127018922194093, 1.000000000000000000, 0.8660254037844387076, 1.000000000000000000, 0.8660254037844387076, 1.000000000000000000, 0.9330127018922207416, 0.9330127018922192983 ) ) 
 REPRESENTATION_ITEM ( '' )  );
#3730=CARTESIAN_POINT ( 'NONE',  ( -61.56765823437498852, 10.34895833299193413, 2.248837904296538515 ) ) ;
#3731=PLANE ( 'NONE',  #752 ) ;
#3736=DIRECTION ( 'NONE',  ( -0.000000000000000000, -1.000000000000000000, -0.000000000000000000 ) ) ;
#3737=CARTESIAN_POINT ( 'NONE',  ( -62.43234176562498305, 11.91145833299193413, 0.7511620957034662593 ) ) ;
#3738=CARTESIAN_POINT ( 'NONE',  ( -61.13531646874998415, 9.828124999658601979, 1.500000000000002220 ) ) ;
#3741=CARTESIAN_POINT ( 'NONE',  ( -61.49999999999998579, 8.510416665983868256, 0.6339745962155628467 ) ) ;
#3742=CARTESIAN_POINT ( 'NONE',  ( -62.86468353124999453, 10.53645833299193413, 1.999225269531025750 ) ) ;
#3744=CARTESIAN_POINT ( 'NONE',  ( -61.56765823437498142, 14.86979166632526805, 0.7511620957034663704 ) ) ;
#3745=CARTESIAN_POINT ( 'NONE',  ( -62.99999999999998579, 15.11458333265053433, 2.077350269189627952 ) ) ;
#3748=CARTESIAN_POINT ( 'NONE',  ( -61.99999999999998579, 16.00000000000000000, 0.5000000000000041078 ) ) ;
#3749=ORIENTED_EDGE ( 'NONE', *, *, #3428, .F. ) ;
#3750=CARTESIAN_POINT ( 'NONE',  ( -62.86468353124999453, 12.72395833299193413, 1.999225269531025750 ) ) ;
#3751=CARTESIAN_POINT ( 'NONE',  ( -61.13531646874998415, 8.598958332991934128, 1.000774730468978468 ) ) ;
#3753=ORIENTED_EDGE ( 'NONE', *, *, #6750, .T. ) ;
#3754=CARTESIAN_POINT ( 'NONE',  ( -60.99999999999998579, 12.00000000000000000, 1.500000000000002220 ) ) ;
#3756=CARTESIAN_POINT ( 'NONE',  ( -62.86468353124999453, 14.76562499965860020, 1.500000000000002220 ) ) ;
#3758=CARTESIAN_POINT ( 'NONE',  ( -61.99999999999998579, 16.00000000000000000, 1.500000000000002220 ) ) ;
#3759=CARTESIAN_POINT ( 'NONE',  ( -62.49999999999998579, 10.55208333265053611, 0.6339745962155627357 ) ) ;
#3761=VECTOR ( 'NONE', #4218, 1000.000000000000000 ) ;
#3763=CARTESIAN_POINT ( 'NONE',  ( -61.73205080756886076, 9.917414549001833279, 2.500000000000003109 ) ) ;
#3765=CARTESIAN_POINT ( 'NONE',  ( -62.86468353124999453, 12.45312499965860198, 1.500000000000002220 ) ) ;
#3769=CARTESIAN_POINT ( 'NONE',  ( -61.99999999999998579, 10.82812499965860198, 2.498450539062049724 ) ) ;
#3770=CARTESIAN_POINT ( 'NONE',  ( -62.49999999999998579, 15.63541666598386826, 2.366025403784441483 ) ) ;
#3771=CARTESIAN_POINT ( 'NONE',  ( -62.86468353124998742, 14.78645833299193413, 1.999225269531025972 ) ) ;
#3777=ORIENTED_EDGE ( 'NONE', *, *, #1352, .T. ) ;
#3778=DIRECTION ( 'NONE',  ( -0.000000000000000000, -1.000000000000000000, -0.000000000000000000 ) ) ;
#3779=CARTESIAN_POINT ( 'NONE',  ( -62.86468353124999453, 15.95312499965860198, 1.500000000000002220 ) ) ;
#3781=CARTESIAN_POINT ( 'NONE',  ( -61.99999999999998579, 11.93750000000000000, 2.500000000000002665 ) ) ;
#3782=DIRECTION ( 'NONE',  ( 0.000000000000000000, 1.000000000000000000, 0.000000000000000000 ) ) ;
#3784=EDGE_CURVE ( 'NONE', #5388, #5305, #3423, .T. ) ;
#3785=CARTESIAN_POINT ( 'NONE',  ( -62.86468353124998032, 14.74479166632526983, 1.000774730468978024 ) ) ;
#3786=CARTESIAN_POINT ( 'NONE',  ( -61.56765823437498852, 10.28645833299193413, 2.248837904296538515 ) ) ;
#3787=CARTESIAN_POINT ( 'NONE',  ( -62.99999999999998579, 11.34374999931720218, 1.500000000000001998 ) ) ;
#3789=CARTESIAN_POINT ( 'NONE',  ( -62.43234176562499016, 10.30729166632526983, 2.248837904296538071 ) ) ;
#3790=EDGE_CURVE ( 'NONE', #1925, #10979, #4561, .T. ) ;
#3791=CARTESIAN_POINT ( 'NONE',  ( -62.99999999999998579, 13.64583333333333215, 2.077350269189627952 ) ) ;
#3793=CARTESIAN_POINT ( 'NONE',  ( -61.99999999999998579, 14.43749999999999822, 2.500000000000002665 ) ) ;
#3797=CARTESIAN_POINT ( 'NONE',  ( -62.99999999999998579, 10.34374999931720218, 1.500000000000001998 ) ) ;
#3798=CARTESIAN_POINT ( 'NONE',  ( -61.56765823437498142, 11.86979166632526805, 0.7511620957034663704 ) ) ;
#3799=CARTESIAN_POINT ( 'NONE',  ( -62.86468353124999453, 10.72395833299193413, 1.999225269531025750 ) ) ;
#3800=CARTESIAN_POINT ( 'NONE',  ( -62.99999999999998579, 8.604166666666666075, 0.9226497308103756012 ) ) ;
#3801=( BOUNDED_CURVE ( )  B_SPLINE_CURVE ( 2, ( #8603, #210, #156, #4202, #982, #7772, #3483, #7607, #3540 ),
 .UNSPECIFIED., .F., .T. ) 
 B_SPLINE_CURVE_WITH_KNOTS ( ( 3, 2, 2, 2, 3 ),
 ( 0.1328125000000000000, 0.1354166666666666574, 0.1406250000000000000, 0.1458333333333333426, 0.1484374999999999722 ),
 .UNSPECIFIED. ) 
 CURVE ( )  GEOMETRIC_REPRESENTATION_ITEM ( )  RATIONAL_B_SPLINE_CURVE ( ( 0.9330127018922194093, 0.9330127018922194093, 1.000000000000000000, 0.8660254037844387076, 1.000000000000000000, 0.8660254037844387076, 1.000000000000000000, 0.9330127018922200755, 0.9330127018922194093 ) ) 
 REPRESENTATION_ITEM ( '' )  );
#3803=FACE_OUTER_BOUND ( 'NONE', #4271, .T. ) ;
#3804=CARTESIAN_POINT ( 'NONE',  ( -62.86468353124999453, 11.01562499965860020, 1.500000000000002220 ) ) ;
#3806=CARTESIAN_POINT ( 'NONE',  ( -62.86468353124998032, 14.68229166632526805, 1.000774730468978246 ) ) ;
#3807=CARTESIAN_POINT ( 'NONE',  ( -60.99999999999998579, 15.21874999931720218, 1.500000000000002220 ) ) ;
#3810=CARTESIAN_POINT ( 'NONE',  ( -61.99999999999998579, 16.00000000000000000, 0.5000000000000041078 ) ) ;
#3811=ORIENTED_EDGE ( 'NONE', *, *, #1647, .T. ) ;
#3812=EDGE_CURVE ( 'NONE', #4311, #10281, #5702, .T. ) ;
#3813=CARTESIAN_POINT ( 'NONE',  ( -61.13531646874997705, 13.30729166632526983, 1.999225269531026417 ) ) ;
#3814=CARTESIAN_POINT ( 'NONE',  ( -61.56765823437498852, 8.286458332991934128, 2.248837904296538515 ) ) ;
#3815=CARTESIAN_POINT ( 'NONE',  ( -61.99999999999998579, 11.68749999999999822, 2.500000000000002665 ) ) ;
#3816=ORIENTED_EDGE ( 'NONE', *, *, #10358, .F. ) ;
#3817=CARTESIAN_POINT ( 'NONE',  ( -62.49999999999998579, 11.83333333333333215, 0.6339745962155627357 ) ) ;
#3818=CARTESIAN_POINT ( 'NONE',  ( -60.99999999999998579, 15.96874999931720218, 1.500000000000002220 ) ) ;
#3820=CARTESIAN_POINT ( 'NONE',  ( -62.26794919243111082, 14.39508544963257286, 2.500000000000003109 ) ) ;
#3821=CARTESIAN_POINT ( 'NONE',  ( -62.49999999999998579, 11.13541666598387003, 2.366025403784441483 ) ) ;
#3825=CARTESIAN_POINT ( 'NONE',  ( -61.99999999999998579, 13.01562499965860198, 2.498450539062049724 ) ) ;
#3827=CARTESIAN_POINT ( 'NONE',  ( -61.13531646874998415, 9.911458332991935904, 1.000774730468978468 ) ) ;
#3828=CARTESIAN_POINT ( 'NONE',  ( -62.49999999999998579, 12.55208333265053611, 0.6339745962155627357 ) ) ;
#3829=ADVANCED_FACE ( 'NONE', ( #9325 ), #5093, .T. ) ;
#3830=CARTESIAN_POINT ( 'NONE',  ( -62.86468353124998032, 15.49479166632526628, 1.000774730468978246 ) ) ;
#3833=CARTESIAN_POINT ( 'NONE',  ( -61.49999999999998579, 10.45833333333333393, 2.366025403784441927 ) ) ;
#3834=ORIENTED_EDGE ( 'NONE', *, *, #8863, .F. ) ;
#3835=LINE ( 'NONE', #9550, #2353 ) ;
#3836=CARTESIAN_POINT ( 'NONE',  ( -61.99999999999998579, 10.18750000000000000, 2.654700538379254571 ) ) ;
#3837=CARTESIAN_POINT ( 'NONE',  ( -61.99999999999998579, 11.31250000000000000, 0.5000000000000013323 ) ) ;
#3840=CARTESIAN_POINT ( 'NONE',  ( -61.13531646874998415, 10.30729166632526805, 1.999225269531026417 ) ) ;
#3841=CARTESIAN_POINT ( 'NONE',  ( -62.26794919243111082, 11.29241454900183328, 0.4999999999999982792 ) ) ;
#3843=CARTESIAN_POINT ( 'NONE',  ( -61.56765823437498852, 10.84895833299193413, 2.248837904296538515 ) ) ;
#3844=CARTESIAN_POINT ( 'NONE',  ( -62.99999999999998579, 12.10416666666666607, 0.9226497308103756012 ) ) ;
#3845=EDGE_LOOP ( 'NONE', ( #4077, #858, #3142, #4779 ) ) ;
#3846=CARTESIAN_POINT ( 'NONE',  ( -61.99999999999998579, 13.90624999931720218, 2.500000000000002665 ) ) ;
#3850=CARTESIAN_POINT ( 'NONE',  ( -61.49999999999998579, 10.26041666598387003, 0.6339745962155628467 ) ) ;
#3851=CARTESIAN_POINT ( 'NONE',  ( -62.43234176562498305, 12.41145833299193413, 0.7511620957034662593 ) ) ;
#3852=EDGE_CURVE ( 'NONE', #1800, #6871, #4143, .T. ) ;
#3853=CARTESIAN_POINT ( 'NONE',  ( -61.13531646874998415, 9.578124999658600203, 1.500000000000002220 ) ) ;
#3854=CARTESIAN_POINT ( 'NONE',  ( -61.99999999999998579, 12.53124999931720396, 0.5000000000000013323 ) ) ;
#3856=CARTESIAN_POINT ( 'NONE',  ( -61.73205080756884655, 8.417414549001831503, 2.500000000000004885 ) ) ;
#3857=CARTESIAN_POINT ( 'NONE',  ( -61.99999999999999289, 11.07812499965860020, 2.498450539062049724 ) ) ;
#3859=CARTESIAN_POINT ( 'NONE',  ( -62.49999999999998579, 13.63541666598387003, 2.366025403784441483 ) ) ;
#3860=CARTESIAN_POINT ( 'NONE',  ( -60.99999999999998579, 14.98958333265053788, 0.9226497308103762673 ) ) ;
#3861=CARTESIAN_POINT ( 'NONE',  ( -61.73205080756886076, 14.66741454900183150, 2.500000000000003109 ) ) ;
#3862=ORIENTED_EDGE ( 'NONE', *, *, #8457, .F. ) ;
#3865=( BOUNDED_CURVE ( )  B_SPLINE_CURVE ( 2, ( #6483, #7201, #10635, #2203, #2253, #590, #2926, #10696, #1254 ),
 .UNSPECIFIED., .F., .T. ) 
 B_SPLINE_CURVE_WITH_KNOTS ( ( 3, 2, 2, 2, 3 ),
 ( 0.8671875000000000000, 0.8697916666666666297, 0.8750000000000000000, 0.8802083333333333703, 0.8828125000000000000 ),
 .UNSPECIFIED. ) 
 CURVE ( )  GEOMETRIC_REPRESENTATION_ITEM ( )  RATIONAL_B_SPLINE_CURVE ( ( 0.9330127018922194093, 0.9330127018922194093, 1.000000000000000000, 0.8660254037844387076, 1.000000000000000000, 0.8660254037844387076, 1.000000000000000000, 0.9330127018922194093, 0.9330127018922194093 ) ) 
 REPRESENTATION_ITEM ( '' )  );
#3866=CARTESIAN_POINT ( 'NONE',  ( -62.86468353124998032, 13.43229166632526983, 1.000774730468978024 ) ) ;
#3867=CARTESIAN_POINT ( 'NONE',  ( -61.56765823437498852, 8.786458332991934128, 2.248837904296538515 ) ) ;
#3869=CARTESIAN_POINT ( 'NONE',  ( -60.99999999999998579, 11.72916666666666785, 2.077350269189628840 ) ) ;
#3870=ORIENTED_EDGE ( 'NONE', *, *, #5076, .T. ) ;
#3871=CARTESIAN_POINT ( 'NONE',  ( -61.99999999999998579, 11.81250000000000000, 0.3452994616207497591 ) ) ;
#3872=CARTESIAN_POINT ( 'NONE',  ( -62.99999999999998579, 8.593749999317203958, 1.500000000000001998 ) ) ;
#3875=CARTESIAN_POINT ( 'NONE',  ( -61.99999999999998579, 10.90624999931720218, 2.654700538379254571 ) ) ;
#3879=CARTESIAN_POINT ( 'NONE',  ( -62.86468353124998742, 12.47395833299193413, 1.999225269531025972 ) ) ;
#3883=CARTESIAN_POINT ( 'NONE',  ( -62.86468353124999453, 11.01562499965860020, 1.500000000000002220 ) ) ;
#3884=DIRECTION ( 'NONE',  ( -0.000000000000000000, -1.000000000000000000, -0.000000000000000000 ) ) ;
#3886=CARTESIAN_POINT ( 'NONE',  ( -61.99999999999998579, 16.07812499965860198, 2.498450539062049724 ) ) ;
#3891=VERTEX_POINT ( 'NONE', #1670 ) ;
#3892=CARTESIAN_POINT ( 'NONE',  ( -61.99999999999998579, 16.00000000000000000, 0.5000000000000041078 ) ) ;
#3893=CARTESIAN_POINT ( 'NONE',  ( -60.99999999999998579, 9.500000000000000000, 1.500000000000002220 ) ) ;
#3896=( BOUNDED_CURVE ( )  B_SPLINE_CURVE ( 2, ( #110, #4439, #59, #3442, #5264, #1679, #7787, #3331, #8670 ),
 .UNSPECIFIED., .F., .F. ) 
 B_SPLINE_CURVE_WITH_KNOTS ( ( 3, 2, 2, 2, 3 ),
 ( 0.1484374999999999722, 0.1510416666666666574, 0.1562500000000000000, 0.1614583333333333426, 0.1640624999999999722 ),
 .UNSPECIFIED. ) 
 CURVE ( )  GEOMETRIC_REPRESENTATION_ITEM ( )  RATIONAL_B_SPLINE_CURVE ( ( 0.9330127018922194093, 0.9330127018922186322, 1.000000000000000000, 0.8660254037844387076, 1.000000000000000000, 0.8660254037844387076, 1.000000000000000000, 0.9330127018922200755, 0.9330127018922194093 ) ) 
 REPRESENTATION_ITEM ( '' )  );
#3897=CARTESIAN_POINT ( 'NONE',  ( -61.99999999999998579, 14.78124999931720218, 0.5000000000000013323 ) ) ;
#3899=CARTESIAN_POINT ( 'NONE',  ( -60.99999999999998579, 8.447916665983870033, 2.077350269189628840 ) ) ;
#3900=CARTESIAN_POINT ( 'NONE',  ( -61.99999999999998579, 12.45312499965860020, 0.5015494609379544944 ) ) ;
#3902=ORIENTED_EDGE ( 'NONE', *, *, #9235, .T. ) ;
#3905=EDGE_CURVE ( 'NONE', #10857, #1159, #10170, .T. ) ;
#3907=ORIENTED_EDGE ( 'NONE', *, *, #4221, .T. ) ;
#3909=CARTESIAN_POINT ( 'NONE',  ( -62.43234176562498305, 13.91145833299193413, 0.7511620957034662593 ) ) ;
#3910=CARTESIAN_POINT ( 'NONE',  ( -61.56765823437498142, 10.86979166632526805, 0.7511620957034663704 ) ) ;
#3912=CARTESIAN_POINT ( 'NONE',  ( -62.99999999999998579, 14.14583333333333393, 2.077350269189627952 ) ) ;
#3913=CARTESIAN_POINT ( 'NONE',  ( -62.43234176562499016, 11.30729166632526805, 2.248837904296538071 ) ) ;
#3916=CARTESIAN_POINT ( 'NONE',  ( -62.99999999999998579, 15.59374999931720218, 1.500000000000001998 ) ) ;
#3917=CARTESIAN_POINT ( 'NONE',  ( -62.99999999999998579, 16.09374999931720396, 1.500000000000001998 ) ) ;
#3918=ORIENTED_EDGE ( 'NONE', *, *, #8577, .T. ) ;
#3919=DIRECTION ( 'NONE',  ( 0.000000000000000000, 1.000000000000000000, 0.000000000000000000 ) ) ;
#3920=ORIENTED_EDGE ( 'NONE', *, *, #6520, .F. ) ;
#3921=CARTESIAN_POINT ( 'NONE',  ( -62.43234176562499016, 12.49479166632526805, 2.248837904296538071 ) ) ;
#3922=CARTESIAN_POINT ( 'NONE',  ( -61.13531646874998415, 10.05729166632526983, 1.999225269531026417 ) ) ;
#3923=CARTESIAN_POINT ( 'NONE',  ( -60.99999999999998579, 11.75000000000000000, 1.500000000000002220 ) ) ;
#3925=CARTESIAN_POINT ( 'NONE',  ( -62.49999999999998579, 12.16666666666666607, 2.366025403784441483 ) ) ;
#3926=CARTESIAN_POINT ( 'NONE',  ( -61.99999999999998579, 11.03124999931720218, 0.5000000000000013323 ) ) ;
#3927=EDGE_CURVE ( 'NONE', #6224, #5880, #255, .T. ) ;
#3928=CARTESIAN_POINT ( 'NONE',  ( -61.49999999999998579, 12.26041666598386826, 0.6339745962155628467 ) ) ;
#3929=EDGE_CURVE ( 'NONE', #10050, #4452, #4019, .T. ) ;
#3931=CARTESIAN_POINT ( 'NONE',  ( -61.13531646874998415, 13.05729166632526628, 1.999225269531026417 ) ) ;
#3934=CARTESIAN_POINT ( 'NONE',  ( -61.13531646874998415, 11.86979166632526805, 1.999225269531026417 ) ) ;
#3935=CARTESIAN_POINT ( 'NONE',  ( -61.73205080756886076, 12.16741454900183506, 2.500000000000003109 ) ) ;
#3942=CARTESIAN_POINT ( 'NONE',  ( -60.99999999999998579, 8.739583332650536107, 0.9226497308103762673 ) ) ;
#3943=CARTESIAN_POINT ( 'NONE',  ( -61.49999999999998579, 10.20833333333333393, 2.366025403784441927 ) ) ;
#3944=CARTESIAN_POINT ( 'NONE',  ( -62.26794919243111082, 9.542414549001833279, 0.4999999999999998890 ) ) ;
#3945=CARTESIAN_POINT ( 'NONE',  ( -61.99999999999998579, 15.78124999931720218, 0.5000000000000013323 ) ) ;
#3947=CARTESIAN_POINT ( 'NONE',  ( -61.49999999999998579, 8.427083332650536107, 2.366025403784441927 ) ) ;
#3950=CARTESIAN_POINT ( 'NONE',  ( -61.56765823437498142, 11.93229166632526805, 0.7511620957034663704 ) ) ;
#3951=CARTESIAN_POINT ( 'NONE',  ( -61.13531646874998415, 8.078124999658601979, 1.500000000000002220 ) ) ;
#3952=VERTEX_POINT ( 'NONE', #5492 ) ;
#3953=ADVANCED_FACE ( 'NONE', ( #1105, #4489 ), #7053, .F. ) ;
#3956=( BOUNDED_CURVE ( )  B_SPLINE_CURVE ( 2, ( #5469, #3287, #4644, #1266, #8047, #436, #5840, #3820, #8105 ),
 .UNSPECIFIED., .F., .F. ) 
 B_SPLINE_CURVE_WITH_KNOTS ( ( 3, 2, 2, 2, 3 ),
 ( 0.7578125000000000000, 0.7604166666666666297, 0.7656250000000000000, 0.7708333333333333703, 0.7734375000000000000 ),
 .UNSPECIFIED. ) 
 CURVE ( )  GEOMETRIC_REPRESENTATION_ITEM ( )  RATIONAL_B_SPLINE_CURVE ( ( 0.9330127018922194093, 0.9330127018922194093, 1.000000000000000000, 0.8660254037844387076, 1.000000000000000000, 0.8660254037844387076, 1.000000000000000000, 0.9330127018922194093, 0.9330127018922194093 ) ) 
 REPRESENTATION_ITEM ( '' )  );
#3958=VERTEX_POINT ( 'NONE', #2950 ) ;
#3960=CARTESIAN_POINT ( 'NONE',  ( -61.13531646874998415, 14.07812499965860198, 1.500000000000002220 ) ) ;
#3962=CARTESIAN_POINT ( 'NONE',  ( -61.13531646874997705, 9.848958332991934128, 1.000774730468978468 ) ) ;
#3963=CARTESIAN_POINT ( 'NONE',  ( -61.99999999999998579, 8.187500000000001776, 2.500000000000003109 ) ) ;
#3966=CARTESIAN_POINT ( 'NONE',  ( -61.13531646874997705, 11.41145833299193590, 1.000774730468978468 ) ) ;
#3967=CARTESIAN_POINT ( 'NONE',  ( -61.99999999999998579, 14.82812499965860020, 2.498450539062049724 ) ) ;
#3970=EDGE_CURVE ( 'NONE', #10876, #4311, #1943, .T. ) ;
#3971=CARTESIAN_POINT ( 'NONE',  ( -61.49999999999998579, 15.76041666598386826, 0.6339745962155628467 ) ) ;
#3974=AXIS2_PLACEMENT_3D ( 'NONE', #6425, #2923, #10694 ) ;
#3976=DIRECTION ( 'NONE',  ( 0.000000000000000000, 0.000000000000000000, 1.000000000000000000 ) ) ;
#3977=CARTESIAN_POINT ( 'NONE',  ( -62.43234176562498305, 14.41145833299193413, 0.7511620957034662593 ) ) ;
#3978=CARTESIAN_POINT ( 'NONE',  ( -61.56765823437498142, 10.36979166632526983, 0.7511620957034663704 ) ) ;
#3981=CARTESIAN_POINT ( 'NONE',  ( -62.49999999999998579, 14.08333333333333393, 0.6339745962155627357 ) ) ;
#3984=CARTESIAN_POINT ( 'NONE',  ( -60.99999999999998579, 11.98958333265053433, 0.9226497308103762673 ) ) ;
#3986=CARTESIAN_POINT ( 'NONE',  ( -62.86468353124999453, 13.45312499965860020, 1.500000000000002220 ) ) ;
#3987=ORIENTED_EDGE ( 'NONE', *, *, #283, .T. ) ;
#3988=EDGE_CURVE ( 'NONE', #562, #7309, #8556, .T. ) ;
#3989=CARTESIAN_POINT ( 'NONE',  ( -62.43234176562498305, 11.72395833299193590, 0.7511620957034662593 ) ) ;
#3990=CARTESIAN_POINT ( 'NONE',  ( -61.99999999999998579, 16.00000000000000000, 0.5000000000000041078 ) ) ;
#3991=CARTESIAN_POINT ( 'NONE',  ( -61.99999999999998579, 15.82812499965860020, 2.498450539062049724 ) ) ;
#3993=CARTESIAN_POINT ( 'NONE',  ( -61.99999999999998579, 11.06250000000000000, 0.5000000000000013323 ) ) ;
#3995=CARTESIAN_POINT ( 'NONE',  ( -62.99999999999998579, 9.864583332650536107, 2.077350269189627952 ) ) ;
#3996=CARTESIAN_POINT ( 'NONE',  ( -60.99999999999998579, 9.770833333333332149, 0.9226497308103762673 ) ) ;
#3999=CARTESIAN_POINT ( 'NONE',  ( -61.99999999999998579, 15.81250000000000000, 0.5000000000000013323 ) ) ;
#4000=CARTESIAN_POINT ( 'NONE',  ( -60.99999999999998579, 8.468749999317202182, 1.500000000000002220 ) ) ;
#4001=EDGE_CURVE ( 'NONE', #5880, #4509, #3835, .T. ) ;
#4002=CARTESIAN_POINT ( 'NONE',  ( -61.13531646874998415, 12.16145833299193413, 1.000774730468978468 ) ) ;
#4005=CARTESIAN_POINT ( 'NONE',  ( -61.99999999999998579, 12.78124999931720218, 0.5000000000000013323 ) ) ;
#4008=CARTESIAN_POINT ( 'NONE',  ( -61.56765823437498852, 14.03645833299193413, 2.248837904296538515 ) ) ;
#4009=DIRECTION ( 'NONE',  ( -0.000000000000000000, -1.000000000000000000, -0.000000000000000000 ) ) ;
#4011=CARTESIAN_POINT ( 'NONE',  ( -61.56765823437498142, 10.93229166632526805, 0.7511620957034663704 ) ) ;
#4012=CARTESIAN_POINT ( 'NONE',  ( -61.99999999999998579, 15.32812499965860198, 2.498450539062049724 ) ) ;
#4013=CARTESIAN_POINT ( 'NONE',  ( -62.99999999999998579, 13.61458333265053611, 2.077350269189627952 ) ) ;
#4014=CARTESIAN_POINT ( 'NONE',  ( -62.99999999999998579, 15.61458333265053611, 2.077350269189627952 ) ) ;
#4016=ORIENTED_EDGE ( 'NONE', *, *, #5528, .F. ) ;
#4019=( BOUNDED_CURVE ( )  B_SPLINE_CURVE ( 2, ( #217, #8836, #3657, #4542, #7948, #2001, #1283, #4660, #8725 ),
 .UNSPECIFIED., .F., .T. ) 
 B_SPLINE_CURVE_WITH_KNOTS ( ( 3, 2, 2, 2, 3 ),
 ( 0.8515625000000000000, 0.8541666666666666297, 0.8593750000000000000, 0.8645833333333333703, 0.8671875000000000000 ),
 .UNSPECIFIED. ) 
 CURVE ( )  GEOMETRIC_REPRESENTATION_ITEM ( )  RATIONAL_B_SPLINE_CURVE ( ( 0.9330127018922194093, 0.9330127018922194093, 1.000000000000000000, 0.8660254037844387076, 1.000000000000000000, 0.8660254037844387076, 1.000000000000000000, 0.9330127018922194093, 0.9330127018922194093 ) ) 
 REPRESENTATION_ITEM ( '' )  );
#4020=CARTESIAN_POINT ( 'NONE',  ( -61.56765823437498142, 13.86979166632526805, 0.7511620957034663704 ) ) ;
#4022=CARTESIAN_POINT ( 'NONE',  ( -62.86468353124999453, 10.45312499965860198, 1.500000000000002220 ) ) ;
#4024=ORIENTED_EDGE ( 'NONE', *, *, #9521, .T. ) ;
#4025=CARTESIAN_POINT ( 'NONE',  ( -61.99999999999998579, 13.93750000000000000, 2.654700538379254571 ) ) ;
#4027=CARTESIAN_POINT ( 'NONE',  ( -61.49999999999998579, 11.67708333265053611, 2.366025403784441927 ) ) ;
#4028=CARTESIAN_POINT ( 'NONE',  ( -61.56765823437498142, 13.86979166632526805, 0.7511620957034663704 ) ) ;
#4030=VERTEX_POINT ( 'NONE', #9160 ) ;
#4031=CARTESIAN_POINT ( 'NONE',  ( -61.99999999999998579, 11.57812499965860198, 2.498450539062049724 ) ) ;
#4034=PRODUCT_DEFINITION_SHAPE ( 'NONE', 'NONE',  #5343 ) ;
#4039=AXIS2_PLACEMENT_3D ( 'NONE', #6137, #1862, #6757 ) ;
#4041=CARTESIAN_POINT ( 'NONE',  ( -62.49999999999998579, 9.802083332650536107, 0.6339745962155627357 ) ) ;
#4042=CARTESIAN_POINT ( 'NONE',  ( -62.99999999999998579, 9.375000000000000000, 1.500000000000001998 ) ) ;
#4043=VECTOR ( 'NONE', #820, 1000.000000000000000 ) ;
#4044=CARTESIAN_POINT ( 'NONE',  ( -62.43234176562498305, 8.223958332991934128, 0.7511620957034662593 ) ) ;
#4045=CARTESIAN_POINT ( 'NONE',  ( -60.99999999999998579, 15.48958333265053433, 0.9226497308103762673 ) ) ;
#4046=EDGE_CURVE ( 'NONE', #4413, #1330, #8953, .T. ) ;
#4048=CARTESIAN_POINT ( 'NONE',  ( -61.56765823437498852, 11.34895833299193590, 2.248837904296538515 ) ) ;
#4049=CARTESIAN_POINT ( 'NONE',  ( -61.99999999999998579, 14.65624999931719863, 2.500000000000002665 ) ) ;
#4051=CARTESIAN_POINT ( 'NONE',  ( -62.99999999999998579, 15.35416666666666785, 0.9226497308103756012 ) ) ;
#4052=EDGE_CURVE ( 'NONE', #5466, #5034, #674, .T. ) ;
#4053=AXIS2_PLACEMENT_3D ( 'NONE', #6840, #2611, #10109 ) ;
#4057=CARTESIAN_POINT ( 'NONE',  ( -61.56765823437498142, 13.36979166632526805, 0.7511620957034663704 ) ) ;
#4060=CARTESIAN_POINT ( 'NONE',  ( -62.49999999999998579, 14.16666666666666785, 2.366025403784441483 ) ) ;
#4061=CARTESIAN_POINT ( 'NONE',  ( -61.13531646874997705, 12.36979166632526805, 1.999225269531026417 ) ) ;
#4062=CARTESIAN_POINT ( 'NONE',  ( -62.86468353124998032, 15.74479166632526805, 1.000774730468978246 ) ) ;
#4064=DIRECTION ( 'NONE',  ( 0.000000000000000000, 0.000000000000000000, -1.000000000000000000 ) ) ;
#4065=CARTESIAN_POINT ( 'NONE',  ( -62.99999999999998579, 15.10416666666666607, 0.9226497308103756012 ) ) ;
#4066=CARTESIAN_POINT ( 'NONE',  ( -62.86468353124999453, 8.265624999658601979, 1.500000000000002220 ) ) ;
#4068=ORIENTED_EDGE ( 'NONE', *, *, #8863, .T. ) ;
#4073=CARTESIAN_POINT ( 'NONE',  ( -61.99999999999999289, 13.76562499965860198, 2.498450539062049724 ) ) ;
#4074=CARTESIAN_POINT ( 'NONE',  ( -61.99999999999998579, 9.890624999658601979, 0.5015494609379544944 ) ) ;
#4075=CARTESIAN_POINT ( 'NONE',  ( -61.13531646874998415, 8.078124999658601979, 1.500000000000002220 ) ) ;
#4077=ORIENTED_EDGE ( 'NONE', *, *, #3927, .F. ) ;
#4078=CARTESIAN_POINT ( 'NONE',  ( -62.99999999999998579, 13.35416666666666785, 0.9226497308103756012 ) ) ;
#4079=CARTESIAN_POINT ( 'NONE',  ( -62.86468353124999453, 9.265624999658600203, 1.500000000000002220 ) ) ;
#4082=CARTESIAN_POINT ( 'NONE',  ( -61.49999999999998579, 12.51041666598386826, 0.6339745962155628467 ) ) ;
#4084=( BOUNDED_CURVE ( )  B_SPLINE_CURVE ( 2, ( #6616, #4097, #9994, #6457, #1544, #4926, #8324, #3109, #9839 ),
 .UNSPECIFIED., .F., .T. ) 
 B_SPLINE_CURVE_WITH_KNOTS ( ( 3, 2, 2, 2, 3 ),
 ( 0.1484374999999999722, 0.1510416666666666574, 0.1562500000000000000, 0.1614583333333333426, 0.1640624999999999722 ),
 .UNSPECIFIED. ) 
 CURVE ( )  GEOMETRIC_REPRESENTATION_ITEM ( )  RATIONAL_B_SPLINE_CURVE ( ( 0.9330127018922194093, 0.9330127018922186322, 1.000000000000000000, 0.8660254037844387076, 1.000000000000000000, 0.8660254037844387076, 1.000000000000000000, 0.9330127018922200755, 0.9330127018922194093 ) ) 
 REPRESENTATION_ITEM ( '' )  );
#4086=CARTESIAN_POINT ( 'NONE',  ( -61.13531646874998415, 13.57812499965860198, 1.500000000000002220 ) ) ;
#4089=CARTESIAN_POINT ( 'NONE',  ( -62.86468353124998032, 11.24479166632526805, 1.000774730468978246 ) ) ;
#4090=LINE ( 'NONE', #6761, #8317 ) ;
#4091=EDGE_CURVE ( 'NONE', #6875, #4509, #7782, .T. ) ;
#4093=DIRECTION ( 'NONE',  ( 0.000000000000000000, 0.000000000000000000, -1.000000000000000000 ) ) ;
#4097=CARTESIAN_POINT ( 'NONE',  ( -61.73205080756886787, 9.417414549001833279, 2.500000000000004885 ) ) ;
#4098=CARTESIAN_POINT ( 'NONE',  ( -60.99999999999998579, 11.50000000000000000, 1.500000000000002220 ) ) ;
#4099=CARTESIAN_POINT ( 'NONE',  ( -61.99999999999998579, 9.781249999317202182, 0.5000000000000013323 ) ) ;
#4101=CARTESIAN_POINT ( 'NONE',  ( -61.99999999999998579, 9.406249999317202182, 2.654700538379254571 ) ) ;
#4102=CARTESIAN_POINT ( 'NONE',  ( -62.86468353124999453, 12.76562499965860198, 1.500000000000002220 ) ) ;
#4103=CARTESIAN_POINT ( 'NONE',  ( -62.49999999999998579, 10.58333333333333393, 0.6339745962155627357 ) ) ;
#4104=ORIENTED_EDGE ( 'NONE', *, *, #1718, .T. ) ;
#4106=CARTESIAN_POINT ( 'NONE',  ( -62.26794919243111082, 15.42633545031536713, 2.500000000000003109 ) ) ;
#4107=ORIENTED_EDGE ( 'NONE', *, *, #901, .F. ) ;
#4109=EDGE_CURVE ( 'NONE', #5909, #2359, #4084, .T. ) ;
#4110=CARTESIAN_POINT ( 'NONE',  ( -62.86468353124998032, 14.68229166632526805, 1.000774730468978246 ) ) ;
#4111=CARTESIAN_POINT ( 'NONE',  ( -60.99999999999998579, 13.72916666666666785, 2.077350269189628840 ) ) ;
#4112=CARTESIAN_POINT ( 'NONE',  ( -60.99999999999998579, 14.49999999999999822, 1.500000000000002220 ) ) ;
#4115=CARTESIAN_POINT ( 'NONE',  ( -61.13531646874997705, 13.36979166632526805, 1.999225269531026417 ) ) ;
#4116=CARTESIAN_POINT ( 'NONE',  ( -62.43234176562499016, 15.30729166632526805, 2.248837904296538071 ) ) ;
#4121=CARTESIAN_POINT ( 'NONE',  ( -61.99999999999998579, 16.15624999931720396, 2.654700538379254571 ) ) ;
#4123=ORIENTED_EDGE ( 'NONE', *, *, #6104, .T. ) ;
#4128=CARTESIAN_POINT ( 'NONE',  ( -61.56765823437498852, 14.53645833299193413, 2.248837904296538515 ) ) ;
#4129=CARTESIAN_POINT ( 'NONE',  ( -61.13531646874998415, 9.828124999658601979, 1.500000000000002220 ) ) ;
#4130=CARTESIAN_POINT ( 'NONE',  ( -61.99999999999999289, 15.20312499965860020, 0.5015494609379544944 ) ) ;
#4131=CARTESIAN_POINT ( 'NONE',  ( -61.99999999999998579, 26.00000000000000355, 1.500000000000002220 ) ) ;
#4133=CARTESIAN_POINT ( 'NONE',  ( -60.99999999999998579, 13.75000000000000000, 1.500000000000002220 ) ) ;
#4134=CARTESIAN_POINT ( 'NONE',  ( -62.43234176562498305, 8.723958332991934128, 0.7511620957034662593 ) ) ;
#4135=SURFACE_STYLE_USAGE ( .BOTH. , #5801 ) ;
#4136=CARTESIAN_POINT ( 'NONE',  ( -60.99999999999998579, 12.23958333265053611, 0.9226497308103762673 ) ) ;
#4137=ADVANCED_FACE ( 'NONE', ( #2226 ), #5605, .T. ) ;
#4139=CARTESIAN_POINT ( 'NONE',  ( -61.13531646874998415, 14.05729166632526805, 1.999225269531026417 ) ) ;
#4142=CARTESIAN_POINT ( 'NONE',  ( -61.13531646874998415, 12.86979166632526628, 1.999225269531026417 ) ) ;
#4143=( BOUNDED_CURVE ( )  B_SPLINE_CURVE ( 2, ( #6833, #8496, #10935, #3326, #828, #3487, #9491, #1775, #6727 ),
 .UNSPECIFIED., .F., .T. ) 
 B_SPLINE_CURVE_WITH_KNOTS ( ( 3, 2, 2, 2, 3 ),
 ( 0.5859375000000000000, 0.5885416666666666297, 0.5937500000000000000, 0.5989583333333333703, 0.6015625000000000000 ),
 .UNSPECIFIED. ) 
 CURVE ( )  GEOMETRIC_REPRESENTATION_ITEM ( )  RATIONAL_B_SPLINE_CURVE ( ( 0.9330127018922194093, 0.9330127018922194093, 1.000000000000000000, 0.8660254037844387076, 1.000000000000000000, 0.8660254037844387076, 1.000000000000000000, 0.9330127018922194093, 0.9330127018922194093 ) ) 
 REPRESENTATION_ITEM ( '' )  );
#4144=DIRECTION ( 'NONE',  ( -0.000000000000000000, -1.000000000000000000, -0.000000000000000000 ) ) ;
#4146=DIRECTION ( 'NONE',  ( -0.000000000000000000, -1.000000000000000000, -0.000000000000000000 ) ) ;
#4148=CARTESIAN_POINT ( 'NONE',  ( -61.99999999999998579, 11.56250000000000000, 0.3452994616207497591 ) ) ;
#4150=CARTESIAN_POINT ( 'NONE',  ( -62.86468353124998032, 9.494791666325269830, 1.000774730468978246 ) ) ;
#4151=CARTESIAN_POINT ( 'NONE',  ( -61.99999999999998579, 16.00000000000000000, 2.500000000000000444 ) ) ;
#4152=CARTESIAN_POINT ( 'NONE',  ( -61.99999999999998579, 12.70312499965860198, 0.5015494609379544944 ) ) ;
#4153=CARTESIAN_POINT ( 'NONE',  ( -62.49999999999998579, 9.135416665983868256, 2.366025403784441483 ) ) ;
#4158=CARTESIAN_POINT ( 'NONE',  ( -62.86468353124999453, 14.70312499965860020, 1.500000000000002220 ) ) ;
#4159=CARTESIAN_POINT ( 'NONE',  ( -61.99999999999998579, 9.531249999317202182, 0.5000000000000013323 ) ) ;
#4161=CARTESIAN_POINT ( 'NONE',  ( -62.99999999999998579, 12.32291666598386826, 0.9226497308103756012 ) ) ;
#4162=CARTESIAN_POINT ( 'NONE',  ( -61.56765823437498852, 12.59895833299193413, 2.248837904296538515 ) ) ;
#4163=CARTESIAN_POINT ( 'NONE',  ( -61.13531646874998415, 15.66145833299193590, 1.000774730468978468 ) ) ;
#4164=CARTESIAN_POINT ( 'NONE',  ( -61.49999999999998579, 15.04166666666666607, 0.6339745962155628467 ) ) ;
#4166=CARTESIAN_POINT ( 'NONE',  ( -62.86468353124999453, 9.015624999658601979, 1.500000000000002220 ) ) ;
#4168=ORIENTED_EDGE ( 'NONE', *, *, #4109, .T. ) ;
#4171=EDGE_CURVE ( 'NONE', #3478, #8518, #3590, .T. ) ;
#4172=CARTESIAN_POINT ( 'NONE',  ( -61.13531646874997705, 14.59895833299193413, 1.000774730468978468 ) ) ;
#4173=CARTESIAN_POINT ( 'NONE',  ( -62.86468353124998742, 10.97395833299193768, 1.999225269531025972 ) ) ;
#4174=CARTESIAN_POINT ( 'NONE',  ( -61.13531646874997705, 15.11979166632526983, 1.999225269531026417 ) ) ;
#4175=CARTESIAN_POINT ( 'NONE',  ( -60.99999999999998579, 14.46874999931720218, 1.500000000000002220 ) ) ;
#4176=ORIENTED_EDGE ( 'NONE', *, *, #722, .F. ) ;
#4177=CARTESIAN_POINT ( 'NONE',  ( -61.49999999999998579, 14.04166666666666785, 0.6339745962155628467 ) ) ;
#4178=CARTESIAN_POINT ( 'NONE',  ( -61.99999999999999289, 8.578124999658601979, 2.498450539062049724 ) ) ;
#4179=CARTESIAN_POINT ( 'NONE',  ( -60.99999999999998579, 12.98958333265053433, 0.9226497308103762673 ) ) ;
#4182=CARTESIAN_POINT ( 'NONE',  ( -61.13531646874998415, 13.80729166632526983, 1.999225269531026417 ) ) ;
#4183=CARTESIAN_POINT ( 'NONE',  ( -62.99999999999998579, 15.62500000000000000, 1.500000000000001998 ) ) ;
#4185=EDGE_CURVE ( 'NONE', #1245, #8943, #959, .T. ) ;
#4187=CARTESIAN_POINT ( 'NONE',  ( -62.43234176562499016, 12.30729166632526805, 2.248837904296538071 ) ) ;
#4189=ORIENTED_EDGE ( 'NONE', *, *, #4091, .F. ) ;
#4194=( BOUNDED_CURVE ( )  B_SPLINE_CURVE ( 2, ( #6006, #66, #7907, #1958, #9565, #8622, #4381, #9394, #7794 ),
 .UNSPECIFIED., .F., .T. ) 
 B_SPLINE_CURVE_WITH_KNOTS ( ( 3, 2, 2, 2, 3 ),
 ( 0.3671875000000000000, 0.3697916666666666852, 0.3750000000000000000, 0.3802083333333333148, 0.3828124999999999445 ),
 .UNSPECIFIED. ) 
 CURVE ( )  GEOMETRIC_REPRESENTATION_ITEM ( )  RATIONAL_B_SPLINE_CURVE ( ( 0.9330127018922194093, 0.9330127018922194093, 1.000000000000000000, 0.8660254037844387076, 1.000000000000000000, 0.8660254037844387076, 1.000000000000000000, 0.9330127018922207416, 0.9330127018922192983 ) ) 
 REPRESENTATION_ITEM ( '' )  );
#4195=ORIENTED_EDGE ( 'NONE', *, *, #3546, .T. ) ;
#4196=CARTESIAN_POINT ( 'NONE',  ( -62.49999999999998579, 11.66666666666666785, 2.366025403784441483 ) ) ;
#4199=CARTESIAN_POINT ( 'NONE',  ( -62.43234176562499016, 8.307291666325268054, 2.248837904296538071 ) ) ;
#4200=CARTESIAN_POINT ( 'NONE',  ( -61.73205080756886076, 10.52008544963257464, 0.5000000000000044409 ) ) ;
#4201=CARTESIAN_POINT ( 'NONE',  ( -62.43234176562499016, 13.05729166632526805, 2.248837904296538071 ) ) ;
#4202=CARTESIAN_POINT ( 'NONE',  ( -62.99999999999998579, 9.322916665983871809, 0.9226497308103756012 ) ) ;
#4204=CARTESIAN_POINT ( 'NONE',  ( -60.99999999999998579, 10.96874999931720218, 1.500000000000002220 ) ) ;
#4207=ORIENTED_EDGE ( 'NONE', *, *, #8822, .T. ) ;
#4208=CARTESIAN_POINT ( 'NONE',  ( -62.43234176562499016, 14.74479166632526805, 2.248837904296538071 ) ) ;
#4210=CARTESIAN_POINT ( 'NONE',  ( -61.73205080756886076, 12.44866454968463110, 2.500000000000003109 ) ) ;
#4213=CARTESIAN_POINT ( 'NONE',  ( -61.13531646874997705, 13.11979166632526805, 1.999225269531026417 ) ) ;
#4214=CARTESIAN_POINT ( 'NONE',  ( -61.13531646874998415, 15.64062499965860198, 1.500000000000002220 ) ) ;
#4217=CARTESIAN_POINT ( 'NONE',  ( -62.43234176562498305, 9.723958332991934128, 0.7511620957034662593 ) ) ;
#4218=DIRECTION ( 'NONE',  ( -0.000000000000000000, -1.000000000000000000, -0.000000000000000000 ) ) ;
#4219=ORIENTED_EDGE ( 'NONE', *, *, #3016, .F. ) ;
#4220=CARTESIAN_POINT ( 'NONE',  ( -61.99999999999998579, 16.00000000000000000, 0.5000000000000041078 ) ) ;
#4221=EDGE_CURVE ( 'NONE', #3055, #10734, #2243, .T. ) ;
#4224=CARTESIAN_POINT ( 'NONE',  ( -62.86468353124998032, 15.43229166632526805, 1.000774730468978024 ) ) ;
#4225=CARTESIAN_POINT ( 'NONE',  ( -61.13531646874998415, 11.82812499965860198, 1.500000000000002220 ) ) ;
#4226=CARTESIAN_POINT ( 'NONE',  ( -62.86468353124998032, 14.99479166632526628, 1.000774730468978024 ) ) ;
#4227=CARTESIAN_POINT ( 'NONE',  ( -62.49999999999998579, 13.05208333265053611, 0.6339745962155627357 ) ) ;
#4229=CARTESIAN_POINT ( 'NONE',  ( -62.49999999999998579, 15.33333333333333393, 0.6339745962155627357 ) ) ;
#4230=CARTESIAN_POINT ( 'NONE',  ( -61.56765823437498142, 8.182291666325268054, 0.7511620957034663704 ) ) ;
#4231=VECTOR ( 'NONE', #1523, 1000.000000000000000 ) ;
#4232=CARTESIAN_POINT ( 'NONE',  ( -62.49999999999998579, 13.88541666598387003, 2.366025403784441483 ) ) ;
#4235=CARTESIAN_POINT ( 'NONE',  ( -61.99999999999999289, 11.01562499965859843, 2.498450539062049724 ) ) ;
#4238=VERTEX_POINT ( 'NONE', #8587 ) ;
#4240=CARTESIAN_POINT ( 'NONE',  ( -62.49999999999998579, 12.91666666666666607, 2.366025403784441483 ) ) ;
#4242=CARTESIAN_POINT ( 'NONE',  ( -62.43234176562498305, 13.47395833299193413, 0.7511620957034662593 ) ) ;
#4243=DIRECTION ( 'NONE',  ( -1.000000000000000000, 0.000000000000000000, -0.000000000000000000 ) ) ;
#4244=EDGE_CURVE ( 'NONE', #8518, #2471, #759, .T. ) ;
#4245=EDGE_LOOP ( 'NONE', ( #7348, #2049, #442, #6615 ) ) ;
#4247=EDGE_LOOP ( 'NONE', ( #9993, #8057, #5079, #5148 ) ) ;
#4248=DIRECTION ( 'NONE',  ( 0.000000000000000000, 0.000000000000000000, -1.000000000000000000 ) ) ;
#4252=CARTESIAN_POINT ( 'NONE',  ( -61.56765823437498852, 8.348958332991934128, 2.248837904296538515 ) ) ;
#4253=CARTESIAN_POINT ( 'NONE',  ( -60.99999999999998579, 14.24999999999999822, 1.500000000000002220 ) ) ;
#4254=CARTESIAN_POINT ( 'NONE',  ( -62.86468353124999453, 12.51562499965860198, 1.500000000000002220 ) ) ;
#4255=CARTESIAN_POINT ( 'NONE',  ( -61.99999999999998579, 12.90624999931720218, 2.500000000000002665 ) ) ;
#4257=CARTESIAN_POINT ( 'NONE',  ( -60.99999999999998579, 10.94791666598387181, 2.077350269189628840 ) ) ;
#4261=CARTESIAN_POINT ( 'NONE',  ( -62.43234176562499016, 15.49479166632526628, 2.248837904296538071 ) ) ;
#4263=CARTESIAN_POINT ( 'NONE',  ( -60.99999999999998579, 12.48958333265053611, 0.9226497308103762673 ) ) ;
#4264=CARTESIAN_POINT ( 'NONE',  ( -62.26794919243111792, 8.823664549684632874, 0.5000000000000059952 ) ) ;
#4265=CARTESIAN_POINT ( 'NONE',  ( -61.99999999999999289, 12.57812499965860198, 2.498450539062049724 ) ) ;
#4266=CARTESIAN_POINT ( 'NONE',  ( -61.13531646874998415, 8.598958332991934128, 1.000774730468978468 ) ) ;
#4270=CARTESIAN_POINT ( 'NONE',  ( -61.13531646874998415, 9.390624999658600203, 1.500000000000002220 ) ) ;
#4271=EDGE_LOOP ( 'NONE', ( #4562, #1864, #7127, #6830 ) ) ;
#4273=CARTESIAN_POINT ( 'NONE',  ( -61.73205080756886076, 12.91741454900183328, 2.500000000000003109 ) ) ;
#4275=CARTESIAN_POINT ( 'NONE',  ( -61.13531646874998415, 15.57812499965860198, 1.500000000000002220 ) ) ;
#4276=CARTESIAN_POINT ( 'NONE',  ( -62.86468353124999453, 10.95312499965860020, 1.500000000000002220 ) ) ;
#4277=CARTESIAN_POINT ( 'NONE',  ( -61.13531646874997705, 15.36979166632526805, 1.999225269531026417 ) ) ;
#4280=CARTESIAN_POINT ( 'NONE',  ( -60.99999999999998579, 14.72916666666666607, 2.077350269189628840 ) ) ;
#4281=EDGE_CURVE ( 'NONE', #470, #5639, #133, .T. ) ;
#4282=CARTESIAN_POINT ( 'NONE',  ( -62.86468353124999453, 9.015624999658601979, 1.500000000000002220 ) ) ;
#4283=CARTESIAN_POINT ( 'NONE',  ( -61.99999999999998579, 13.65624999931720218, 2.654700538379254571 ) ) ;
#4285=ORIENTED_EDGE ( 'NONE', *, *, #4412, .F. ) ;
#4287=CARTESIAN_POINT ( 'NONE',  ( -61.73205080756886076, 9.698664549684629321, 2.500000000000003109 ) ) ;
#4288=CARTESIAN_POINT ( 'NONE',  ( -61.56765823437498142, 11.61979166632526805, 0.7511620957034663704 ) ) ;
#4290=( BOUNDED_CURVE ( )  B_SPLINE_CURVE ( 2, ( #8591, #971, #7876, #7097, #1982, #7989, #196, #374, #257 ),
 .UNSPECIFIED., .F., .F. ) 
 B_SPLINE_CURVE_WITH_KNOTS ( ( 3, 2, 2, 2, 3 ),
 ( 0.7265625000000000000, 0.7291666666666666297, 0.7343750000000000000, 0.7395833333333333703, 0.7421875000000000000 ),
 .UNSPECIFIED. ) 
 CURVE ( )  GEOMETRIC_REPRESENTATION_ITEM ( )  RATIONAL_B_SPLINE_CURVE ( ( 0.9330127018922194093, 0.9330127018922194093, 1.000000000000000000, 0.8660254037844387076, 1.000000000000000000, 0.8660254037844387076, 1.000000000000000000, 0.9330127018922194093, 0.9330127018922194093 ) ) 
 REPRESENTATION_ITEM ( '' )  );
#4291=CARTESIAN_POINT ( 'NONE',  ( -61.99999999999998579, 11.53124999931720218, 0.5000000000000013323 ) ) ;
#4294=CARTESIAN_POINT ( 'NONE',  ( -61.13531646874998415, 13.36979166632526628, 1.999225269531026417 ) ) ;
#4295=CARTESIAN_POINT ( 'NONE',  ( -60.99999999999998579, 11.46874999931720218, 1.500000000000002220 ) ) ;
#4296=CARTESIAN_POINT ( 'NONE',  ( -61.99999999999998579, 9.906249999317203958, 2.654700538379254571 ) ) ;
#4297=ORIENTED_EDGE ( 'NONE', *, *, #497, .T. ) ;
#4303=CARTESIAN_POINT ( 'NONE',  ( -61.13531646874998415, 11.09895833299193413, 1.000774730468978468 ) ) ;
#4306=CARTESIAN_POINT ( 'NONE',  ( -62.43234176562498305, 9.473958332991935904, 0.7511620957034662593 ) ) ;
#4307=CARTESIAN_POINT ( 'NONE',  ( -61.99999999999998579, 13.90624999931720218, 2.500000000000002665 ) ) ;
#4309=CARTESIAN_POINT ( 'NONE',  ( -61.99999999999998579, 13.20312499965860198, 0.5015494609379544944 ) ) ;
#4310=CARTESIAN_POINT ( 'NONE',  ( -60.99999999999998579, 8.239583332650536107, 0.9226497308103762673 ) ) ;
#4311=VERTEX_POINT ( 'NONE', #4291 ) ;
#4313=ORIENTED_EDGE ( 'NONE', *, *, #2354, .F. ) ;
#4314=CARTESIAN_POINT ( 'NONE',  ( -61.49999999999998579, 14.26041666598387003, 0.6339745962155628467 ) ) ;
#4315=CARTESIAN_POINT ( 'NONE',  ( -61.13531646874998415, 14.84895833299193413, 1.000774730468978468 ) ) ;
#4316=CARTESIAN_POINT ( 'NONE',  ( -62.99999999999998579, 8.864583332650536107, 2.077350269189627952 ) ) ;
#4317=CARTESIAN_POINT ( 'NONE',  ( -61.99999999999998579, 16.00000000000000000, 0.5000000000000041078 ) ) ;
#4319=CARTESIAN_POINT ( 'NONE',  ( -61.99999999999999289, 14.20312499965860198, 0.5015494609379544944 ) ) ;
#4321=CARTESIAN_POINT ( 'NONE',  ( -62.43234176562499016, 8.744791666325268054, 2.248837904296538071 ) ) ;
#4322=CARTESIAN_POINT ( 'NONE',  ( -61.99999999999998579, 15.06249999999999822, 0.5000000000000013323 ) ) ;
#4324=CARTESIAN_POINT ( 'NONE',  ( -62.43234176562498305, 9.473958332991935904, 0.7511620957034662593 ) ) ;
#4328=CARTESIAN_POINT ( 'NONE',  ( -61.99999999999998579, 12.90624999931720218, 2.500000000000002665 ) ) ;
#4329=CARTESIAN_POINT ( 'NONE',  ( -61.13531646874997705, 15.80729166632526628, 1.999225269531026417 ) ) ;
#4330=CARTESIAN_POINT ( 'NONE',  ( -61.13531646874998415, 10.59895833299193413, 1.000774730468978468 ) ) ;
#4331=CARTESIAN_POINT ( 'NONE',  ( -61.99999999999999289, 9.515624999658600203, 2.498450539062049724 ) ) ;
#4332=ORIENTED_EDGE ( 'NONE', *, *, #9866, .T. ) ;
#4333=CARTESIAN_POINT ( 'NONE',  ( -60.99999999999998579, 15.72916666666666785, 2.077350269189628840 ) ) ;
#4334=CARTESIAN_POINT ( 'NONE',  ( -62.43234176562498305, 10.72395833299193413, 0.7511620957034662593 ) ) ;
#4336=CARTESIAN_POINT ( 'NONE',  ( -61.49999999999998579, 12.92708333265053611, 2.366025403784441927 ) ) ;
#4340=CARTESIAN_POINT ( 'NONE',  ( -62.86468353124999453, 11.95312499965860198, 1.500000000000002220 ) ) ;
#4341=FACE_OUTER_BOUND ( 'NONE', #986, .T. ) ;
#4342=CARTESIAN_POINT ( 'NONE',  ( -61.73205080756886076, 15.44866454968462932, 2.500000000000003109 ) ) ;
#4345=CARTESIAN_POINT ( 'NONE',  ( -61.99999999999998579, 12.70312499965860198, 0.5015494609379544944 ) ) ;
#4348=CARTESIAN_POINT ( 'NONE',  ( -62.49999999999998579, 8.635416665983868256, 2.366025403784441483 ) ) ;
#4352=EDGE_CURVE ( 'NONE', #8495, #7998, #5985, .T. ) ;
#4353=( BOUNDED_CURVE ( )  B_SPLINE_CURVE ( 2, ( #3781, #8956, #6400, #4715, #9553, #8123, #9724, #9786, #5556 ),
 .UNSPECIFIED., .F., .T. ) 
 B_SPLINE_CURVE_WITH_KNOTS ( ( 3, 2, 2, 2, 3 ),
 ( 0.4921875000000000000, 0.4947916666666666852, 0.5000000000000000000, 0.5052083333333333703, 0.5078125000000000000 ),
 .UNSPECIFIED. ) 
 CURVE ( )  GEOMETRIC_REPRESENTATION_ITEM ( )  RATIONAL_B_SPLINE_CURVE ( ( 0.9330127018922194093, 0.9330127018922194093, 1.000000000000000000, 0.8660254037844387076, 1.000000000000000000, 0.8660254037844387076, 1.000000000000000000, 0.9330127018922194093, 0.9330127018922194093 ) ) 
 REPRESENTATION_ITEM ( '' )  );
#4354=CARTESIAN_POINT ( 'NONE',  ( -62.86468353124998032, 11.18229166632526983, 1.000774730468978246 ) ) ;
#4355=ORIENTED_EDGE ( 'NONE', *, *, #4171, .F. ) ;
#4356=CARTESIAN_POINT ( 'NONE',  ( -62.43234176562499016, 9.307291666325268054, 2.248837904296538071 ) ) ;
#4358=CARTESIAN_POINT ( 'NONE',  ( -62.86468353124999453, 15.01562499965860020, 1.500000000000002220 ) ) ;
#4359=EDGE_CURVE ( 'NONE', #3891, #5034, #7313, .T. ) ;
#4367=CARTESIAN_POINT ( 'NONE',  ( -61.99999999999998579, 8.562500000000001776, 0.3452994616207497591 ) ) ;
#4368=CARTESIAN_POINT ( 'NONE',  ( -62.26794919243111082, 9.823664549684629321, 0.5000000000000013323 ) ) ;
#4372=CARTESIAN_POINT ( 'NONE',  ( -62.86468353124999453, 14.28645833299193413, 1.999225269531025750 ) ) ;
#4373=CARTESIAN_POINT ( 'NONE',  ( -61.99999999999998579, 9.390624999658600203, 0.5015494609379544944 ) ) ;
#4375=CARTESIAN_POINT ( 'NONE',  ( -62.26794919243111082, 15.79241454900183506, 0.5000000000000013323 ) ) ;
#4376=CARTESIAN_POINT ( 'NONE',  ( -62.43234176562499016, 8.557291666325268054, 2.248837904296538071 ) ) ;
#4378=CARTESIAN_POINT ( 'NONE',  ( -62.26794919243111082, 14.14508544963257286, 2.500000000000003109 ) ) ;
#4379=ORIENTED_EDGE ( 'NONE', *, *, #4633, .F. ) ;
#4381=CARTESIAN_POINT ( 'NONE',  ( -61.49999999999998579, 11.26041666598387003, 0.6339745962155628467 ) ) ;
#4382=EDGE_CURVE ( 'NONE', #5639, #2471, #5465, .T. ) ;
#4383=CARTESIAN_POINT ( 'NONE',  ( -62.86468353124999453, 14.95312499965860020, 1.500000000000002220 ) ) ;
#4384=CARTESIAN_POINT ( 'NONE',  ( -62.86468353124998032, 11.43229166632526805, 1.000774730468978246 ) ) ;
#4385=VECTOR ( 'NONE', #7671, 1000.000000000000000 ) ;
#4386=CARTESIAN_POINT ( 'NONE',  ( -61.13531646874997705, 9.098958332991935904, 1.000774730468978468 ) ) ;
#4387=CARTESIAN_POINT ( 'NONE',  ( -60.99999999999998579, 9.697916665983870033, 2.077350269189628840 ) ) ;
#4389=CARTESIAN_POINT ( 'NONE',  ( -61.49999999999998579, 15.04166666666666607, 0.6339745962155628467 ) ) ;
#4390=CARTESIAN_POINT ( 'NONE',  ( -61.13531646874998415, 10.14062499965860198, 1.500000000000002220 ) ) ;
#4392=CARTESIAN_POINT ( 'NONE',  ( -61.99999999999998579, 13.15624999931720396, 2.654700538379254571 ) ) ;
#4395=CARTESIAN_POINT ( 'NONE',  ( -61.99999999999998579, 16.00000000000000000, 1.500000000000002220 ) ) ;
#4399=CARTESIAN_POINT ( 'NONE',  ( -61.99999999999999289, 11.64062499965860198, 0.5015494609379544944 ) ) ;
#4400=CARTESIAN_POINT ( 'NONE',  ( -62.99999999999998579, 15.64583333333333393, 2.077350269189627952 ) ) ;
#4401=APPLICATION_CONTEXT ( 'automotive_design' ) ;
#4402=CARTESIAN_POINT ( 'NONE',  ( -61.49999999999998579, 13.04166666666666607, 0.6339745962155628467 ) ) ;
#4404=CARTESIAN_POINT ( 'NONE',  ( -62.49999999999998579, 10.91666666666666607, 2.366025403784441483 ) ) ;
#4405=CARTESIAN_POINT ( 'NONE',  ( -61.99999999999998579, 16.00000000000000000, 1.500000000000002220 ) ) ;
#4406=AXIS2_PLACEMENT_3D ( 'NONE', #9845, #568, #7232 ) ;
#4407=CARTESIAN_POINT ( 'NONE',  ( -61.99999999999998579, 13.70312499965860198, 0.5015494609379544944 ) ) ;
#4409=CARTESIAN_POINT ( 'NONE',  ( -61.49999999999998579, 10.20833333333333393, 2.366025403784441927 ) ) ;
#4410=CARTESIAN_POINT ( 'NONE',  ( -62.49999999999998579, 9.385416665983870033, 2.366025403784441483 ) ) ;
#4412=EDGE_CURVE ( 'NONE', #5522, #3958, #7146, .T. ) ;
#4413=VERTEX_POINT ( 'NONE', #8204 ) ;
#4415=CARTESIAN_POINT ( 'NONE',  ( -60.99999999999998579, 9.968749999317202182, 1.500000000000002220 ) ) ;
#4417=EDGE_CURVE ( 'NONE', #9464, #35, #6297, .T. ) ;
#4418=CARTESIAN_POINT ( 'NONE',  ( -61.56765823437498142, 10.86979166632526805, 0.7511620957034663704 ) ) ;
#4420=ORIENTED_EDGE ( 'NONE', *, *, #1732, .T. ) ;
#4421=CARTESIAN_POINT ( 'NONE',  ( -61.13531646874998415, 10.39062499965860198, 1.500000000000002220 ) ) ;
#4423=EDGE_CURVE ( 'NONE', #7302, #2222, #6769, .T. ) ;
#4425=CARTESIAN_POINT ( 'NONE',  ( -61.99999999999998579, 14.07812499965860020, 2.498450539062049724 ) ) ;
#4427=CARTESIAN_POINT ( 'NONE',  ( -62.99999999999998579, 12.07291666598387181, 0.9226497308103756012 ) ) ;
#4429=( BOUNDED_CURVE ( )  B_SPLINE_CURVE ( 2, ( #2821, #6210, #6094, #10366, #5301, #4476, #5535, #9823, #1378 ),
 .UNSPECIFIED., .F., .T. ) 
 B_SPLINE_CURVE_WITH_KNOTS ( ( 3, 2, 2, 2, 3 ),
 ( 0.6640625000000000000, 0.6666666666666666297, 0.6718750000000000000, 0.6770833333333333703, 0.6796875000000000000 ),
 .UNSPECIFIED. ) 
 CURVE ( )  GEOMETRIC_REPRESENTATION_ITEM ( )  RATIONAL_B_SPLINE_CURVE ( ( 0.9330127018922194093, 0.9330127018922194093, 1.000000000000000000, 0.8660254037844387076, 1.000000000000000000, 0.8660254037844387076, 1.000000000000000000, 0.9330127018922194093, 0.9330127018922194093 ) ) 
 REPRESENTATION_ITEM ( '' )  );
#4430=CARTESIAN_POINT ( 'NONE',  ( -61.99999999999998579, 10.56249999999999822, 0.5000000000000013323 ) ) ;
#4431=ORIENTED_EDGE ( 'NONE', *, *, #5763, .F. ) ;
#4432=CARTESIAN_POINT ( 'NONE',  ( -60.99999999999998579, 12.73958333265053611, 0.9226497308103762673 ) ) ;
#4433=CARTESIAN_POINT ( 'NONE',  ( -61.99999999999998579, 8.312500000000000000, 0.3452994616207497591 ) ) ;
#4434=CARTESIAN_POINT ( 'NONE',  ( -62.99999999999998579, 8.822916665983868256, 0.9226497308103756012 ) ) ;
#4437=CARTESIAN_POINT ( 'NONE',  ( -62.43234176562499016, 13.80729166632526805, 2.248837904296538071 ) ) ;
#4438=CARTESIAN_POINT ( 'NONE',  ( -61.56765823437498142, 8.619791666325268054, 0.7511620957034663704 ) ) ;
#4439=CARTESIAN_POINT ( 'NONE',  ( -61.73205080756886787, 9.198664549684631098, 2.500000000000004885 ) ) ;
#4441=CARTESIAN_POINT ( 'NONE',  ( -61.99999999999998579, 10.45312499965860198, 0.5015494609379544944 ) ) ;
#4443=ORIENTED_EDGE ( 'NONE', *, *, #7358, .T. ) ;
#4445=CARTESIAN_POINT ( 'NONE',  ( -60.99999999999998579, 12.96874999931720396, 1.500000000000002220 ) ) ;
#4447=DIRECTION ( 'NONE',  ( -0.000000000000000000, -1.000000000000000000, -0.000000000000000000 ) ) ;
#4448=CARTESIAN_POINT ( 'NONE',  ( -62.86468353124998742, 12.47395833299193413, 1.999225269531025972 ) ) ;
#4449=EDGE_CURVE ( 'NONE', #6224, #6875, #9645, .T. ) ;
#4450=CARTESIAN_POINT ( 'NONE',  ( -62.43234176562499016, 9.244791666325268054, 2.248837904296538071 ) ) ;
#4451=CARTESIAN_POINT ( 'NONE',  ( -60.99999999999998579, 9.718749999317202182, 1.500000000000002220 ) ) ;
#4452=VERTEX_POINT ( 'NONE', #1196 ) ;
#4453=CARTESIAN_POINT ( 'NONE',  ( -62.49999999999998579, 10.80208333265053611, 0.6339745962155627357 ) ) ;
#4455=CARTESIAN_POINT ( 'NONE',  ( -61.99999999999999289, 9.453124999658600203, 0.5015494609379544944 ) ) ;
#4457=CARTESIAN_POINT ( 'NONE',  ( -61.13531646874998415, 15.82812499965860198, 1.500000000000002220 ) ) ;
#4458=CARTESIAN_POINT ( 'NONE',  ( -60.99999999999998579, 14.94791666598387003, 2.077350269189628840 ) ) ;
#4459=CARTESIAN_POINT ( 'NONE',  ( -61.99999999999998579, 13.18750000000000000, 2.500000000000002665 ) ) ;
#4463=CARTESIAN_POINT ( 'NONE',  ( -62.86468353124998032, 11.93229166632526628, 1.000774730468978024 ) ) ;
#4464=CARTESIAN_POINT ( 'NONE',  ( -62.86468353124998032, 9.182291666325268054, 1.000774730468978246 ) ) ;
#4467=CARTESIAN_POINT ( 'NONE',  ( -62.99999999999998579, 10.85416666666666785, 0.9226497308103756012 ) ) ;
#4469=CARTESIAN_POINT ( 'NONE',  ( -61.99999999999998579, 14.07812499965860020, 2.498450539062049724 ) ) ;
#4471=EDGE_CURVE ( 'NONE', #6004, #5909, #3040, .T. ) ;
#4473=CARTESIAN_POINT ( 'NONE',  ( -61.99999999999998579, 8.781249999317203958, 0.3452994616207497591 ) ) ;
#4474=EDGE_LOOP ( 'NONE', ( #4016, #3685, #8431, #2170 ) ) ;
#4476=CARTESIAN_POINT ( 'NONE',  ( -62.99999999999998579, 13.39583333333333393, 2.077350269189627952 ) ) ;
#4477=VECTOR ( 'NONE', #6427, 1000.000000000000000 ) ;
#4478=CARTESIAN_POINT ( 'NONE',  ( -62.43234176562499016, 10.99479166632526805, 2.248837904296538071 ) ) ;
#4481=CARTESIAN_POINT ( 'NONE',  ( -61.56765823437498852, 9.848958332991934128, 2.248837904296538515 ) ) ;
#4482=CARTESIAN_POINT ( 'NONE',  ( -62.99999999999998579, 15.61458333265053433, 2.077350269189627952 ) ) ;
#4483=CARTESIAN_POINT ( 'NONE',  ( -62.86468353124998032, 14.74479166632526628, 1.000774730468978246 ) ) ;
#4484=CARTESIAN_POINT ( 'NONE',  ( -61.99999999999998579, 11.18750000000000000, 2.500000000000002665 ) ) ;
#4489=FACE_OUTER_BOUND ( 'NONE', #9665, .T. ) ;
#4490=CARTESIAN_POINT ( 'NONE',  ( -61.49999999999998579, 8.791666666666666075, 0.6339745962155628467 ) ) ;
#4491=FACE_OUTER_BOUND ( 'NONE', #5816, .T. ) ;
#4494=CARTESIAN_POINT ( 'NONE',  ( -62.86468353124998032, 13.74479166632526805, 1.000774730468978024 ) ) ;
#4495=CARTESIAN_POINT ( 'NONE',  ( -61.99999999999998579, 9.515624999658601979, 2.498450539062049724 ) ) ;
#4496=CARTESIAN_POINT ( 'NONE',  ( -61.99999999999997868, 11.28124999931720041, 0.5000000000000013323 ) ) ;
#4497=( BOUNDED_CURVE ( )  B_SPLINE_CURVE ( 2, ( #10631, #681, #3030, #4065, #3133, #1365, #3230, #6530, #9912 ),
 .UNSPECIFIED., .F., .T. ) 
 B_SPLINE_CURVE_WITH_KNOTS ( ( 3, 2, 2, 2, 3 ),
 ( 0.8828125000000000000, 0.8854166666666666297, 0.8906250000000000000, 0.8958333333333333703, 0.8984375000000000000 ),
 .UNSPECIFIED. ) 
 CURVE ( )  GEOMETRIC_REPRESENTATION_ITEM ( )  RATIONAL_B_SPLINE_CURVE ( ( 0.9330127018922194093, 0.9330127018922194093, 1.000000000000000000, 0.8660254037844387076, 1.000000000000000000, 0.8660254037844387076, 1.000000000000000000, 0.9330127018922194093, 0.9330127018922194093 ) ) 
 REPRESENTATION_ITEM ( '' )  );
#4499=CARTESIAN_POINT ( 'NONE',  ( -61.13531646874998415, 10.14062499965860198, 1.500000000000002220 ) ) ;
#4503=CARTESIAN_POINT ( 'NONE',  ( -61.99999999999997868, 11.43750000000000000, 2.500000000000002665 ) ) ;
#4506=CARTESIAN_POINT ( 'NONE',  ( -61.99999999999998579, 12.76562499965860198, 2.498450539062049724 ) ) ;
#4507=CARTESIAN_POINT ( 'NONE',  ( -62.43234176562499016, 8.744791666325268054, 2.248837904296538071 ) ) ;
#4509=VERTEX_POINT ( 'NONE', #7527 ) ;
#4510=CARTESIAN_POINT ( 'NONE',  ( -61.99999999999998579, 10.78124999931720218, 0.5000000000000013323 ) ) ;
#4511=CARTESIAN_POINT ( 'NONE',  ( -62.43234176562498305, 9.973958332991934128, 0.7511620957034662593 ) ) ;
#4513=CARTESIAN_POINT ( 'NONE',  ( -62.43234176562499016, 14.99479166632526805, 2.248837904296538071 ) ) ;
#4514=CARTESIAN_POINT ( 'NONE',  ( -61.49999999999998579, 14.17708333265053611, 2.366025403784441927 ) ) ;
#4518=EDGE_LOOP ( 'NONE', ( #8155, #8199, #1817, #5806 ) ) ;
#4520=CARTESIAN_POINT ( 'NONE',  ( -62.86468353124999453, 12.45312499965860198, 1.500000000000002220 ) ) ;
#4521=DIRECTION ( 'NONE',  ( 0.000000000000000000, 0.000000000000000000, -1.000000000000000000 ) ) ;
#4524=CARTESIAN_POINT ( 'NONE',  ( -62.99999999999998579, 12.62500000000000000, 1.500000000000001998 ) ) ;
#4525=CYLINDRICAL_SURFACE ( 'NONE', #8560, 0.9999999999999981126 ) ;
#4526=CARTESIAN_POINT ( 'NONE',  ( -61.13531646874998415, 14.91145833299193413, 1.000774730468978468 ) ) ;
#4528=CARTESIAN_POINT ( 'NONE',  ( -62.99999999999998579, 10.61458333265053611, 2.077350269189627952 ) ) ;
#4529=ORIENTED_EDGE ( 'NONE', *, *, #4281, .F. ) ;
#4532=CARTESIAN_POINT ( 'NONE',  ( -61.99999999999998579, 11.26562499965860198, 2.498450539062049724 ) ) ;
#4533=EDGE_CURVE ( 'NONE', #2384, #5580, #6656, .T. ) ;
#4534=ORIENTED_EDGE ( 'NONE', *, *, #4812, .T. ) ;
#4535=CARTESIAN_POINT ( 'NONE',  ( -61.99999999999998579, 10.07812499965860198, 2.498450539062049724 ) ) ;
#4537=CARTESIAN_POINT ( 'NONE',  ( -62.86468353124998032, 14.49479166632526805, 1.000774730468978246 ) ) ;
#4541=VERTEX_POINT ( 'NONE', #5012 ) ;
#4542=CARTESIAN_POINT ( 'NONE',  ( -62.99999999999998579, 15.07291666598387003, 0.9226497308103756012 ) ) ;
#4543=CARTESIAN_POINT ( 'NONE',  ( -60.99999999999998579, 8.020833333333333925, 0.9226497308103762673 ) ) ;
#4545=CARTESIAN_POINT ( 'NONE',  ( -61.99999999999998579, 16.15624999931720041, 2.500000000000002665 ) ) ;
#4546=CYLINDRICAL_SURFACE ( 'NONE', #9922, 0.9999999999999981126 ) ;
#4547=CARTESIAN_POINT ( 'NONE',  ( -61.56765823437498142, 14.68229166632526805, 0.7511620957034663704 ) ) ;
#4548=CARTESIAN_POINT ( 'NONE',  ( -62.86468353124999453, 10.20312499965860198, 1.500000000000002220 ) ) ;
#4551=CARTESIAN_POINT ( 'NONE',  ( -61.13531646874998415, 10.66145833299193413, 1.000774730468978468 ) ) ;
#4552=CARTESIAN_POINT ( 'NONE',  ( -61.99999999999998579, 9.562500000000000000, 0.5000000000000013323 ) ) ;
#4553=ORIENTED_EDGE ( 'NONE', *, *, #3905, .F. ) ;
#4557=CARTESIAN_POINT ( 'NONE',  ( -60.99999999999998579, 10.00000000000000000, 1.500000000000002220 ) ) ;
#4558=CARTESIAN_POINT ( 'NONE',  ( -62.86468353124998742, 12.22395833299193413, 1.999225269531025972 ) ) ;
#4559=CARTESIAN_POINT ( 'NONE',  ( -61.13531646874998415, 8.828124999658601979, 1.500000000000002220 ) ) ;
#4560=CARTESIAN_POINT ( 'NONE',  ( -61.99999999999998579, 26.00000000000000355, 1.500000000000002220 ) ) ;
#4561=( BOUNDED_CURVE ( )  B_SPLINE_CURVE ( 2, ( #987, #7668, #5043, #9435, #10156, #6048, #1834, #8393, #7612 ),
 .UNSPECIFIED., .F., .T. ) 
 B_SPLINE_CURVE_WITH_KNOTS ( ( 3, 2, 2, 2, 3 ),
 ( 0.6171875000000000000, 0.6197916666666666297, 0.6250000000000000000, 0.6302083333333333703, 0.6328125000000000000 ),
 .UNSPECIFIED. ) 
 CURVE ( )  GEOMETRIC_REPRESENTATION_ITEM ( )  RATIONAL_B_SPLINE_CURVE ( ( 0.9330127018922194093, 0.9330127018922194093, 1.000000000000000000, 0.8660254037844387076, 1.000000000000000000, 0.8660254037844387076, 1.000000000000000000, 0.9330127018922194093, 0.9330127018922194093 ) ) 
 REPRESENTATION_ITEM ( '' )  );
#4562=ORIENTED_EDGE ( 'NONE', *, *, #10476, .F. ) ;
#4564=CARTESIAN_POINT ( 'NONE',  ( -62.86468353124998032, 9.994791666325268054, 1.000774730468978024 ) ) ;
#4566=CARTESIAN_POINT ( 'NONE',  ( -61.56765823437498852, 15.78645833299193590, 2.248837904296538515 ) ) ;
#4568=CARTESIAN_POINT ( 'NONE',  ( -62.99999999999998579, 15.09374999931720218, 1.500000000000001998 ) ) ;
#4569=CARTESIAN_POINT ( 'NONE',  ( -61.99999999999998579, 16.03124999931720041, 0.5000000000000013323 ) ) ;
#4570=VERTEX_POINT ( 'NONE', #3345 ) ;
#4573=CARTESIAN_POINT ( 'NONE',  ( -61.13531646874997705, 12.34895833299193413, 1.000774730468978468 ) ) ;
#4574=CARTESIAN_POINT ( 'NONE',  ( -61.56765823437498852, 8.536458332991934128, 2.248837904296538515 ) ) ;
#4575=AXIS2_PLACEMENT_3D ( 'NONE', #609, #3884, #7277 ) ;
#4578=CARTESIAN_POINT ( 'NONE',  ( -61.49999999999998579, 12.70833333333333393, 2.366025403784441927 ) ) ;
#4580=CARTESIAN_POINT ( 'NONE',  ( -61.99999999999998579, 14.45312499965860020, 0.5015494609379544944 ) ) ;
#4584=CARTESIAN_POINT ( 'NONE',  ( -60.99999999999998579, 11.21874999931720218, 1.500000000000002220 ) ) ;
#4586=DIRECTION ( 'NONE',  ( 0.000000000000000000, 0.000000000000000000, -1.000000000000000000 ) ) ;
#4589=CARTESIAN_POINT ( 'NONE',  ( -61.56765823437498142, 12.11979166632526628, 0.7511620957034663704 ) ) ;
#4590=EDGE_CURVE ( 'NONE', #918, #8781, #9088, .T. ) ;
#4595=CARTESIAN_POINT ( 'NONE',  ( -61.56765823437498852, 10.59895833299193413, 2.248837904296538515 ) ) ;
#4598=CARTESIAN_POINT ( 'NONE',  ( -62.86468353124999453, 14.51562499965860020, 1.500000000000002220 ) ) ;
#4599=FACE_OUTER_BOUND ( 'NONE', #4247, .T. ) ;
#4602=VERTEX_POINT ( 'NONE', #5746 ) ;
#4603=DIRECTION ( 'NONE',  ( -0.000000000000000000, -1.000000000000000000, -0.000000000000000000 ) ) ;
#4604=CARTESIAN_POINT ( 'NONE',  ( -61.49999999999998579, 8.041666666666667851, 0.6339745962155628467 ) ) ;
#4607=LINE ( 'NONE', #9610, #7435 ) ;
#4609=CARTESIAN_POINT ( 'NONE',  ( -62.43234176562499016, 14.80729166632526805, 2.248837904296538071 ) ) ;
#4610=CARTESIAN_POINT ( 'NONE',  ( -62.86468353124998032, 9.932291666325269830, 1.000774730468978246 ) ) ;
#4615=ADVANCED_FACE ( 'NONE', ( #5852 ), #5063, .T. ) ;
#4616=CARTESIAN_POINT ( 'NONE',  ( -61.99999999999998579, 11.07812499965860020, 2.498450539062049724 ) ) ;
#4619=CARTESIAN_POINT ( 'NONE',  ( -62.26794919243111082, 14.32366454968462932, 0.5000000000000013323 ) ) ;
#4623=CARTESIAN_POINT ( 'NONE',  ( -61.99999999999998579, 10.28124999931720218, 0.5000000000000013323 ) ) ;
#4624=CARTESIAN_POINT ( 'NONE',  ( -62.43234176562498305, 13.16145833299193413, 0.7511620957034662593 ) ) ;
#4625=CARTESIAN_POINT ( 'NONE',  ( -62.43234176562499016, 10.24479166632526805, 2.248837904296538071 ) ) ;
#4627=CARTESIAN_POINT ( 'NONE',  ( -62.86468353124998032, 11.49479166632526805, 1.000774730468978024 ) ) ;
#4629=CARTESIAN_POINT ( 'NONE',  ( -61.99999999999998579, 15.01562499965860198, 2.498450539062049724 ) ) ;
#4630=CARTESIAN_POINT ( 'NONE',  ( -60.99999999999998579, 14.44791666598387003, 2.077350269189628840 ) ) ;
#4631=CARTESIAN_POINT ( 'NONE',  ( -60.99999999999998579, 14.69791666598386826, 2.077350269189628840 ) ) ;
#4633=EDGE_CURVE ( 'NONE', #5222, #3446, #6539, .T. ) ;
#4634=CYLINDRICAL_SURFACE ( 'NONE', #1649, 0.9999999999999981126 ) ;
#4635=ORIENTED_EDGE ( 'NONE', *, *, #3970, .T. ) ;
#4636=( BOUNDED_CURVE ( )  B_SPLINE_CURVE ( 2, ( #9321, #4310, #7827, #823, #98 ),
 .UNSPECIFIED., .F., .T. ) 
 B_SPLINE_CURVE_WITH_KNOTS ( ( 3, 2, 3 ),
 ( 0.000000000000000000, 0.005208333333333333044, 0.007812499999999973112 ),
 .UNSPECIFIED. ) 
 CURVE ( )  GEOMETRIC_REPRESENTATION_ITEM ( )  RATIONAL_B_SPLINE_CURVE ( ( 1.000000000000000000, 0.8660254037844387076, 1.000000000000000000, 0.9330127018922200755, 0.9330127018922194093 ) ) 
 REPRESENTATION_ITEM ( '' )  );
#4637=CARTESIAN_POINT ( 'NONE',  ( -61.56765823437498142, 12.86979166632526805, 0.7511620957034663704 ) ) ;
#4638=CARTESIAN_POINT ( 'NONE',  ( -61.13531646874998415, 9.098958332991934128, 1.000774730468978468 ) ) ;
#4639=DIRECTION ( 'NONE',  ( -0.000000000000000000, -1.000000000000000000, -0.000000000000000000 ) ) ;
#4640=ORIENTED_EDGE ( 'NONE', *, *, #7550, .F. ) ;
#4641=CARTESIAN_POINT ( 'NONE',  ( -60.99999999999998579, 13.02083333333333215, 0.9226497308103762673 ) ) ;
#4643=CARTESIAN_POINT ( 'NONE',  ( -61.13531646874998415, 14.14062499965860198, 1.500000000000002220 ) ) ;
#4644=CARTESIAN_POINT ( 'NONE',  ( -62.49999999999998579, 14.30208333265053611, 0.6339745962155627357 ) ) ;
#4645=CARTESIAN_POINT ( 'NONE',  ( -61.49999999999998579, 10.67708333265053611, 2.366025403784441927 ) ) ;
#4647=CARTESIAN_POINT ( 'NONE',  ( -62.99999999999998579, 14.85416666666666607, 0.9226497308103756012 ) ) ;
#4648=CARTESIAN_POINT ( 'NONE',  ( -62.86468353124998742, 12.97395833299193413, 1.999225269531025972 ) ) ;
#4652=CARTESIAN_POINT ( 'NONE',  ( -61.56765823437498852, 10.09895833299193413, 2.248837904296538515 ) ) ;
#4655=CARTESIAN_POINT ( 'NONE',  ( -60.99999999999998579, 8.947916665983868256, 2.077350269189628840 ) ) ;
#4657=DIRECTION ( 'NONE',  ( -0.000000000000000000, -1.000000000000000000, -0.000000000000000000 ) ) ;
#4660=CARTESIAN_POINT ( 'NONE',  ( -62.26794919243111082, 15.14508544963257108, 2.500000000000003109 ) ) ;
#4661=CARTESIAN_POINT ( 'NONE',  ( -62.99999999999998579, 10.12500000000000000, 1.500000000000001998 ) ) ;
#4662=CARTESIAN_POINT ( 'NONE',  ( -61.99999999999998579, 11.18750000000000000, 2.500000000000002665 ) ) ;
#4664=( BOUNDED_CURVE ( )  B_SPLINE_CURVE ( 2, ( #9358, #8476, #10083, #3470, #4295, #5027, #6660, #10239, #709 ),
 .UNSPECIFIED., .F., .F. ) 
 B_SPLINE_CURVE_WITH_KNOTS ( ( 3, 2, 2, 2, 3 ),
 ( 0.3984375000000000000, 0.4010416666666666852, 0.4062500000000000000, 0.4114583333333333148, 0.4140625000000000000 ),
 .UNSPECIFIED. ) 
 CURVE ( )  GEOMETRIC_REPRESENTATION_ITEM ( )  RATIONAL_B_SPLINE_CURVE ( ( 0.9330127018922194093, 0.9330127018922194093, 1.000000000000000000, 0.8660254037844387076, 1.000000000000000000, 0.8660254037844387076, 1.000000000000000000, 0.9330127018922194093, 0.9330127018922194093 ) ) 
 REPRESENTATION_ITEM ( '' )  );
#4667=CARTESIAN_POINT ( 'NONE',  ( -62.86468353124998742, 10.22395833299193413, 1.999225269531025972 ) ) ;
#4669=CARTESIAN_POINT ( 'NONE',  ( -61.56765823437498142, 10.68229166632526805, 0.7511620957034663704 ) ) ;
#4673=CARTESIAN_POINT ( 'NONE',  ( -62.49999999999998579, 9.166666666666666075, 2.366025403784441483 ) ) ;
#4675=ORIENTED_EDGE ( 'NONE', *, *, #10296, .T. ) ;
#4676=CARTESIAN_POINT ( 'NONE',  ( -60.99999999999998579, 10.23958333265053788, 0.9226497308103762673 ) ) ;
#4678=CARTESIAN_POINT ( 'NONE',  ( -62.86468353124998742, 12.97395833299193413, 1.999225269531025972 ) ) ;
#4679=CARTESIAN_POINT ( 'NONE',  ( -61.56765823437498852, 10.28645833299193413, 2.248837904296538515 ) ) ;
#4682=CARTESIAN_POINT ( 'NONE',  ( -60.99999999999998579, 8.447916665983870033, 2.077350269189628840 ) ) ;
#4683=CARTESIAN_POINT ( 'NONE',  ( -62.43234176562499016, 11.55729166632526805, 2.248837904296538071 ) ) ;
#4685=CARTESIAN_POINT ( 'NONE',  ( -62.43234176562498305, 15.41145833299193590, 0.7511620957034662593 ) ) ;
#4686=CARTESIAN_POINT ( 'NONE',  ( -62.99999999999998579, 14.86458333265053611, 2.077350269189627952 ) ) ;
#4688=ORIENTED_EDGE ( 'NONE', *, *, #7597, .F. ) ;
#4691=CARTESIAN_POINT ( 'NONE',  ( -61.56765823437498142, 13.36979166632526805, 0.7511620957034663704 ) ) ;
#4692=CARTESIAN_POINT ( 'NONE',  ( -62.43234176562498305, 8.161458332991934128, 0.7511620957034662593 ) ) ;
#4693=CARTESIAN_POINT ( 'NONE',  ( -61.49999999999998579, 11.70833333333333215, 2.366025403784441927 ) ) ;
#4695=CARTESIAN_POINT ( 'NONE',  ( -61.49999999999998579, 12.04166666666666607, 0.6339745962155628467 ) ) ;
#4696=CARTESIAN_POINT ( 'NONE',  ( -62.99999999999998579, 11.11458333265053611, 2.077350269189627952 ) ) ;
#4699=CARTESIAN_POINT ( 'NONE',  ( -62.49999999999998579, 10.13541666598387003, 2.366025403784441483 ) ) ;
#4700=VERTEX_POINT ( 'NONE', #1477 ) ;
#4703=CARTESIAN_POINT ( 'NONE',  ( -61.13531646874998415, 12.05729166632526628, 1.999225269531026417 ) ) ;
#4705=CARTESIAN_POINT ( 'NONE',  ( -62.86468353124998032, 11.49479166632526805, 1.000774730468978246 ) ) ;
#4706=CARTESIAN_POINT ( 'NONE',  ( -61.49999999999998579, 12.17708333265053611, 2.366025403784441927 ) ) ;
#4708=CARTESIAN_POINT ( 'NONE',  ( -61.13531646874998415, 15.36979166632526983, 1.999225269531026417 ) ) ;
#4710=EDGE_LOOP ( 'NONE', ( #10272, #7654, #7633 ) ) ;
#4711=DIRECTION ( 'NONE',  ( -0.000000000000000000, -1.000000000000000000, -0.000000000000000000 ) ) ;
#4713=CARTESIAN_POINT ( 'NONE',  ( -60.99999999999998579, 9.479166666666666075, 2.077350269189628840 ) ) ;
#4715=CARTESIAN_POINT ( 'NONE',  ( -60.99999999999998579, 11.97916666666666785, 2.077350269189628840 ) ) ;
#4716=FACE_OUTER_BOUND ( 'NONE', #9096, .T. ) ;
#4717=CARTESIAN_POINT ( 'NONE',  ( -61.13531646874998415, 10.57812499965860198, 1.500000000000002220 ) ) ;
#4718=CARTESIAN_POINT ( 'NONE',  ( -60.99999999999998579, 8.218749999317202182, 1.500000000000002220 ) ) ;
#4719=CARTESIAN_POINT ( 'NONE',  ( -61.99999999999998579, 12.32812499965860376, 2.498450539062049724 ) ) ;
#4720=DIRECTION ( 'NONE',  ( 0.000000000000000000, 0.000000000000000000, 1.000000000000000000 ) ) ;
#4722=CARTESIAN_POINT ( 'NONE',  ( -62.99999999999998579, 15.39583333333333393, 2.077350269189627952 ) ) ;
#4724=CARTESIAN_POINT ( 'NONE',  ( -62.49999999999998579, 10.13541666598387003, 2.366025403784441483 ) ) ;
#4725=EDGE_CURVE ( 'NONE', #4541, #5466, #3361, .T. ) ;
#4726=CARTESIAN_POINT ( 'NONE',  ( -62.86468353124999453, 14.20312499965860020, 1.500000000000002220 ) ) ;
#4727=CARTESIAN_POINT ( 'NONE',  ( -62.43234176562499016, 10.74479166632526805, 2.248837904296538071 ) ) ;
#4731=CARTESIAN_POINT ( 'NONE',  ( -61.13531646874998415, 10.89062499965860020, 1.500000000000002220 ) ) ;
#4734=DIRECTION ( 'NONE',  ( -0.000000000000000000, -1.000000000000000000, -0.000000000000000000 ) ) ;
#4735=CARTESIAN_POINT ( 'NONE',  ( -61.99999999999998579, 8.328124999658601979, 2.498450539062049724 ) ) ;
#4739=CARTESIAN_POINT ( 'NONE',  ( -61.38196601871477043, 16.00549858343031673, 0.7021215470841072337 ) ) ;
#4742=CARTESIAN_POINT ( 'NONE',  ( -62.43234176562499016, 13.49479166632526805, 2.248837904296538071 ) ) ;
#4743=CARTESIAN_POINT ( 'NONE',  ( -61.56765823437498142, 9.619791666325268054, 0.7511620957034663704 ) ) ;
#4747=CARTESIAN_POINT ( 'NONE',  ( -61.99999999999998579, 13.06250000000000355, 0.3452994616207497591 ) ) ;
#4750=CARTESIAN_POINT ( 'NONE',  ( -62.99999999999998579, 11.09374999931720218, 1.500000000000001998 ) ) ;
#4754=CARTESIAN_POINT ( 'NONE',  ( -61.99999999999998579, 12.01562499965860020, 2.498450539062049724 ) ) ;
#4756=ORIENTED_EDGE ( 'NONE', *, *, #5697, .F. ) ;
#4757=VECTOR ( 'NONE', #8025, 1000.000000000000000 ) ;
#4758=CARTESIAN_POINT ( 'NONE',  ( -61.13531646874998415, 11.61979166632526983, 1.999225269531026417 ) ) ;
#4759=CARTESIAN_POINT ( 'NONE',  ( -61.99999999999998579, 12.53124999931720396, 0.5000000000000013323 ) ) ;
#4761=CARTESIAN_POINT ( 'NONE',  ( -61.99999999999998579, 8.687500000000000000, 2.500000000000002665 ) ) ;
#4762=VERTEX_POINT ( 'NONE', #182 ) ;
#4763=EDGE_CURVE ( 'NONE', #9934, #1925, #7848, .T. ) ;
#4764=CARTESIAN_POINT ( 'NONE',  ( -61.99999999999998579, 26.00000000000000355, -1.000000000000000000 ) ) ;
#4766=AXIS2_PLACEMENT_3D ( 'NONE', #7840, #7731, #10268 ) ;
#4770=CARTESIAN_POINT ( 'NONE',  ( -62.99999999999998579, 9.854166666666666075, 0.9226497308103756012 ) ) ;
#4772=CARTESIAN_POINT ( 'NONE',  ( -61.99999999999998579, 16.00000000000000000, 1.500000000000002220 ) ) ;
#4774=CARTESIAN_POINT ( 'NONE',  ( -62.99999999999998579, 14.86458333265053611, 2.077350269189627952 ) ) ;
#4776=CARTESIAN_POINT ( 'NONE',  ( -62.49999999999998579, 8.552083332650536107, 0.6339745962155627357 ) ) ;
#4777=CARTESIAN_POINT ( 'NONE',  ( -61.99999999999998579, 11.45312499965860020, 0.5015494609379544944 ) ) ;
#4778=CARTESIAN_POINT ( 'NONE',  ( -62.26794919243111082, 9.145085449632572860, 2.500000000000004885 ) ) ;
#4779=ORIENTED_EDGE ( 'NONE', *, *, #4001, .F. ) ;
#4781=CARTESIAN_POINT ( 'NONE',  ( -61.99999999999998579, 15.18750000000000000, 2.500000000000002665 ) ) ;
#4784=CARTESIAN_POINT ( 'NONE',  ( -61.49999999999998579, 14.17708333265053611, 2.366025403784441927 ) ) ;
#4785=CARTESIAN_POINT ( 'NONE',  ( -61.99999999999998579, 14.39062499965859843, 0.5015494609379544944 ) ) ;
#4786=CARTESIAN_POINT ( 'NONE',  ( -61.13531646874998415, 10.57812499965860198, 1.500000000000002220 ) ) ;
#4787=CARTESIAN_POINT ( 'NONE',  ( -60.99999999999998579, 11.69791666598387181, 2.077350269189628840 ) ) ;
#4788=ORIENTED_EDGE ( 'NONE', *, *, #10096, .T. ) ;
#4789=CARTESIAN_POINT ( 'NONE',  ( -61.99999999999998579, 16.00000000000000000, 2.500000000000000444 ) ) ;
#4790=CARTESIAN_POINT ( 'NONE',  ( -61.13531646874997705, 10.86979166632526805, 1.999225269531026417 ) ) ;
#4791=CARTESIAN_POINT ( 'NONE',  ( -62.99999999999998579, 13.57291666598387359, 0.9226497308103756012 ) ) ;
#4792=VECTOR ( 'NONE', #4146, 1000.000000000000000 ) ;
#4793=CARTESIAN_POINT ( 'NONE',  ( -62.49999999999998579, 15.88541666598386826, 2.366025403784441483 ) ) ;
#4796=ADVANCED_FACE ( 'NONE', ( #3453 ), #1304, .F. ) ;
#4798=LINE ( 'NONE', #3810, #4477 ) ;
#4799=( BOUNDED_CURVE ( )  B_SPLINE_CURVE ( 2, ( #10792, #8294, #584, #4791, #8251, #4013, #3859, #2396, #4893 ),
 .UNSPECIFIED., .F., .T. ) 
 B_SPLINE_CURVE_WITH_KNOTS ( ( 3, 2, 2, 2, 3 ),
 ( 0.6640625000000000000, 0.6666666666666666297, 0.6718750000000000000, 0.6770833333333333703, 0.6796875000000000000 ),
 .UNSPECIFIED. ) 
 CURVE ( )  GEOMETRIC_REPRESENTATION_ITEM ( )  RATIONAL_B_SPLINE_CURVE ( ( 0.9330127018922194093, 0.9330127018922194093, 1.000000000000000000, 0.8660254037844387076, 1.000000000000000000, 0.8660254037844387076, 1.000000000000000000, 0.9330127018922194093, 0.9330127018922194093 ) ) 
 REPRESENTATION_ITEM ( '' )  );
#4800=EDGE_CURVE ( 'NONE', #947, #2754, #5704, .T. ) ;
#4801=CARTESIAN_POINT ( 'NONE',  ( -62.43234176562498305, 13.66145833299193413, 0.7511620957034662593 ) ) ;
#4802=CARTESIAN_POINT ( 'NONE',  ( -61.13531646874998415, 10.32812499965860198, 1.500000000000002220 ) ) ;
#4803=CARTESIAN_POINT ( 'NONE',  ( -62.26794919243111082, 10.54241454900183506, 0.4999999999999982792 ) ) ;
#4805=CARTESIAN_POINT ( 'NONE',  ( -62.99999999999998579, 13.85416666666666785, 0.9226497308103756012 ) ) ;
#4807=CARTESIAN_POINT ( 'NONE',  ( -62.99999999999998579, 11.84374999931720218, 1.500000000000001998 ) ) ;
#4809=CARTESIAN_POINT ( 'NONE',  ( -61.56765823437498142, 12.61979166632526805, 0.7511620957034663704 ) ) ;
#4810=DIRECTION ( 'NONE',  ( 0.000000000000000000, 0.000000000000000000, -1.000000000000000000 ) ) ;
#4812=EDGE_CURVE ( 'NONE', #3446, #607, #1183, .T. ) ;
#4813=CARTESIAN_POINT ( 'NONE',  ( -62.86468353124998742, 12.03645833299193413, 1.999225269531025972 ) ) ;
#4816=CARTESIAN_POINT ( 'NONE',  ( -61.13531646874998415, 15.64062499965860198, 1.500000000000002220 ) ) ;
#4820=CARTESIAN_POINT ( 'NONE',  ( -62.99999999999998579, 9.843749999317202182, 1.500000000000001998 ) ) ;
#4821=CARTESIAN_POINT ( 'NONE',  ( -62.49999999999998579, 9.666666666666667851, 2.366025403784441483 ) ) ;
#4823=CARTESIAN_POINT ( 'NONE',  ( -61.13531646874998415, 8.140624999658601979, 1.500000000000002220 ) ) ;
#4824=CARTESIAN_POINT ( 'NONE',  ( -62.26794919243111082, 14.89508544963257286, 2.500000000000003109 ) ) ;
#4828=CARTESIAN_POINT ( 'NONE',  ( -61.13531646874998415, 11.66145833299193590, 1.000774730468978468 ) ) ;
#4829=CARTESIAN_POINT ( 'NONE',  ( -62.99999999999998579, 10.64583333333333570, 2.077350269189627952 ) ) ;
#4830=EDGE_LOOP ( 'NONE', ( #376, #10531, #10716, #5166 ) ) ;
#4831=CARTESIAN_POINT ( 'NONE',  ( -61.99999999999998579, 15.31250000000000000, 0.5000000000000013323 ) ) ;
#4833=CYLINDRICAL_SURFACE ( 'NONE', #9451, 0.9999999999999981126 ) ;
#4836=CARTESIAN_POINT ( 'NONE',  ( -61.99999999999998579, 13.31249999999999822, 0.5000000000000013323 ) ) ;
#4837=CARTESIAN_POINT ( 'NONE',  ( -62.86468353124998742, 13.22395833299193235, 1.999225269531025972 ) ) ;
#4838=CARTESIAN_POINT ( 'NONE',  ( -61.56765823437498852, 10.53645833299193413, 2.248837904296538515 ) ) ;
#4839=CARTESIAN_POINT ( 'NONE',  ( -62.99999999999998579, 8.322916665983870033, 0.9226497308103756012 ) ) ;
#4840=CARTESIAN_POINT ( 'NONE',  ( -61.99999999999999289, 11.95312499965860198, 0.5015494609379544944 ) ) ;
#4841=CARTESIAN_POINT ( 'NONE',  ( -61.13531646874998415, 15.36979166632526983, 1.999225269531026417 ) ) ;
#4843=CARTESIAN_POINT ( 'NONE',  ( -61.99999999999998579, 26.00000000000000355, 1.500000000000002220 ) ) ;
#4844=CARTESIAN_POINT ( 'NONE',  ( -60.99999999999998579, 16.21874999931720396, 1.500000000000002220 ) ) ;
#4846=VERTEX_POINT ( 'NONE', #3854 ) ;
#4849=EDGE_CURVE ( 'NONE', #1608, #5268, #10686, .T. ) ;
#4851=CARTESIAN_POINT ( 'NONE',  ( -62.86468353124999453, 14.47395833299193413, 1.999225269531025750 ) ) ;
#4852=CARTESIAN_POINT ( 'NONE',  ( -62.86468353124998742, 9.723958332991934128, 1.999225269531025972 ) ) ;
#4856=CARTESIAN_POINT ( 'NONE',  ( -62.99999999999998579, 14.35416666666666785, 0.9226497308103756012 ) ) ;
#4858=CARTESIAN_POINT ( 'NONE',  ( -61.99999999999998579, 13.28124999931720041, 0.5000000000000013323 ) ) ;
#4860=CARTESIAN_POINT ( 'NONE',  ( -60.99999999999998579, 11.44791666598387003, 2.077350269189628840 ) ) ;
#4862=( BOUNDED_CURVE ( )  B_SPLINE_CURVE ( 2, ( #1464, #8194, #10787, #4839, #9175, #1561, #4944, #8247, #9907 ),
 .UNSPECIFIED., .F., .F. ) 
 B_SPLINE_CURVE_WITH_KNOTS ( ( 3, 2, 2, 2, 3 ),
 ( 0.007812499999999973112, 0.01041666666666666609, 0.01562500000000000000, 0.02083333333333333218, 0.02343749999999996531 ),
 .UNSPECIFIED. ) 
 CURVE ( )  GEOMETRIC_REPRESENTATION_ITEM ( )  RATIONAL_B_SPLINE_CURVE ( ( 0.9330127018922194093, 0.9330127018922187432, 1.000000000000000000, 0.8660254037844387076, 1.000000000000000000, 0.8660254037844387076, 1.000000000000000000, 0.9330127018922202975, 0.9330127018922194093 ) ) 
 REPRESENTATION_ITEM ( '' )  );
#4863=CARTESIAN_POINT ( 'NONE',  ( -62.86468353124998032, 13.93229166632526805, 1.000774730468978246 ) ) ;
#4864=ORIENTED_EDGE ( 'NONE', *, *, #9058, .T. ) ;
#4865=CARTESIAN_POINT ( 'NONE',  ( -62.86468353124998742, 11.28645833299193590, 1.999225269531025972 ) ) ;
#4867=EDGE_CURVE ( 'NONE', #7493, #8372, #3076, .T. ) ;
#4868=CARTESIAN_POINT ( 'NONE',  ( -62.43234176562499016, 16.05729166632526628, 2.248837904296538071 ) ) ;
#4874=CARTESIAN_POINT ( 'NONE',  ( -61.99999999999998579, 9.562500000000000000, 0.3452994616207497591 ) ) ;
#4876=CARTESIAN_POINT ( 'NONE',  ( -61.99999999999998579, 8.562500000000000000, 0.5000000000000013323 ) ) ;
#4877=CARTESIAN_POINT ( 'NONE',  ( -61.73205080756886076, 12.19866454968462932, 2.500000000000003109 ) ) ;
#4878=DIRECTION ( 'NONE',  ( 0.000000000000000000, 0.000000000000000000, -1.000000000000000000 ) ) ;
#4879=CARTESIAN_POINT ( 'NONE',  ( -61.13531646874998415, 12.39062499965860198, 1.500000000000002220 ) ) ;
#4881=ORIENTED_EDGE ( 'NONE', *, *, #5472, .F. ) ;
#4882=CARTESIAN_POINT ( 'NONE',  ( -61.99999999999998579, 9.281249999317203958, 0.5000000000000013323 ) ) ;
#4884=DIRECTION ( 'NONE',  ( -0.000000000000000000, -1.000000000000000000, -0.000000000000000000 ) ) ;
#4885=CARTESIAN_POINT ( 'NONE',  ( -62.86468353124998742, 13.47395833299193413, 1.999225269531025972 ) ) ;
#4886=CARTESIAN_POINT ( 'NONE',  ( -62.99999999999998579, 11.85416666666666607, 0.9226497308103756012 ) ) ;
#4888=CARTESIAN_POINT ( 'NONE',  ( -61.99999999999998579, 13.06250000000000178, 0.5000000000000013323 ) ) ;
#4889=CARTESIAN_POINT ( 'NONE',  ( -61.99999999999999289, 13.07812499965860198, 2.498450539062049724 ) ) ;
#4890=CARTESIAN_POINT ( 'NONE',  ( -61.13531646874998415, 15.14062499965860020, 1.500000000000002220 ) ) ;
#4891=DIRECTION ( 'NONE',  ( -0.000000000000000000, -1.000000000000000000, -0.000000000000000000 ) ) ;
#4893=CARTESIAN_POINT ( 'NONE',  ( -61.99999999999998579, 13.65624999931720218, 2.500000000000002665 ) ) ;
#4894=CARTESIAN_POINT ( 'NONE',  ( -62.99999999999998579, 15.84374999931720218, 1.500000000000001998 ) ) ;
#4899=EDGE_CURVE ( 'NONE', #5865, #6224, #3235, .T. ) ;
#4900=CARTESIAN_POINT ( 'NONE',  ( -61.56765823437498142, 14.86979166632526805, 0.7511620957034663704 ) ) ;
#4901=CARTESIAN_POINT ( 'NONE',  ( -61.99999999999998579, 9.390624999658600203, 0.5015494609379544944 ) ) ;
#4902=CARTESIAN_POINT ( 'NONE',  ( -61.13531646874997705, 16.11979166632526628, 1.999225269531026417 ) ) ;
#4903=CARTESIAN_POINT ( 'NONE',  ( -60.99999999999998579, 14.48958333265054144, 0.9226497308103762673 ) ) ;
#4905=CARTESIAN_POINT ( 'NONE',  ( -61.49999999999998579, 13.54166666666666785, 0.6339745962155628467 ) ) ;
#4906=EDGE_CURVE ( 'NONE', #10281, #7755, #621, .T. ) ;
#4908=CARTESIAN_POINT ( 'NONE',  ( -61.99999999999998579, 11.28124999931720041, 0.3452994616207497591 ) ) ;
#4909=DIRECTION ( 'NONE',  ( 0.000000000000000000, 0.000000000000000000, -1.000000000000000000 ) ) ;
#4913=CARTESIAN_POINT ( 'NONE',  ( -62.86468353124998742, 13.97395833299193413, 1.999225269531025972 ) ) ;
#4914=CARTESIAN_POINT ( 'NONE',  ( -61.99999999999997868, 11.43750000000000000, 2.500000000000002665 ) ) ;
#4916=CARTESIAN_POINT ( 'NONE',  ( -61.13531646874998415, 11.66145833299193590, 1.000774730468978468 ) ) ;
#4917=( BOUNDED_CURVE ( )  B_SPLINE_CURVE ( 2, ( #10403, #8524, #9463, #8582, #10180, #2576, #2633, #6969, #7918 ),
 .UNSPECIFIED., .F., .T. ) 
 B_SPLINE_CURVE_WITH_KNOTS ( ( 3, 2, 2, 2, 3 ),
 ( 0.8203125000000000000, 0.8229166666666666297, 0.8281250000000000000, 0.8333333333333333703, 0.8359375000000000000 ),
 .UNSPECIFIED. ) 
 CURVE ( )  GEOMETRIC_REPRESENTATION_ITEM ( )  RATIONAL_B_SPLINE_CURVE ( ( 0.9330127018922194093, 0.9330127018922194093, 1.000000000000000000, 0.8660254037844387076, 1.000000000000000000, 0.8660254037844387076, 1.000000000000000000, 0.9330127018922194093, 0.9330127018922194093 ) ) 
 REPRESENTATION_ITEM ( '' )  );
#4918=CARTESIAN_POINT ( 'NONE',  ( -61.99999999999998579, 16.00000000000000000, 1.500000000000002220 ) ) ;
#4925=ORIENTED_EDGE ( 'NONE', *, *, #3272, .F. ) ;
#4926=CARTESIAN_POINT ( 'NONE',  ( -60.99999999999998579, 9.489583332650536107, 0.9226497308103762673 ) ) ;
#4927=CARTESIAN_POINT ( 'NONE',  ( -62.99999999999998579, 10.64583333333333570, 2.077350269189627952 ) ) ;
#4930=FACE_OUTER_BOUND ( 'NONE', #10250, .T. ) ;
#4931=CARTESIAN_POINT ( 'NONE',  ( -61.49999999999998579, 9.010416665983868256, 0.6339745962155628467 ) ) ;
#4933=CARTESIAN_POINT ( 'NONE',  ( -62.43234176562499016, 11.30729166632526805, 2.248837904296538071 ) ) ;
#4934=LINE ( 'NONE', #7343, #9625 ) ;
#4940=CARTESIAN_POINT ( 'NONE',  ( -61.56765823437498142, 13.86979166632526805, 0.7511620957034663704 ) ) ;
#4944=CARTESIAN_POINT ( 'NONE',  ( -62.49999999999998579, 8.385416665983870033, 2.366025403784441483 ) ) ;
#4945=CARTESIAN_POINT ( 'NONE',  ( -62.43234176562498305, 12.97395833299193590, 0.7511620957034662593 ) ) ;
#4946=EDGE_CURVE ( 'NONE', #10494, #2251, #8991, .T. ) ;
#4947=CARTESIAN_POINT ( 'NONE',  ( -61.99999999999998579, 14.95312499965860198, 0.5015494609379544944 ) ) ;
#4952=CARTESIAN_POINT ( 'NONE',  ( -61.13531646874998415, 8.140624999658601979, 1.500000000000002220 ) ) ;
#4953=CARTESIAN_POINT ( 'NONE',  ( -62.99999999999998579, 10.39583333333333393, 2.077350269189627952 ) ) ;
#4958=CARTESIAN_POINT ( 'NONE',  ( -61.13531646874997705, 14.34895833299193413, 1.000774730468978468 ) ) ;
#4959=CARTESIAN_POINT ( 'NONE',  ( -62.86468353124998032, 10.18229166632526805, 1.000774730468978246 ) ) ;
#4960=CARTESIAN_POINT ( 'NONE',  ( -61.13531646874997705, 15.61979166632526628, 1.999225269531026417 ) ) ;
#4963=CARTESIAN_POINT ( 'NONE',  ( -61.49999999999998579, 13.29166666666666607, 0.6339745962155628467 ) ) ;
#4964=CARTESIAN_POINT ( 'NONE',  ( -61.56765823437498852, 8.848958332991934128, 2.248837904296538515 ) ) ;
#4966=CARTESIAN_POINT ( 'NONE',  ( -61.49999999999998579, 11.92708333265053611, 2.366025403784441927 ) ) ;
#4969=CARTESIAN_POINT ( 'NONE',  ( -62.86468353124999453, 13.70312499965860198, 1.500000000000002220 ) ) ;
#4970=CARTESIAN_POINT ( 'NONE',  ( -61.49999999999998579, 11.54166666666666785, 0.6339745962155628467 ) ) ;
#4972=CARTESIAN_POINT ( 'NONE',  ( -62.43234176562498305, 12.97395833299193590, 0.7511620957034662593 ) ) ;
#4973=FACE_OUTER_BOUND ( 'NONE', #2154, .T. ) ;
#4977=( BOUNDED_CURVE ( )  B_SPLINE_CURVE ( 2, ( #5569, #10393, #8085, #2966, #7186, #8134, #2853, #10452, #3619 ),
 .UNSPECIFIED., .F., .T. ) 
 B_SPLINE_CURVE_WITH_KNOTS ( ( 3, 2, 2, 2, 3 ),
 ( 0.9609375000000000000, 0.9635416666666666297, 0.9687500000000000000, 0.9739583333333333703, 0.9765625000000000000 ),
 .UNSPECIFIED. ) 
 CURVE ( )  GEOMETRIC_REPRESENTATION_ITEM ( )  RATIONAL_B_SPLINE_CURVE ( ( 0.9330127018922194093, 0.9330127018922194093, 1.000000000000000000, 0.8660254037844387076, 1.000000000000000000, 0.8660254037844387076, 1.000000000000000000, 0.9330127018922194093, 0.9330127018922194093 ) ) 
 REPRESENTATION_ITEM ( '' )  );
#4981=CARTESIAN_POINT ( 'NONE',  ( -62.99999999999998579, 11.39583333333333393, 2.077350269189627952 ) ) ;
#4984=CARTESIAN_POINT ( 'NONE',  ( -61.13531646874998415, 13.16145833299193413, 1.000774730468978468 ) ) ;
#4989=CARTESIAN_POINT ( 'NONE',  ( -61.73205080756888208, 10.91741454900183328, 2.500000000000006661 ) ) ;
#4990=EDGE_LOOP ( 'NONE', ( #2927, #10193, #4195, #4788 ) ) ;
#4991=CARTESIAN_POINT ( 'NONE',  ( -61.99999999999998579, 15.76562499965860020, 2.498450539062049724 ) ) ;
#4996=CARTESIAN_POINT ( 'NONE',  ( -61.56765823437498142, 12.93229166632526805, 0.7511620957034663704 ) ) ;
#4997=VECTOR ( 'NONE', #3736, 1000.000000000000000 ) ;
#4998=CARTESIAN_POINT ( 'NONE',  ( -62.43234176562499016, 15.80729166632526628, 2.248837904296538071 ) ) ;
#4999=CARTESIAN_POINT ( 'NONE',  ( -61.49999999999998579, 14.95833333333333393, 2.366025403784441927 ) ) ;
#5001=CARTESIAN_POINT ( 'NONE',  ( -62.86468353124998032, 8.994791666325268054, 1.000774730468978246 ) ) ;
#5004=CARTESIAN_POINT ( 'NONE',  ( -61.99999999999998579, 11.78124999931720218, 0.5000000000000013323 ) ) ;
#5006=CIRCLE ( 'NONE', #10326, 0.9999999999999983347 ) ;
#5008=VECTOR ( 'NONE', #1259, 1000.000000000000000 ) ;
#5009=CARTESIAN_POINT ( 'NONE',  ( -62.86468353124999453, 14.45312499965860020, 1.500000000000002220 ) ) ;
#5010=CARTESIAN_POINT ( 'NONE',  ( -62.43234176562498305, 11.66145833299193590, 0.7511620957034662593 ) ) ;
#5011=CARTESIAN_POINT ( 'NONE',  ( -61.56765823437498142, 15.18229166632526805, 0.7511620957034663704 ) ) ;
#5012=CARTESIAN_POINT ( 'NONE',  ( -61.99999999999998579, 9.656249999317202182, 2.500000000000002665 ) ) ;
#5014=CARTESIAN_POINT ( 'NONE',  ( -60.99999999999998579, 13.97916666666666785, 2.077350269189628840 ) ) ;
#5015=CARTESIAN_POINT ( 'NONE',  ( -61.13531646874997705, 8.911458332991934128, 1.000774730468978468 ) ) ;
#5017=( NAMED_UNIT ( * ) PLANE_ANGLE_UNIT ( ) SI_UNIT ( $, .RADIAN. ) );
#5018=VECTOR ( 'NONE', #8795, 1000.000000000000000 ) ;
#5019=CARTESIAN_POINT ( 'NONE',  ( -62.99999999999998579, 11.61458333265053611, 2.077350269189627952 ) ) ;
#5021=CARTESIAN_POINT ( 'NONE',  ( -60.99999999999998579, 9.500000000000000000, 1.500000000000002220 ) ) ;
#5023=CARTESIAN_POINT ( 'NONE',  ( -61.99999999999998579, 13.51562499965860198, 2.498450539062049724 ) ) ;
#5024=CARTESIAN_POINT ( 'NONE',  ( -61.99999999999998579, 14.43749999999999822, 2.500000000000002665 ) ) ;
#5025=ORIENTED_EDGE ( 'NONE', *, *, #2419, .T. ) ;
#5026=CARTESIAN_POINT ( 'NONE',  ( -61.13531646874998415, 13.14062499965860198, 1.500000000000002220 ) ) ;
#5027=CARTESIAN_POINT ( 'NONE',  ( -60.99999999999998579, 11.48958333265053611, 0.9226497308103762673 ) ) ;
#5029=ORIENTED_EDGE ( 'NONE', *, *, #10336, .F. ) ;
#5030=CARTESIAN_POINT ( 'NONE',  ( -62.26794919243111082, 12.42633545031537068, 2.500000000000003109 ) ) ;
#5031=EDGE_CURVE ( 'NONE', #8575, #5931, #8274, .T. ) ;
#5033=CARTESIAN_POINT ( 'NONE',  ( -60.99999999999998579, 10.75000000000000000, 1.500000000000002220 ) ) ;
#5034=VERTEX_POINT ( 'NONE', #10892 ) ;
#5035=CARTESIAN_POINT ( 'NONE',  ( -62.86468353124999453, 8.265624999658601979, 1.500000000000002220 ) ) ;
#5038=CARTESIAN_POINT ( 'NONE',  ( -61.13531646874998415, 12.86979166632526628, 1.999225269531026417 ) ) ;
#5039=CARTESIAN_POINT ( 'NONE',  ( -60.99999999999998579, 13.27083333333333215, 0.9226497308103762673 ) ) ;
#5043=CARTESIAN_POINT ( 'NONE',  ( -61.49999999999998579, 13.17708333265053433, 2.366025403784441927 ) ) ;
#5044=CARTESIAN_POINT ( 'NONE',  ( -61.99999999999998579, 14.76562499965859843, 2.498450539062049724 ) ) ;
#5045=DIRECTION ( 'NONE',  ( 0.000000000000000000, 0.000000000000000000, -1.000000000000000000 ) ) ;
#5046=LINE ( 'NONE', #4317, #7967 ) ;
#5047=CARTESIAN_POINT ( 'NONE',  ( -61.99999999999998579, 15.18750000000000000, 2.500000000000002665 ) ) ;
#5048=CARTESIAN_POINT ( 'NONE',  ( -62.86468353124999453, 12.53645833299193413, 1.999225269531025750 ) ) ;
#5049=CARTESIAN_POINT ( 'NONE',  ( -62.86468353124998742, 15.78645833299193590, 1.999225269531025972 ) ) ;
#5050=CYLINDRICAL_SURFACE ( 'NONE', #4053, 0.9999999999999981126 ) ;
#5052=CARTESIAN_POINT ( 'NONE',  ( -61.99999999999998579, 9.453124999658600203, 0.5015494609379544944 ) ) ;
#5054=DIRECTION ( 'NONE',  ( 0.000000000000000000, 0.000000000000000000, -1.000000000000000000 ) ) ;
#5055=ORIENTED_EDGE ( 'NONE', *, *, #4052, .F. ) ;
#5059=CARTESIAN_POINT ( 'NONE',  ( -62.86468353124999453, 15.22395833299193590, 1.999225269531025750 ) ) ;
#5060=CARTESIAN_POINT ( 'NONE',  ( -61.13531646874998415, 11.59895833299193590, 1.000774730468978468 ) ) ;
#5061=EDGE_CURVE ( 'NONE', #1608, #10509, #1746, .T. ) ;
#5062=CARTESIAN_POINT ( 'NONE',  ( -62.86468353124999453, 15.53645833299193590, 1.999225269531025750 ) ) ;
#5063=CYLINDRICAL_SURFACE ( 'NONE', #10127, 2.500000000000002220 ) ;
#5064=ORIENTED_EDGE ( 'NONE', *, *, #8342, .T. ) ;
#5065=CARTESIAN_POINT ( 'NONE',  ( -61.49999999999998579, 15.20833333333333393, 2.366025403784441927 ) ) ;
#5066=CARTESIAN_POINT ( 'NONE',  ( -61.13531646874997705, 8.619791666325268054, 1.999225269531026417 ) ) ;
#5067=CARTESIAN_POINT ( 'NONE',  ( -61.99999999999998579, 12.65624999931720396, 2.654700538379254571 ) ) ;
#5069=CYLINDRICAL_SURFACE ( 'NONE', #9820, 0.9999999999999981126 ) ;
#5070=CARTESIAN_POINT ( 'NONE',  ( -61.99999999999999289, 12.14062499965860198, 0.5015494609379544944 ) ) ;
#5074=CARTESIAN_POINT ( 'NONE',  ( -62.86468353124999453, 12.76562499965860198, 1.500000000000002220 ) ) ;
#5075=DIRECTION ( 'NONE',  ( 0.000000000000000000, 0.000000000000000000, -1.000000000000000000 ) ) ;
#5076=EDGE_CURVE ( 'NONE', #2754, #947, #7775, .T. ) ;
#5078=CARTESIAN_POINT ( 'NONE',  ( -61.99999999999998579, 12.18749999999999822, 2.500000000000002665 ) ) ;
#5079=ORIENTED_EDGE ( 'NONE', *, *, #4533, .T. ) ;
#5080=LINE ( 'NONE', #9264, #4792 ) ;
#5082=ORIENTED_EDGE ( 'NONE', *, *, #703, .T. ) ;
#5083=CARTESIAN_POINT ( 'NONE',  ( -61.56765823437498852, 9.348958332991935904, 2.248837904296538515 ) ) ;
#5084=EDGE_CURVE ( 'NONE', #7919, #2018, #9494, .T. ) ;
#5085=CARTESIAN_POINT ( 'NONE',  ( -62.86468353124998032, 12.99479166632526805, 1.000774730468978246 ) ) ;
#5086=CARTESIAN_POINT ( 'NONE',  ( -62.99999999999998579, 12.11458333265053611, 2.077350269189627952 ) ) ;
#5087=VERTEX_POINT ( 'NONE', #7004 ) ;
#5093=CYLINDRICAL_SURFACE ( 'NONE', #6078, 0.9999999999999981126 ) ;
#5094=CARTESIAN_POINT ( 'NONE',  ( -61.13531646874998415, 15.82812499965860198, 1.500000000000002220 ) ) ;
#5095=CARTESIAN_POINT ( 'NONE',  ( -61.99999999999998579, 16.00000000000000000, 2.500000000000000444 ) ) ;
#5096=CARTESIAN_POINT ( 'NONE',  ( -60.99999999999998579, 12.50000000000000000, 1.500000000000002220 ) ) ;
#5097=CARTESIAN_POINT ( 'NONE',  ( -61.99999999999997868, 10.68749999999999822, 2.500000000000002665 ) ) ;
#5098=CARTESIAN_POINT ( 'NONE',  ( -62.43234176562499016, 12.80729166632526805, 2.248837904296538071 ) ) ;
#5099=CARTESIAN_POINT ( 'NONE',  ( -61.56765823437498852, 9.036458332991935904, 2.248837904296538515 ) ) ;
#5100=CYLINDRICAL_SURFACE ( 'NONE', #5111, 0.9999999999999981126 ) ;
#5101=FACE_OUTER_BOUND ( 'NONE', #3845, .T. ) ;
#5102=CARTESIAN_POINT ( 'NONE',  ( -62.86468353124998742, 8.786458332991934128, 1.999225269531025972 ) ) ;
#5106=CARTESIAN_POINT ( 'NONE',  ( -61.99999999999998579, 12.03124999931720041, 0.5000000000000013323 ) ) ;
#5108=CARTESIAN_POINT ( 'NONE',  ( -61.99999999999999289, 15.01562499965860020, 2.498450539062049724 ) ) ;
#5109=CARTESIAN_POINT ( 'NONE',  ( -61.13531646874998415, 11.07812499965860020, 1.500000000000002220 ) ) ;
#5110=CARTESIAN_POINT ( 'NONE',  ( -62.43234176562499016, 15.05729166632526805, 2.248837904296538071 ) ) ;
#5111=AXIS2_PLACEMENT_3D ( 'NONE', #942, #5896, #5 ) ;
#5114=CARTESIAN_POINT ( 'NONE',  ( -61.99999999999998579, 15.68750000000000000, 2.654700538379254571 ) ) ;
#5115=CARTESIAN_POINT ( 'NONE',  ( -61.56765823437498142, 9.182291666325268054, 0.7511620957034663704 ) ) ;
#5117=CARTESIAN_POINT ( 'NONE',  ( -60.99999999999998579, 13.21874999931720396, 1.500000000000002220 ) ) ;
#5119=ORIENTED_EDGE ( 'NONE', *, *, #5084, .F. ) ;
#5123=CARTESIAN_POINT ( 'NONE',  ( -61.13531646874998415, 11.57812499965860198, 1.500000000000002220 ) ) ;
#5125=VECTOR ( 'NONE', #8185, 1000.000000000000000 ) ;
#5127=CARTESIAN_POINT ( 'NONE',  ( -61.99999999999998579, 12.81250000000000000, 0.5000000000000013323 ) ) ;
#5128=CARTESIAN_POINT ( 'NONE',  ( -61.13531646874998415, 13.39062499965860020, 1.500000000000002220 ) ) ;
#5130=LINE ( 'NONE', #913, #9370 ) ;
#5131=CARTESIAN_POINT ( 'NONE',  ( -62.49999999999998579, 9.802083332650536107, 0.6339745962155627357 ) ) ;
#5132=ORIENTED_EDGE ( 'NONE', *, *, #9294, .F. ) ;
#5133=CARTESIAN_POINT ( 'NONE',  ( -61.99999999999998579, 13.93749999999999822, 2.500000000000002665 ) ) ;
#5134=ORIENTED_EDGE ( 'NONE', *, *, #3278, .F. ) ;
#5135=FACE_OUTER_BOUND ( 'NONE', #1217, .T. ) ;
#5136=( BOUNDED_CURVE ( )  B_SPLINE_CURVE ( 2, ( #3312, #9313, #10138, #6872, #10246, #2654, #2539, #5030, #10088 ),
 .UNSPECIFIED., .F., .T. ) 
 B_SPLINE_CURVE_WITH_KNOTS ( ( 3, 2, 2, 2, 3 ),
 ( 0.5390625000000000000, 0.5416666666666666297, 0.5468750000000000000, 0.5520833333333333703, 0.5546875000000000000 ),
 .UNSPECIFIED. ) 
 CURVE ( )  GEOMETRIC_REPRESENTATION_ITEM ( )  RATIONAL_B_SPLINE_CURVE ( ( 0.9330127018922194093, 0.9330127018922194093, 1.000000000000000000, 0.8660254037844387076, 1.000000000000000000, 0.8660254037844387076, 1.000000000000000000, 0.9330127018922194093, 0.9330127018922194093 ) ) 
 REPRESENTATION_ITEM ( '' )  );
#5137=CARTESIAN_POINT ( 'NONE',  ( -61.99999999999998579, 11.51562499965860020, 2.498450539062049724 ) ) ;
#5141=CARTESIAN_POINT ( 'NONE',  ( -61.13531646874998415, 9.119791666325268054, 1.999225269531026417 ) ) ;
#5144=CARTESIAN_POINT ( 'NONE',  ( -61.56765823437498142, 12.93229166632526805, 0.7511620957034663704 ) ) ;
#5145=CARTESIAN_POINT ( 'NONE',  ( -62.26794919243111082, 12.14508544963257464, 2.500000000000003109 ) ) ;
#5146=ORIENTED_EDGE ( 'NONE', *, *, #9135, .F. ) ;
#5148=ORIENTED_EDGE ( 'NONE', *, *, #10172, .F. ) ;
#5149=CARTESIAN_POINT ( 'NONE',  ( -61.56765823437498852, 14.78645833299193413, 2.248837904296538515 ) ) ;
#5152=CARTESIAN_POINT ( 'NONE',  ( -62.49999999999998579, 12.38541666598386826, 2.366025403784441483 ) ) ;
#5153=CARTESIAN_POINT ( 'NONE',  ( -61.13531646874997705, 13.61979166632526983, 1.999225269531026417 ) ) ;
#5154=CARTESIAN_POINT ( 'NONE',  ( -61.13531646874998415, 9.328124999658600203, 1.500000000000002220 ) ) ;
#5156=CYLINDRICAL_SURFACE ( 'NONE', #1931, 0.9999999999999981126 ) ;
#5157=CARTESIAN_POINT ( 'NONE',  ( -62.86468353124998742, 9.036458332991934128, 1.999225269531025972 ) ) ;
#5158=CARTESIAN_POINT ( 'NONE',  ( -60.99999999999998579, 15.73958333265053788, 0.9226497308103762673 ) ) ;
#5162=CARTESIAN_POINT ( 'NONE',  ( -62.43234176562498305, 15.16145833299193590, 0.7511620957034662593 ) ) ;
#5163=CARTESIAN_POINT ( 'NONE',  ( -61.13531646874998415, 11.05729166632526805, 1.999225269531026417 ) ) ;
#5164=CARTESIAN_POINT ( 'NONE',  ( -61.99999999999999289, 8.640624999658601979, 0.5015494609379544944 ) ) ;
#5166=ORIENTED_EDGE ( 'NONE', *, *, #3313, .T. ) ;
#5167=CARTESIAN_POINT ( 'NONE',  ( -62.99999999999998579, 14.89583333333333570, 2.077350269189627952 ) ) ;
#5168=CARTESIAN_POINT ( 'NONE',  ( -61.13531646874997705, 8.869791666325268054, 1.999225269531026417 ) ) ;
#5170=CARTESIAN_POINT ( 'NONE',  ( -62.49999999999998579, 12.63541666598386826, 2.366025403784441483 ) ) ;
#5171=CARTESIAN_POINT ( 'NONE',  ( -61.99999999999998579, 13.06250000000000178, 0.5000000000000013323 ) ) ;
#5172=VECTOR ( 'NONE', #1343, 1000.000000000000000 ) ;
#5173=CARTESIAN_POINT ( 'NONE',  ( -62.26794919243111082, 11.67633545031536890, 2.500000000000003109 ) ) ;
#5174=CARTESIAN_POINT ( 'NONE',  ( -61.13531646874997705, 11.34895833299193413, 1.000774730468978468 ) ) ;
#5180=EDGE_CURVE ( 'NONE', #8943, #9934, #5046, .T. ) ;
#5181=CARTESIAN_POINT ( 'NONE',  ( -62.43234176562499016, 13.05729166632526805, 2.248837904296538071 ) ) ;
#5183=DIRECTION ( 'NONE',  ( -0.000000000000000000, -1.000000000000000000, -0.000000000000000000 ) ) ;
#5184=CARTESIAN_POINT ( 'NONE',  ( -62.49999999999998579, 9.552083332650536107, 0.6339745962155627357 ) ) ;
#5185=ORIENTED_EDGE ( 'NONE', *, *, #9918, .F. ) ;
#5187=CARTESIAN_POINT ( 'NONE',  ( -61.99999999999998579, 13.43749999999999822, 2.500000000000002665 ) ) ;
#5191=CARTESIAN_POINT ( 'NONE',  ( -61.99999999999998579, 11.89062499965860198, 0.5015494609379544944 ) ) ;
#5193=CARTESIAN_POINT ( 'NONE',  ( 0.000000000000000000, 0.000000000000000000, 0.000000000000000000 ) ) ;
#5195=EDGE_CURVE ( 'NONE', #5268, #4846, #8623, .T. ) ;
#5196=CARTESIAN_POINT ( 'NONE',  ( -62.86468353124999453, 9.015624999658601979, 1.500000000000002220 ) ) ;
#5197=CARTESIAN_POINT ( 'NONE',  ( -62.49999999999998579, 13.80208333265053611, 0.6339745962155627357 ) ) ;
#5199=CARTESIAN_POINT ( 'NONE',  ( -62.43234176562498305, 12.72395833299193413, 0.7511620957034662593 ) ) ;
#5202=( BOUNDED_CURVE ( )  B_SPLINE_CURVE ( 2, ( #2496, #6831, #10202, #10375, #7169, #8895, #9604, #8657, #2835 ),
 .UNSPECIFIED., .F., .T. ) 
 B_SPLINE_CURVE_WITH_KNOTS ( ( 3, 2, 2, 2, 3 ),
 ( 0.1640624999999999722, 0.1666666666666666574, 0.1718750000000000000, 0.1770833333333333426, 0.1796875000000000000 ),
 .UNSPECIFIED. ) 
 CURVE ( )  GEOMETRIC_REPRESENTATION_ITEM ( )  RATIONAL_B_SPLINE_CURVE ( ( 0.9330127018922194093, 0.9330127018922186322, 1.000000000000000000, 0.8660254037844387076, 1.000000000000000000, 0.8660254037844387076, 1.000000000000000000, 0.9330127018922194093, 0.9330127018922194093 ) ) 
 REPRESENTATION_ITEM ( '' )  );
#5205=CARTESIAN_POINT ( 'NONE',  ( -62.99999999999998579, 11.59374999931720218, 1.500000000000001998 ) ) ;
#5206=CARTESIAN_POINT ( 'NONE',  ( -61.13531646874998415, 15.05729166632526805, 1.999225269531026417 ) ) ;
#5207=FACE_OUTER_BOUND ( 'NONE', #6819, .T. ) ;
#5210=CARTESIAN_POINT ( 'NONE',  ( -62.86468353124999453, 13.76562499965860198, 1.500000000000002220 ) ) ;
#5211=CARTESIAN_POINT ( 'NONE',  ( -62.86468353124999453, 8.203124999658601979, 1.500000000000002220 ) ) ;
#5213=CARTESIAN_POINT ( 'NONE',  ( -61.99999999999998579, 15.78124999931720041, 0.5000000000000013323 ) ) ;
#5214=CARTESIAN_POINT ( 'NONE',  ( -61.13531646874998415, 8.619791666325268054, 1.999225269531026417 ) ) ;
#5215=CARTESIAN_POINT ( 'NONE',  ( -62.99999999999998579, 14.09374999931720218, 1.500000000000001998 ) ) ;
#5217=LINE ( 'NONE', #3447, #706 ) ;
#5218=CARTESIAN_POINT ( 'NONE',  ( -62.86468353124998032, 15.93229166632526628, 1.000774730468978024 ) ) ;
#5219=CARTESIAN_POINT ( 'NONE',  ( -61.13531646874998415, 11.34895833299193413, 1.000774730468978468 ) ) ;
#5220=CARTESIAN_POINT ( 'NONE',  ( -62.86468353124998032, 8.682291666325268054, 1.000774730468978024 ) ) ;
#5221=CARTESIAN_POINT ( 'NONE',  ( -62.99999999999998579, 13.07291666598386826, 0.9226497308103756012 ) ) ;
#5222=VERTEX_POINT ( 'NONE', #3490 ) ;
#5223=CARTESIAN_POINT ( 'NONE',  ( -62.49999999999998579, 14.91666666666666607, 2.366025403784441483 ) ) ;
#5224=CARTESIAN_POINT ( 'NONE',  ( -61.13531646874997705, 10.36979166632526983, 1.999225269531026417 ) ) ;
#5226=CARTESIAN_POINT ( 'NONE',  ( -62.99999999999998579, 13.32291666598386826, 0.9226497308103756012 ) ) ;
#5231=CARTESIAN_POINT ( 'NONE',  ( -61.99999999999999289, 11.39062499965859843, 0.5015494609379544944 ) ) ;
#5235=ORIENTED_EDGE ( 'NONE', *, *, #9211, .T. ) ;
#5236=CARTESIAN_POINT ( 'NONE',  ( -61.49999999999998579, 10.95833333333333393, 2.366025403784441927 ) ) ;
#5238=CARTESIAN_POINT ( 'NONE',  ( -62.86468353124998032, 13.74479166632526805, 1.000774730468978246 ) ) ;
#5241=CARTESIAN_POINT ( 'NONE',  ( -61.49999999999998579, 8.760416665983868256, 0.6339745962155628467 ) ) ;
#5245=CARTESIAN_POINT ( 'NONE',  ( -62.43234176562498305, 11.66145833299193590, 0.7511620957034662593 ) ) ;
#5248=CARTESIAN_POINT ( 'NONE',  ( -61.56765823437498142, 9.182291666325268054, 0.7511620957034663704 ) ) ;
#5251=CARTESIAN_POINT ( 'NONE',  ( -62.86468353124998742, 14.28645833299193413, 1.999225269531025972 ) ) ;
#5252=CARTESIAN_POINT ( 'NONE',  ( -61.99999999999998579, 12.15624999931720041, 2.500000000000002665 ) ) ;
#5253=VERTEX_POINT ( 'NONE', #8839 ) ;
#5258=CARTESIAN_POINT ( 'NONE',  ( -61.49999999999998579, 8.208333333333333925, 2.366025403784441927 ) ) ;
#5259=DIRECTION ( 'NONE',  ( 0.000000000000000000, 0.000000000000000000, -1.000000000000000000 ) ) ;
#5262=CARTESIAN_POINT ( 'NONE',  ( -62.86468353124999453, 13.78645833299193413, 1.999225269531025750 ) ) ;
#5263=CARTESIAN_POINT ( 'NONE',  ( -61.13531646874998415, 8.848958332991935904, 1.000774730468978468 ) ) ;
#5264=CARTESIAN_POINT ( 'NONE',  ( -60.99999999999998579, 9.250000000000000000, 1.500000000000002220 ) ) ;
#5266=CARTESIAN_POINT ( 'NONE',  ( -61.13531646874998415, 9.869791666325269830, 1.999225269531026417 ) ) ;
#5268=VERTEX_POINT ( 'NONE', #7056 ) ;
#5270=CARTESIAN_POINT ( 'NONE',  ( -61.99999999999999289, 15.51562499965860198, 2.498450539062049724 ) ) ;
#5271=EDGE_CURVE ( 'NONE', #2471, #9265, #4607, .T. ) ;
#5272=CARTESIAN_POINT ( 'NONE',  ( -61.99999999999998579, 12.01562499965860020, 2.498450539062049724 ) ) ;
#5274=CARTESIAN_POINT ( 'NONE',  ( -62.86468353124999453, 8.953124999658601979, 1.500000000000002220 ) ) ;
#5276=ORIENTED_EDGE ( 'NONE', *, *, #7407, .T. ) ;
#5277=CARTESIAN_POINT ( 'NONE',  ( -61.49999999999998579, 15.54166666666666607, 0.6339745962155628467 ) ) ;
#5278=CARTESIAN_POINT ( 'NONE',  ( -61.13531646874997705, 9.911458332991934128, 1.000774730468978468 ) ) ;
#5279=AXIS2_PLACEMENT_3D ( 'NONE', #8717, #8653, #8830 ) ;
#5281=CARTESIAN_POINT ( 'NONE',  ( -61.13531646874998415, 15.57812499965860198, 1.500000000000002220 ) ) ;
#5282=CARTESIAN_POINT ( 'NONE',  ( -60.99999999999998579, 13.48958333265053611, 0.9226497308103762673 ) ) ;
#5285=CARTESIAN_POINT ( 'NONE',  ( -60.99999999999998579, 9.770833333333332149, 0.9226497308103762673 ) ) ;
#5288=CARTESIAN_POINT ( 'NONE',  ( -62.43234176562498305, 11.16145833299193590, 0.7511620957034662593 ) ) ;
#5290=DIRECTION ( 'NONE',  ( 0.000000000000000000, 0.000000000000000000, -1.000000000000000000 ) ) ;
#5292=CARTESIAN_POINT ( 'NONE',  ( -60.99999999999998579, 11.22916666666666785, 2.077350269189628840 ) ) ;
#5293=CARTESIAN_POINT ( 'NONE',  ( -62.99999999999998579, 10.12500000000000000, 1.500000000000001998 ) ) ;
#5295=CARTESIAN_POINT ( 'NONE',  ( -61.99999999999998579, 14.32812499965860020, 2.498450539062049724 ) ) ;
#5297=CARTESIAN_POINT ( 'NONE',  ( -61.49999999999998579, 9.760416665983870033, 0.6339745962155628467 ) ) ;
#5301=CARTESIAN_POINT ( 'NONE',  ( -62.99999999999998579, 13.37500000000000000, 1.500000000000001998 ) ) ;
#5303=CARTESIAN_POINT ( 'NONE',  ( -61.99999999999998579, 10.76562499965860020, 2.498450539062049724 ) ) ;
#5305=VERTEX_POINT ( 'NONE', #395 ) ;
#5306=CARTESIAN_POINT ( 'NONE',  ( -61.56765823437498852, 10.34895833299193413, 2.248837904296538515 ) ) ;
#5309=CARTESIAN_POINT ( 'NONE',  ( -61.56765823437498142, 14.68229166632526805, 0.7511620957034663704 ) ) ;
#5311=VERTEX_POINT ( 'NONE', #8900 ) ;
#5315=CARTESIAN_POINT ( 'NONE',  ( -60.99999999999998579, 8.229166666666667851, 2.077350269189628840 ) ) ;
#5318=CARTESIAN_POINT ( 'NONE',  ( -61.13531646874997705, 14.66145833299193413, 1.000774730468978468 ) ) ;
#5319=CARTESIAN_POINT ( 'NONE',  ( -62.43234176562498305, 9.161458332991935904, 0.7511620957034662593 ) ) ;
#5321=CARTESIAN_POINT ( 'NONE',  ( -61.99999999999998579, 10.78124999931720218, 0.5000000000000013323 ) ) ;
#5323=CARTESIAN_POINT ( 'NONE',  ( -61.99999999999998579, 10.70312499965860198, 0.5015494609379544944 ) ) ;
#5326=CARTESIAN_POINT ( 'NONE',  ( -62.99999999999998579, 14.39583333333333215, 2.077350269189627952 ) ) ;
#5327=CARTESIAN_POINT ( 'NONE',  ( -61.73205080756886076, 13.02008544963257108, 0.5000000000000014433 ) ) ;
#5329=CARTESIAN_POINT ( 'NONE',  ( -61.56765823437498142, 12.61979166632526805, 0.7511620957034663704 ) ) ;
#5330=CARTESIAN_POINT ( 'NONE',  ( -62.43234176562499016, 8.994791666325268054, 2.248837904296538071 ) ) ;
#5332=( BOUNDED_CURVE ( )  B_SPLINE_CURVE ( 2, ( #804, #8421, #7280, #9252, #5021, #3200, #6603, #5752, #9147 ),
 .UNSPECIFIED., .F., .T. ) 
 B_SPLINE_CURVE_WITH_KNOTS ( ( 3, 2, 2, 2, 3 ),
 ( 0.1796875000000000000, 0.1822916666666666574, 0.1875000000000000000, 0.1927083333333333426, 0.1953124999999999722 ),
 .UNSPECIFIED. ) 
 CURVE ( )  GEOMETRIC_REPRESENTATION_ITEM ( )  RATIONAL_B_SPLINE_CURVE ( ( 0.9330127018922194093, 0.9330127018922194093, 1.000000000000000000, 0.8660254037844387076, 1.000000000000000000, 0.8660254037844387076, 1.000000000000000000, 0.9330127018922200755, 0.9330127018922194093 ) ) 
 REPRESENTATION_ITEM ( '' )  );
#5333=ORIENTED_EDGE ( 'NONE', *, *, #963, .F. ) ;
#5334=LINE ( 'NONE', #6419, #139 ) ;
#5336=CARTESIAN_POINT ( 'NONE',  ( -62.43234176562499016, 9.807291666325268054, 2.248837904296538071 ) ) ;
#5338=CARTESIAN_POINT ( 'NONE',  ( -62.86468353124999453, 14.70312499965860020, 1.500000000000002220 ) ) ;
#5339=CARTESIAN_POINT ( 'NONE',  ( -62.99999999999998579, 14.84374999931720218, 1.500000000000001998 ) ) ;
#5343=PRODUCT_DEFINITION ( 'UNKNOWN', '', #2150, #1298 ) ;
#5344=CARTESIAN_POINT ( 'NONE',  ( -61.56765823437498852, 13.53645833299193413, 2.248837904296538515 ) ) ;
#5345=CARTESIAN_POINT ( 'NONE',  ( -61.99999999999998579, 8.390624999658601979, 0.5015494609379544944 ) ) ;
#5346=CARTESIAN_POINT ( 'NONE',  ( -62.49999999999998579, 8.333333333333333925, 0.6339745962155627357 ) ) ;
#5347=ORIENTED_EDGE ( 'NONE', *, *, #9781, .T. ) ;
#5348=CARTESIAN_POINT ( 'NONE',  ( -60.99999999999998579, 12.25000000000000000, 1.500000000000002220 ) ) ;
#5349=CARTESIAN_POINT ( 'NONE',  ( -61.99999999999998579, 16.00000000000000000, 0.5000000000000041078 ) ) ;
#5350=CARTESIAN_POINT ( 'NONE',  ( -61.13531646874998415, 14.36979166632527161, 1.999225269531026417 ) ) ;
#5355=CARTESIAN_POINT ( 'NONE',  ( -62.99999999999998579, 10.36458333265053433, 2.077350269189627952 ) ) ;
#5358=CARTESIAN_POINT ( 'NONE',  ( -61.49999999999998579, 10.01041666598387003, 0.6339745962155628467 ) ) ;
#5360=CARTESIAN_POINT ( 'NONE',  ( -61.56765823437498142, 11.11979166632526805, 0.7511620957034663704 ) ) ;
#5364=CARTESIAN_POINT ( 'NONE',  ( -62.86468353124998742, 10.03645833299193235, 1.999225269531025972 ) ) ;
#5366=( BOUNDED_CURVE ( )  B_SPLINE_CURVE ( 2, ( #10199, #5981, #8488, #872, #4253, #7658, #7715, #1768, #1156 ),
 .UNSPECIFIED., .F., .F. ) 
 B_SPLINE_CURVE_WITH_KNOTS ( ( 3, 2, 2, 2, 3 ),
 ( 0.7734375000000000000, 0.7760416666666666297, 0.7812500000000000000, 0.7864583333333333703, 0.7890625000000000000 ),
 .UNSPECIFIED. ) 
 CURVE ( )  GEOMETRIC_REPRESENTATION_ITEM ( )  RATIONAL_B_SPLINE_CURVE ( ( 0.9330127018922194093, 0.9330127018922194093, 1.000000000000000000, 0.8660254037844387076, 1.000000000000000000, 0.8660254037844387076, 1.000000000000000000, 0.9330127018922194093, 0.9330127018922194093 ) ) 
 REPRESENTATION_ITEM ( '' )  );
#5368=CARTESIAN_POINT ( 'NONE',  ( -62.86468353124999453, 14.26562499965860020, 1.500000000000002220 ) ) ;
#5370=VERTEX_POINT ( 'NONE', #1346 ) ;
#5371=EDGE_CURVE ( 'NONE', #3072, #10303, #4353, .T. ) ;
#5372=CARTESIAN_POINT ( 'NONE',  ( -60.99999999999998579, 10.47916666666666607, 2.077350269189628840 ) ) ;
#5373=ORIENTED_EDGE ( 'NONE', *, *, #9615, .T. ) ;
#5375=DIRECTION ( 'NONE',  ( 0.000000000000000000, 1.000000000000000000, 0.000000000000000000 ) ) ;
#5377=CARTESIAN_POINT ( 'NONE',  ( -62.43234176562499016, 15.99479166632526628, 2.248837904296538071 ) ) ;
#5381=CARTESIAN_POINT ( 'NONE',  ( -62.86468353124999453, 14.51562499965860020, 1.500000000000002220 ) ) ;
#5382=CARTESIAN_POINT ( 'NONE',  ( -62.43234176562499016, 9.994791666325268054, 2.248837904296538071 ) ) ;
#5384=LINE ( 'NONE', #1290, #2637 ) ;
#5386=CARTESIAN_POINT ( 'NONE',  ( -61.99999999999998579, 10.95312499965860020, 0.5015494609379544944 ) ) ;
#5387=CARTESIAN_POINT ( 'NONE',  ( -62.49999999999998579, 12.16666666666666607, 2.366025403784441483 ) ) ;
#5388=VERTEX_POINT ( 'NONE', #6285 ) ;
#5390=CARTESIAN_POINT ( 'NONE',  ( -61.99999999999998579, 16.00000000000000000, 0.5000000000000041078 ) ) ;
#5391=ORIENTED_EDGE ( 'NONE', *, *, #283, .F. ) ;
#5392=CARTESIAN_POINT ( 'NONE',  ( -61.99999999999998579, 10.15624999931720041, 2.500000000000002665 ) ) ;
#5393=CARTESIAN_POINT ( 'NONE',  ( -61.56765823437498142, 13.11979166632526805, 0.7511620957034663704 ) ) ;
#5394=CARTESIAN_POINT ( 'NONE',  ( -62.86468353124998032, 9.432291666325268054, 1.000774730468978024 ) ) ;
#5396=CARTESIAN_POINT ( 'NONE',  ( -62.26794919243111082, 10.79241454900183328, 0.5000000000000013323 ) ) ;
#5397=CARTESIAN_POINT ( 'NONE',  ( -61.56765823437498142, 9.682291666325268054, 0.7511620957034663704 ) ) ;
#5399=CARTESIAN_POINT ( 'NONE',  ( -61.13531646874998415, 15.34895833299193590, 1.000774730468978468 ) ) ;
#5400=CARTESIAN_POINT ( 'NONE',  ( -62.99999999999998579, 15.07291666598386826, 0.9226497308103756012 ) ) ;
#5402=VERTEX_POINT ( 'NONE', #10382 ) ;
#5407=CARTESIAN_POINT ( 'NONE',  ( -62.86468353124999453, 12.95312499965860198, 1.500000000000002220 ) ) ;
#5408=CARTESIAN_POINT ( 'NONE',  ( -61.99999999999998579, 16.00000000000000000, 1.500000000000002220 ) ) ;
#5409=CARTESIAN_POINT ( 'NONE',  ( -62.99999999999998579, 10.61458333265053611, 2.077350269189627952 ) ) ;
#5410=ORIENTED_EDGE ( 'NONE', *, *, #7451, .F. ) ;
#5411=CARTESIAN_POINT ( 'NONE',  ( -61.99999999999998579, 12.31250000000000000, 0.3452994616207497591 ) ) ;
#5412=LINE ( 'NONE', #5349, #414 ) ;
#5413=CARTESIAN_POINT ( 'NONE',  ( -62.43234176562499016, 14.30729166632526983, 2.248837904296538071 ) ) ;
#5414=CARTESIAN_POINT ( 'NONE',  ( -60.99999999999998579, 10.27083333333333393, 0.9226497308103762673 ) ) ;
#5415=CARTESIAN_POINT ( 'NONE',  ( -61.49999999999998579, 11.01041666598386826, 0.6339745962155628467 ) ) ;
#5416=ORIENTED_EDGE ( 'NONE', *, *, #6052, .T. ) ;
#5417=CYLINDRICAL_SURFACE ( 'NONE', #10089, 0.9999999999999981126 ) ;
#5419=CARTESIAN_POINT ( 'NONE',  ( -62.86468353124998032, 12.43229166632526628, 1.000774730468978246 ) ) ;
#5421=ORIENTED_EDGE ( 'NONE', *, *, #9314, .T. ) ;
#5423=CARTESIAN_POINT ( 'NONE',  ( -62.43234176562498305, 10.22395833299193413, 0.7511620957034662593 ) ) ;
#5425=CARTESIAN_POINT ( 'NONE',  ( -61.13531646874998415, 14.66145833299193590, 1.000774730468978468 ) ) ;
#5428=CYLINDRICAL_SURFACE ( 'NONE', #3031, 0.9999999999999981126 ) ;
#5429=VERTEX_POINT ( 'NONE', #6228 ) ;
#5430=CARTESIAN_POINT ( 'NONE',  ( -61.99999999999998579, 8.687500000000000000, 2.500000000000002665 ) ) ;
#5431=CARTESIAN_POINT ( 'NONE',  ( -62.99999999999998579, 8.395833333333333925, 2.077350269189627952 ) ) ;
#5432=CARTESIAN_POINT ( 'NONE',  ( -60.99999999999998579, 11.22916666666666607, 2.077350269189628840 ) ) ;
#5434=EDGE_CURVE ( 'NONE', #10100, #5639, #3303, .T. ) ;
#5436=CARTESIAN_POINT ( 'NONE',  ( -61.56765823437498142, 14.93229166632526805, 0.7511620957034663704 ) ) ;
#5437=CARTESIAN_POINT ( 'NONE',  ( -61.13531646874998415, 10.07812499965860198, 1.500000000000002220 ) ) ;
#5438=DIRECTION ( 'NONE',  ( -0.000000000000000000, -1.000000000000000000, -0.000000000000000000 ) ) ;
#5440=CARTESIAN_POINT ( 'NONE',  ( -62.86468353124998032, 10.99479166632526628, 1.000774730468978246 ) ) ;
#5441=DIRECTION ( 'NONE',  ( -0.000000000000000000, -1.000000000000000000, -0.000000000000000000 ) ) ;
#5444=ADVANCED_FACE ( 'NONE', ( #10728 ), #8233, .T. ) ;
#5447=CARTESIAN_POINT ( 'NONE',  ( -62.86468353124999453, 12.70312499965860198, 1.500000000000002220 ) ) ;
#5448=CARTESIAN_POINT ( 'NONE',  ( -61.56765823437498142, 9.619791666325268054, 0.7511620957034663704 ) ) ;
#5450=ORIENTED_EDGE ( 'NONE', *, *, #1734, .T. ) ;
#5452=CARTESIAN_POINT ( 'NONE',  ( -61.13531646874997705, 9.619791666325268054, 1.999225269531026417 ) ) ;
#5454=SHAPE_DEFINITION_REPRESENTATION ( #4034, #6156 ) ;
#5455=CARTESIAN_POINT ( 'NONE',  ( -62.86468353124998032, 15.43229166632526805, 1.000774730468978246 ) ) ;
#5456=CARTESIAN_POINT ( 'NONE',  ( -61.99999999999998579, 14.78124999931720218, 0.3452994616207497591 ) ) ;
#5457=CARTESIAN_POINT ( 'NONE',  ( -61.49999999999998579, 14.67708333265053611, 2.366025403784441927 ) ) ;
#5461=AXIS2_PLACEMENT_3D ( 'NONE', #9283, #1617, #9330 ) ;
#5462=CARTESIAN_POINT ( 'NONE',  ( -62.86468353124998032, 12.68229166632526628, 1.000774730468978024 ) ) ;
#5463=CARTESIAN_POINT ( 'NONE',  ( -62.86468353124998032, 8.432291666325266277, 1.000774730468978246 ) ) ;
#5465=LINE ( 'NONE', #1424, #6799 ) ;
#5466=VERTEX_POINT ( 'NONE', #4099 ) ;
#5467=CARTESIAN_POINT ( 'NONE',  ( -60.99999999999998579, 13.00000000000000178, 1.500000000000002220 ) ) ;
#5468=CARTESIAN_POINT ( 'NONE',  ( -61.56765823437498142, 13.68229166632526805, 0.7511620957034663704 ) ) ;
#5469=CARTESIAN_POINT ( 'NONE',  ( -61.99999999999998579, 14.28124999931720218, 0.5000000000000013323 ) ) ;
#5471=CARTESIAN_POINT ( 'NONE',  ( -61.49999999999998579, 10.42708333265053611, 2.366025403784441927 ) ) ;
#5472=EDGE_CURVE ( 'NONE', #1239, #10050, #7068, .T. ) ;
#5476=CARTESIAN_POINT ( 'NONE',  ( -61.56765823437498852, 12.78645833299193413, 2.248837904296538515 ) ) ;
#5481=CARTESIAN_POINT ( 'NONE',  ( -61.56765823437498142, 10.43229166632526983, 0.7511620957034663704 ) ) ;
#5484=CARTESIAN_POINT ( 'NONE',  ( -62.43234176562498305, 14.97395833299193590, 0.7511620957034662593 ) ) ;
#5486=ORIENTED_EDGE ( 'NONE', *, *, #10039, .T. ) ;
#5488=EDGE_CURVE ( 'NONE', #7998, #5865, #6712, .T. ) ;
#5492=CARTESIAN_POINT ( 'NONE',  ( -61.99999999999998579, 10.03124999931720218, 0.5000000000000013323 ) ) ;
#5493=CARTESIAN_POINT ( 'NONE',  ( -62.99999999999998579, 8.125000000000000000, 1.500000000000001998 ) ) ;
#5495=CARTESIAN_POINT ( 'NONE',  ( -61.73205080756886076, 11.30133545031536890, 0.5000000000000014433 ) ) ;
#5498=CARTESIAN_POINT ( 'NONE',  ( -61.13531646874998415, 9.598958332991934128, 1.000774730468978468 ) ) ;
#5500=DIRECTION ( 'NONE',  ( -0.000000000000000000, -1.000000000000000000, -0.000000000000000000 ) ) ;
#5501=FACE_OUTER_BOUND ( 'NONE', #10256, .T. ) ;
#5502=CARTESIAN_POINT ( 'NONE',  ( -62.43234176562499016, 10.55729166632526983, 2.248837904296538071 ) ) ;
#5505=CARTESIAN_POINT ( 'NONE',  ( -60.99999999999998579, 13.94791666598387003, 2.077350269189628840 ) ) ;
#5506=LINE ( 'NONE', #5390, #5018 ) ;
#5507=( BOUNDED_CURVE ( )  B_SPLINE_CURVE ( 2, ( #3616, #4619, #9564, #7128, #10510, #5326, #2071, #8019, #3793 ),
 .UNSPECIFIED., .F., .T. ) 
 B_SPLINE_CURVE_WITH_KNOTS ( ( 3, 2, 2, 2, 3 ),
 ( 0.7890625000000000000, 0.7916666666666666297, 0.7968750000000000000, 0.8020833333333333703, 0.8046875000000000000 ),
 .UNSPECIFIED. ) 
 CURVE ( )  GEOMETRIC_REPRESENTATION_ITEM ( )  RATIONAL_B_SPLINE_CURVE ( ( 0.9330127018922194093, 0.9330127018922194093, 1.000000000000000000, 0.8660254037844387076, 1.000000000000000000, 0.8660254037844387076, 1.000000000000000000, 0.9330127018922194093, 0.9330127018922194093 ) ) 
 REPRESENTATION_ITEM ( '' )  );
#5509=CARTESIAN_POINT ( 'NONE',  ( -61.49999999999998579, 10.17708333265053611, 2.366025403784441927 ) ) ;
#5510=CARTESIAN_POINT ( 'NONE',  ( -62.86468353124998032, 12.68229166632526983, 1.000774730468978246 ) ) ;
#5512=CARTESIAN_POINT ( 'NONE',  ( -61.13531646874997705, 9.557291666325269830, 1.999225269531026417 ) ) ;
#5514=ORIENTED_EDGE ( 'NONE', *, *, #8885, .F. ) ;
#5515=CARTESIAN_POINT ( 'NONE',  ( -62.99999999999998579, 15.85416666666666430, 0.9226497308103756012 ) ) ;
#5516=CARTESIAN_POINT ( 'NONE',  ( -62.43234176562498305, 11.47395833299193590, 0.7511620957034662593 ) ) ;
#5517=CARTESIAN_POINT ( 'NONE',  ( -62.43234176562499016, 15.24479166632526805, 2.248837904296538071 ) ) ;
#5518=CARTESIAN_POINT ( 'NONE',  ( -62.49999999999998579, 14.63541666598387003, 2.366025403784441483 ) ) ;
#5521=CARTESIAN_POINT ( 'NONE',  ( -61.99999999999998579, 16.03124999931720041, 0.5000000000000013323 ) ) ;
#5522=VERTEX_POINT ( 'NONE', #2331 ) ;
#5523=CARTESIAN_POINT ( 'NONE',  ( -61.13531646874997705, 12.80729166632526983, 1.999225269531026417 ) ) ;
#5524=CARTESIAN_POINT ( 'NONE',  ( -62.43234176562498305, 8.411458332991934128, 0.7511620957034662593 ) ) ;
#5525=CARTESIAN_POINT ( 'NONE',  ( -62.99999999999998579, 10.57291666598387181, 0.9226497308103756012 ) ) ;
#5526=VERTEX_POINT ( 'NONE', #3945 ) ;
#5527=CARTESIAN_POINT ( 'NONE',  ( -61.99999999999998579, 12.06250000000000000, 0.3452994616207497591 ) ) ;
#5528=EDGE_CURVE ( 'NONE', #2070, #1239, #6618, .T. ) ;
#5530=CARTESIAN_POINT ( 'NONE',  ( -62.26794919243111082, 13.29241454900183328, 0.5000000000000013323 ) ) ;
#5532=CARTESIAN_POINT ( 'NONE',  ( -61.99999999999998579, 10.78124999931720396, 0.3452994616207497591 ) ) ;
#5535=CARTESIAN_POINT ( 'NONE',  ( -62.49999999999998579, 13.41666666666666785, 2.366025403784441483 ) ) ;
#5536=CARTESIAN_POINT ( 'NONE',  ( -61.56765823437498142, 12.36979166632526805, 0.7511620957034663704 ) ) ;
#5538=ORIENTED_EDGE ( 'NONE', *, *, #4533, .F. ) ;
#5540=AXIS2_PLACEMENT_3D ( 'NONE', #10705, #9872, #2260 ) ;
#5541=CARTESIAN_POINT ( 'NONE',  ( -61.13531646874998415, 10.89062499965860020, 1.500000000000002220 ) ) ;
#5543=CARTESIAN_POINT ( 'NONE',  ( -62.86468353124998742, 16.03645833299193768, 1.999225269531025972 ) ) ;
#5544=CARTESIAN_POINT ( 'NONE',  ( -61.99999999999998579, 15.81250000000000000, 0.5000000000000013323 ) ) ;
#5548=ADVANCED_FACE ( 'NONE', ( #10772 ), #9842, .T. ) ;
#5551=ORIENTED_EDGE ( 'NONE', *, *, #3464, .F. ) ;
#5553=CARTESIAN_POINT ( 'NONE',  ( -62.49999999999998579, 9.333333333333333925, 0.6339745962155627357 ) ) ;
#5554=CARTESIAN_POINT ( 'NONE',  ( -61.49999999999998579, 11.20833333333333393, 2.366025403784441927 ) ) ;
#5556=CARTESIAN_POINT ( 'NONE',  ( -61.99999999999998579, 12.06250000000000000, 0.5000000000000013323 ) ) ;
#5557=DIRECTION ( 'NONE',  ( 0.000000000000000000, 0.000000000000000000, -1.000000000000000000 ) ) ;
#5559=ADVANCED_FACE ( 'NONE', ( #718 ), #10880, .T. ) ;
#5560=CARTESIAN_POINT ( 'NONE',  ( -62.86468353124998742, 10.47395833299193413, 1.999225269531025972 ) ) ;
#5561=FACE_OUTER_BOUND ( 'NONE', #2577, .T. ) ;
#5562=CARTESIAN_POINT ( 'NONE',  ( -61.13531646874998415, 11.64062499965860198, 1.500000000000002220 ) ) ;
#5563=CARTESIAN_POINT ( 'NONE',  ( -61.99999999999998579, 12.18749999999999822, 2.500000000000002665 ) ) ;
#5568=ORIENTED_EDGE ( 'NONE', *, *, #5488, .T. ) ;
#5569=CARTESIAN_POINT ( 'NONE',  ( -61.99999999999998579, 15.68749999999999645, 2.500000000000002665 ) ) ;
#5570=CARTESIAN_POINT ( 'NONE',  ( -62.86468353124999453, 13.20312499965860198, 1.500000000000002220 ) ) ;
#5571=CARTESIAN_POINT ( 'NONE',  ( -62.86468353124999453, 10.22395833299193413, 1.999225269531025750 ) ) ;
#5572=CARTESIAN_POINT ( 'NONE',  ( -62.26794919243111082, 8.676335450315370679, 2.500000000000003109 ) ) ;
#5574=CARTESIAN_POINT ( 'NONE',  ( -61.99999999999998579, 16.00000000000000000, 4.000000000000004441 ) ) ;
#5575=CARTESIAN_POINT ( 'NONE',  ( -62.43234176562499016, 11.80729166632526805, 2.248837904296538071 ) ) ;
#5578=CARTESIAN_POINT ( 'NONE',  ( -62.99999999999998579, 15.86458333265053788, 2.077350269189627952 ) ) ;
#5580=VERTEX_POINT ( 'NONE', #10670 ) ;
#5582=ORIENTED_EDGE ( 'NONE', *, *, #6990, .T. ) ;
#5583=( BOUNDED_CURVE ( )  B_SPLINE_CURVE ( 2, ( #9004, #7339, #9997, #8328, #7447, #1347, #9787, #2332, #10828 ),
 .UNSPECIFIED., .F., .F. ) 
 B_SPLINE_CURVE_WITH_KNOTS ( ( 3, 2, 2, 2, 3 ),
 ( 0.02343749999999996531, 0.02604166666666666782, 0.03125000000000000000, 0.03645833333333333565, 0.03906250000000002082 ),
 .UNSPECIFIED. ) 
 CURVE ( )  GEOMETRIC_REPRESENTATION_ITEM ( )  RATIONAL_B_SPLINE_CURVE ( ( 0.9330127018922194093, 0.9330127018922185211, 1.000000000000000000, 0.8660254037844387076, 1.000000000000000000, 0.8660254037844387076, 1.000000000000000000, 0.9330127018922187432, 0.9330127018922192983 ) ) 
 REPRESENTATION_ITEM ( '' )  );
#5584=ADVANCED_FACE ( 'NONE', ( #1446 ), #2891, .T. ) ;
#5585=CARTESIAN_POINT ( 'NONE',  ( -62.86468353124999453, 12.22395833299193413, 1.999225269531025750 ) ) ;
#5586=CARTESIAN_POINT ( 'NONE',  ( -61.13531646874998415, 9.307291666325268054, 1.999225269531026417 ) ) ;
#5587=DIRECTION ( 'NONE',  ( -0.000000000000000000, -1.000000000000000000, -0.000000000000000000 ) ) ;
#5589=CARTESIAN_POINT ( 'NONE',  ( -61.99999999999998579, 12.81250000000000000, 0.3452994616207497591 ) ) ;
#5590=CARTESIAN_POINT ( 'NONE',  ( -61.73205080756885366, 8.948664549684629321, 2.500000000000001332 ) ) ;
#5592=CARTESIAN_POINT ( 'NONE',  ( -62.99999999999998579, 10.82291666598387003, 0.9226497308103756012 ) ) ;
#5594=ADVANCED_FACE ( 'NONE', ( #3182 ), #1518, .T. ) ;
#5595=CARTESIAN_POINT ( 'NONE',  ( -61.99999999999998579, 13.26562499965860198, 2.498450539062049724 ) ) ;
#5596=CARTESIAN_POINT ( 'NONE',  ( -60.99999999999998579, 15.97916666666666607, 2.077350269189628840 ) ) ;
#5598=CARTESIAN_POINT ( 'NONE',  ( -61.56765823437498142, 11.18229166632526805, 0.7511620957034663704 ) ) ;
#5599=DIRECTION ( 'NONE',  ( -0.000000000000000000, -1.000000000000000000, -0.000000000000000000 ) ) ;
#5600=CARTESIAN_POINT ( 'NONE',  ( -62.86468353124999453, 15.76562499965860198, 1.500000000000002220 ) ) ;
#5601=ORIENTED_EDGE ( 'NONE', *, *, #2763, .T. ) ;
#5603=ORIENTED_EDGE ( 'NONE', *, *, #811, .T. ) ;
#5605=CYLINDRICAL_SURFACE ( 'NONE', #3387, 0.9999999999999981126 ) ;
#5606=CARTESIAN_POINT ( 'NONE',  ( -61.99999999999998579, 9.437500000000000000, 2.654700538379254571 ) ) ;
#5608=CARTESIAN_POINT ( 'NONE',  ( -61.99999999999998579, 15.03124999931720218, 0.5000000000000013323 ) ) ;
#5609=DIRECTION ( 'NONE',  ( 0.000000000000000000, 0.000000000000000000, -1.000000000000000000 ) ) ;
#5612=CARTESIAN_POINT ( 'NONE',  ( -62.86468353124998032, 11.99479166632526805, 1.000774730468978246 ) ) ;
#5613=EDGE_CURVE ( 'NONE', #1330, #3363, #4799, .T. ) ;
#5615=ORIENTED_EDGE ( 'NONE', *, *, #5084, .T. ) ;
#5616=CARTESIAN_POINT ( 'NONE',  ( -61.73205080756885366, 9.167414549001831503, 2.500000000000001332 ) ) ;
#5617=CARTESIAN_POINT ( 'NONE',  ( -61.49999999999998579, 15.29166666666666607, 0.6339745962155628467 ) ) ;
#5619=CARTESIAN_POINT ( 'NONE',  ( -61.73205080756886076, 13.66741454900183150, 2.500000000000003109 ) ) ;
#5620=CARTESIAN_POINT ( 'NONE',  ( -62.86468353124998742, 14.22395833299193590, 1.999225269531025972 ) ) ;
#5621=CARTESIAN_POINT ( 'NONE',  ( -61.56765823437498142, 10.36979166632526983, 0.7511620957034663704 ) ) ;
#5622=CARTESIAN_POINT ( 'NONE',  ( -62.49999999999998579, 8.166666666666667851, 2.366025403784441483 ) ) ;
#5623=ORIENTED_EDGE ( 'NONE', *, *, #388, .T. ) ;
#5624=LINE ( 'NONE', #4789, #3324 ) ;
#5625=CARTESIAN_POINT ( 'NONE',  ( -61.13531646874997705, 11.11979166632526805, 1.999225269531026417 ) ) ;
#5627=CARTESIAN_POINT ( 'NONE',  ( -62.86468353124998742, 15.97395833299193590, 1.999225269531025972 ) ) ;
#5628=CARTESIAN_POINT ( 'NONE',  ( -61.49999999999998579, 15.42708333265053611, 2.366025403784441927 ) ) ;
#5633=ORIENTED_EDGE ( 'NONE', *, *, #1384, .F. ) ;
#5634=ADVANCED_FACE ( 'NONE', ( #9181 ), #8144, .T. ) ;
#5635=CARTESIAN_POINT ( 'NONE',  ( -61.13531646874997705, 13.55729166632526805, 1.999225269531026417 ) ) ;
#5636=CARTESIAN_POINT ( 'NONE',  ( -62.86468353124998742, 9.973958332991932352, 1.999225269531025972 ) ) ;
#5639=VERTEX_POINT ( 'NONE', #6422 ) ;
#5640=CARTESIAN_POINT ( 'NONE',  ( -61.49999999999998579, 14.20833333333333393, 2.366025403784441927 ) ) ;
#5643=CARTESIAN_POINT ( 'NONE',  ( -60.99999999999998579, 12.21874999931720218, 1.500000000000002220 ) ) ;
#5644=( BOUNDED_CURVE ( )  B_SPLINE_CURVE ( 2, ( #6793, #10059, #2449, #10213, #6736, #5841, #8451, #1784, #10943 ),
 .UNSPECIFIED., .F., .T. ) 
 B_SPLINE_CURVE_WITH_KNOTS ( ( 3, 2, 2, 2, 3 ),
 ( 0.6484375000000000000, 0.6510416666666666297, 0.6562500000000000000, 0.6614583333333333703, 0.6640625000000000000 ),
 .UNSPECIFIED. ) 
 CURVE ( )  GEOMETRIC_REPRESENTATION_ITEM ( )  RATIONAL_B_SPLINE_CURVE ( ( 0.9330127018922194093, 0.9330127018922194093, 1.000000000000000000, 0.8660254037844387076, 1.000000000000000000, 0.8660254037844387076, 1.000000000000000000, 0.9330127018922194093, 0.9330127018922194093 ) ) 
 REPRESENTATION_ITEM ( '' )  );
#5647=CARTESIAN_POINT ( 'NONE',  ( -62.86468353124998742, 13.22395833299193235, 1.999225269531025972 ) ) ;
#5650=CARTESIAN_POINT ( 'NONE',  ( -62.43234176562499016, 11.05729166632526805, 2.248837904296538071 ) ) ;
#5653=CARTESIAN_POINT ( 'NONE',  ( -62.43234176562498305, 15.97395833299193590, 0.7511620957034662593 ) ) ;
#5655=DIRECTION ( 'NONE',  ( 0.000000000000000000, 0.000000000000000000, -1.000000000000000000 ) ) ;
#5657=AXIS2_PLACEMENT_3D ( 'NONE', #7487, #6032, #5075 ) ;
#5659=CARTESIAN_POINT ( 'NONE',  ( -61.99999999999997868, 8.781249999317202182, 0.5000000000000013323 ) ) ;
#5660=CARTESIAN_POINT ( 'NONE',  ( -62.49999999999998579, 10.16666666666666785, 2.366025403784441483 ) ) ;
#5661=CARTESIAN_POINT ( 'NONE',  ( -61.99999999999998579, 11.93750000000000000, 2.500000000000002665 ) ) ;
#5662=DIRECTION ( 'NONE',  ( -0.000000000000000000, -1.000000000000000000, -0.000000000000000000 ) ) ;
#5663=CARTESIAN_POINT ( 'NONE',  ( -62.26794919243111082, 14.79241454900183150, 0.5000000000000013323 ) ) ;
#5664=EDGE_CURVE ( 'NONE', #9779, #4602, #6587, .T. ) ;
#5667=CARTESIAN_POINT ( 'NONE',  ( -61.99999999999998579, 11.95312499965860198, 0.5015494609379544944 ) ) ;
#5669=CARTESIAN_POINT ( 'NONE',  ( -62.26794919243111082, 14.64508544963257464, 2.500000000000003109 ) ) ;
#5671=LINE ( 'NONE', #2235, #5125 ) ;
#5674=ORIENTED_EDGE ( 'NONE', *, *, #3929, .T. ) ;
#5675=DIRECTION ( 'NONE',  ( 0.000000000000000000, 0.000000000000000000, -1.000000000000000000 ) ) ;
#5676=CARTESIAN_POINT ( 'NONE',  ( -62.86468353124998032, 14.43229166632526805, 1.000774730468978246 ) ) ;
#5678=CARTESIAN_POINT ( 'NONE',  ( -61.99999999999999289, 9.640624999658601979, 0.5015494609379544944 ) ) ;
#5680=CARTESIAN_POINT ( 'NONE',  ( -61.73205080756886076, 14.55133545031536890, 0.5000000000000014433 ) ) ;
#5682=CARTESIAN_POINT ( 'NONE',  ( -61.56765823437498852, 11.84895833299193413, 2.248837904296538515 ) ) ;
#5683=CARTESIAN_POINT ( 'NONE',  ( -61.99999999999998579, 15.70312499965860198, 0.5015494609379544944 ) ) ;
#5686=CARTESIAN_POINT ( 'NONE',  ( -61.49999999999998579, 15.92708333265053433, 2.366025403784441927 ) ) ;
#5687=CARTESIAN_POINT ( 'NONE',  ( -62.26794919243111082, 10.32366454968463287, 0.4999999999999982792 ) ) ;
#5691=CARTESIAN_POINT ( 'NONE',  ( -61.56765823437498142, 14.61979166632526805, 0.7511620957034663704 ) ) ;
#5692=CARTESIAN_POINT ( 'NONE',  ( -61.13531646874998415, 10.07812499965860198, 1.500000000000002220 ) ) ;
#5695=CARTESIAN_POINT ( 'NONE',  ( -60.99999999999998579, 13.50000000000000000, 1.500000000000002220 ) ) ;
#5696=CARTESIAN_POINT ( 'NONE',  ( -61.49999999999998579, 9.041666666666666075, 0.6339745962155628467 ) ) ;
#5697=EDGE_CURVE ( 'NONE', #10833, #9209, #4497, .T. ) ;
#5698=CARTESIAN_POINT ( 'NONE',  ( -62.99999999999998579, 12.36458333265053611, 2.077350269189627952 ) ) ;
#5699=CARTESIAN_POINT ( 'NONE',  ( -62.86468353124999453, 14.20312499965860020, 1.500000000000002220 ) ) ;
#5701=CARTESIAN_POINT ( 'NONE',  ( -61.13531646874998415, 11.14062499965860020, 1.500000000000002220 ) ) ;
#5702=( BOUNDED_CURVE ( )  B_SPLINE_CURVE ( 2, ( #7724, #881, #5939, #51, #5205, #3435, #935, #10204, #2552 ),
 .UNSPECIFIED., .F., .T. ) 
 B_SPLINE_CURVE_WITH_KNOTS ( ( 3, 2, 2, 2, 3 ),
 ( 0.4140625000000000000, 0.4166666666666666852, 0.4218750000000000000, 0.4270833333333333148, 0.4296875000000000555 ),
 .UNSPECIFIED. ) 
 CURVE ( )  GEOMETRIC_REPRESENTATION_ITEM ( )  RATIONAL_B_SPLINE_CURVE ( ( 0.9330127018922194093, 0.9330127018922194093, 1.000000000000000000, 0.8660254037844387076, 1.000000000000000000, 0.8660254037844387076, 1.000000000000000000, 0.9330127018922178550, 0.9330127018922192983 ) ) 
 REPRESENTATION_ITEM ( '' )  );
#5703=CARTESIAN_POINT ( 'NONE',  ( -61.99999999999998579, 12.15624999931720041, 2.500000000000002665 ) ) ;
#5704=CIRCLE ( 'NONE', #6972, 2.500000000000002220 ) ;
#5705=CARTESIAN_POINT ( 'NONE',  ( -61.56765823437498852, 16.09895833299193768, 2.248837904296538515 ) ) ;
#5711=CARTESIAN_POINT ( 'NONE',  ( -62.49999999999998579, 9.916666666666667851, 2.366025403784441483 ) ) ;
#5713=CARTESIAN_POINT ( 'NONE',  ( -61.99999999999998579, 8.203124999658601979, 0.5015494609379544944 ) ) ;
#5716=CARTESIAN_POINT ( 'NONE',  ( -61.99999999999998579, 15.53124999931720041, 0.5000000000000013323 ) ) ;
#5717=AXIS2_PLACEMENT_3D ( 'NONE', #6333, #2945, #2889 ) ;
#5718=VECTOR ( 'NONE', #3778, 1000.000000000000000 ) ;
#5719=CARTESIAN_POINT ( 'NONE',  ( -61.13531646874998415, 12.36979166632526628, 1.999225269531026417 ) ) ;
#5722=CARTESIAN_POINT ( 'NONE',  ( -61.99999999999998579, 9.062500000000000000, 0.5000000000000013323 ) ) ;
#5729=CARTESIAN_POINT ( 'NONE',  ( -61.13531646874998415, 14.32812499965860020, 1.500000000000002220 ) ) ;
#5730=CARTESIAN_POINT ( 'NONE',  ( -62.26794919243111082, 11.82366454968463110, 0.5000000000000013323 ) ) ;
#5731=CARTESIAN_POINT ( 'NONE',  ( -61.73205080756886076, 14.44866454968463110, 2.500000000000003109 ) ) ;
#5733=CARTESIAN_POINT ( 'NONE',  ( -61.13531646874997705, 12.11979166632526628, 1.999225269531026417 ) ) ;
#5734=CARTESIAN_POINT ( 'NONE',  ( -61.56765823437498852, 15.59895833299193590, 2.248837904296538515 ) ) ;
#5735=DIRECTION ( 'NONE',  ( -0.000000000000000000, -1.000000000000000000, -0.000000000000000000 ) ) ;
#5736=CARTESIAN_POINT ( 'NONE',  ( -61.99999999999998579, 16.01562499965860198, 2.498450539062049724 ) ) ;
#5737=CARTESIAN_POINT ( 'NONE',  ( -62.99999999999998579, 15.82291666598386826, 0.9226497308103756012 ) ) ;
#5738=DIRECTION ( 'NONE',  ( 0.000000000000000000, 0.000000000000000000, -1.000000000000000000 ) ) ;
#5739=ORIENTED_EDGE ( 'NONE', *, *, #1348, .T. ) ;
#5741=CARTESIAN_POINT ( 'NONE',  ( -62.99999999999998579, 11.86458333265053788, 2.077350269189627952 ) ) ;
#5742=CARTESIAN_POINT ( 'NONE',  ( -61.99999999999998579, 12.43749999999999822, 2.500000000000002665 ) ) ;
#5743=CARTESIAN_POINT ( 'NONE',  ( -62.43234176562499016, 14.74479166632526805, 2.248837904296538071 ) ) ;
#5744=CARTESIAN_POINT ( 'NONE',  ( -61.99999999999998579, 10.51562499965860198, 2.498450539062049724 ) ) ;
#5745=CARTESIAN_POINT ( 'NONE',  ( -62.43234176562498305, 15.22395833299193590, 0.7511620957034662593 ) ) ;
#5746=CARTESIAN_POINT ( 'NONE',  ( -61.99999999999998579, 15.65624999931720218, 2.500000000000002665 ) ) ;
#5747=ORIENTED_EDGE ( 'NONE', *, *, #8577, .F. ) ;
#5748=CARTESIAN_POINT ( 'NONE',  ( -60.99999999999998579, 14.22916666666666785, 2.077350269189628840 ) ) ;
#5751=CARTESIAN_POINT ( 'NONE',  ( -60.99999999999998579, 12.48958333265053611, 0.9226497308103762673 ) ) ;
#5752=CARTESIAN_POINT ( 'NONE',  ( -61.73205080756885366, 9.551335450315368902, 0.5000000000000028866 ) ) ;
#5755=CARTESIAN_POINT ( 'NONE',  ( -61.13531646874998415, 14.55729166632526628, 1.999225269531026417 ) ) ;
#5756=CARTESIAN_POINT ( 'NONE',  ( -61.99999999999998579, 15.56249999999999822, 0.5000000000000013323 ) ) ;
#5757=ORIENTED_EDGE ( 'NONE', *, *, #4244, .T. ) ;
#5758=CARTESIAN_POINT ( 'NONE',  ( -61.13531646874998415, 11.16145833299193413, 1.000774730468978468 ) ) ;
#5759=CYLINDRICAL_SURFACE ( 'NONE', #4575, 0.9999999999999981126 ) ;
#5762=CARTESIAN_POINT ( 'NONE',  ( -61.99999999999998579, 11.18750000000000000, 2.500000000000002665 ) ) ;
#5763=EDGE_CURVE ( 'NONE', #5311, #5466, #3288, .T. ) ;
#5764=( BOUNDED_CURVE ( )  B_SPLINE_CURVE ( 2, ( #8283, #665, #6572, #7552, #8334, #2285, #723, #5669, #4049 ),
 .UNSPECIFIED., .F., .F. ) 
 B_SPLINE_CURVE_WITH_KNOTS ( ( 3, 2, 2, 2, 3 ),
 ( 0.7890625000000000000, 0.7916666666666666297, 0.7968750000000000000, 0.8020833333333333703, 0.8046875000000000000 ),
 .UNSPECIFIED. ) 
 CURVE ( )  GEOMETRIC_REPRESENTATION_ITEM ( )  RATIONAL_B_SPLINE_CURVE ( ( 0.9330127018922194093, 0.9330127018922194093, 1.000000000000000000, 0.8660254037844387076, 1.000000000000000000, 0.8660254037844387076, 1.000000000000000000, 0.9330127018922194093, 0.9330127018922194093 ) ) 
 REPRESENTATION_ITEM ( '' )  );
#5767=CARTESIAN_POINT ( 'NONE',  ( -61.99999999999998579, 11.43750000000000000, 2.654700538379254571 ) ) ;
#5768=CARTESIAN_POINT ( 'NONE',  ( -61.99999999999998579, 16.00000000000000000, 1.500000000000002220 ) ) ;
#5769=CARTESIAN_POINT ( 'NONE',  ( -61.49999999999998579, 12.20833333333333393, 2.366025403784441927 ) ) ;
#5770=CARTESIAN_POINT ( 'NONE',  ( -62.99999999999998579, 9.614583332650536107, 2.077350269189627952 ) ) ;
#5771=CARTESIAN_POINT ( 'NONE',  ( -61.56765823437498142, 11.68229166632526805, 0.7511620957034663704 ) ) ;
#5772=CARTESIAN_POINT ( 'NONE',  ( -62.49999999999998579, 9.052083332650536107, 0.6339745962155627357 ) ) ;
#5773=ORIENTED_EDGE ( 'NONE', *, *, #1003, .T. ) ;
#5774=CARTESIAN_POINT ( 'NONE',  ( -62.26794919243111082, 15.32366454968462932, 0.5000000000000013323 ) ) ;
#5775=ADVANCED_FACE ( 'NONE', ( #8352 ), #7515, .T. ) ;
#5776=ORIENTED_EDGE ( 'NONE', *, *, #2597, .F. ) ;
#5778=CARTESIAN_POINT ( 'NONE',  ( -62.43234176562499016, 13.24479166632526805, 2.248837904296538071 ) ) ;
#5779=CYLINDRICAL_SURFACE ( 'NONE', #6980, 0.9999999999999981126 ) ;
#5782=CARTESIAN_POINT ( 'NONE',  ( -62.86468353124998032, 12.74479166632526805, 1.000774730468978024 ) ) ;
#5783=CARTESIAN_POINT ( 'NONE',  ( -62.43234176562498305, 15.47395833299193590, 0.7511620957034662593 ) ) ;
#5786=CARTESIAN_POINT ( 'NONE',  ( -61.13531646874998415, 16.07812499965860198, 1.500000000000002220 ) ) ;
#5788=CARTESIAN_POINT ( 'NONE',  ( -61.99999999999998579, 16.03124999931720396, 0.3452994616207497591 ) ) ;
#5793=CARTESIAN_POINT ( 'NONE',  ( -61.13531646874997705, 14.09895833299193413, 1.000774730468978468 ) ) ;
#5794=CARTESIAN_POINT ( 'NONE',  ( -62.86468353124998032, 9.682291666325266277, 1.000774730468978246 ) ) ;
#5795=CARTESIAN_POINT ( 'NONE',  ( -61.13531646874998415, 15.89062499965860198, 1.500000000000002220 ) ) ;
#5796=CARTESIAN_POINT ( 'NONE',  ( -61.06765823437498852, 8.179687499487902969, 1.500000000000002220 ) ) ;
#5797=ORIENTED_EDGE ( 'NONE', *, *, #697, .F. ) ;
#5798=CARTESIAN_POINT ( 'NONE',  ( -62.99999999999998579, 13.37500000000000000, 1.500000000000001998 ) ) ;
#5799=CARTESIAN_POINT ( 'NONE',  ( -61.13531646874997705, 8.369791666325269830, 1.999225269531026417 ) ) ;
#5801=SURFACE_SIDE_STYLE ('',( #3198 ) ) ;
#5802=CARTESIAN_POINT ( 'NONE',  ( -60.99999999999998579, 11.48958333265053611, 0.9226497308103762673 ) ) ;
#5804=CARTESIAN_POINT ( 'NONE',  ( -61.56765823437498142, 13.36979166632526805, 0.7511620957034663704 ) ) ;
#5806=ORIENTED_EDGE ( 'NONE', *, *, #3546, .F. ) ;
#5808=CARTESIAN_POINT ( 'NONE',  ( -61.13531646874998415, 12.41145833299193413, 1.000774730468978468 ) ) ;
#5816=EDGE_LOOP ( 'NONE', ( #8147, #2849, #4635, #5936 ) ) ;
#5817=CARTESIAN_POINT ( 'NONE',  ( -61.49999999999998579, 15.45833333333333393, 2.366025403784441927 ) ) ;
#5818=CARTESIAN_POINT ( 'NONE',  ( -60.99999999999998579, 11.00000000000000000, 1.500000000000002220 ) ) ;
#5821=CARTESIAN_POINT ( 'NONE',  ( -62.26794919243111082, 13.79241454900183150, 0.5000000000000013323 ) ) ;
#5823=EDGE_CURVE ( 'NONE', #7075, #1330, #5644, .T. ) ;
#5825=CARTESIAN_POINT ( 'NONE',  ( -61.99999999999998579, 12.57812499965860198, 2.498450539062049724 ) ) ;
#5828=DIRECTION ( 'NONE',  ( -0.000000000000000000, -1.000000000000000000, -0.000000000000000000 ) ) ;
#5830=EDGE_LOOP ( 'NONE', ( #2087, #7032, #8242, #2564 ) ) ;
#5832=CARTESIAN_POINT ( 'NONE',  ( -61.13531646874998415, 15.57812499965860198, 1.500000000000002220 ) ) ;
#5836=DIRECTION ( 'NONE',  ( -0.000000000000000000, -1.000000000000000000, -0.000000000000000000 ) ) ;
#5837=CARTESIAN_POINT ( 'NONE',  ( -61.99999999999999289, 12.20312499965860198, 0.5015494609379544944 ) ) ;
#5838=CARTESIAN_POINT ( 'NONE',  ( -61.99999999999998579, 15.45312499965860020, 0.5015494609379544944 ) ) ;
#5840=CARTESIAN_POINT ( 'NONE',  ( -62.49999999999998579, 14.38541666598387003, 2.366025403784441483 ) ) ;
#5841=CARTESIAN_POINT ( 'NONE',  ( -60.99999999999998579, 13.48958333265053611, 0.9226497308103762673 ) ) ;
#5842=CARTESIAN_POINT ( 'NONE',  ( -62.86468353124998742, 8.536458332991934128, 1.999225269531025972 ) ) ;
#5844=ORIENTED_EDGE ( 'NONE', *, *, #8228, .T. ) ;
#5849=CARTESIAN_POINT ( 'NONE',  ( -62.86468353124999453, 14.20312499965860020, 1.500000000000002220 ) ) ;
#5850=CARTESIAN_POINT ( 'NONE',  ( -61.13531646874998415, 11.55729166632526983, 1.999225269531026417 ) ) ;
#5851=CARTESIAN_POINT ( 'NONE',  ( -62.86468353124999453, 15.03645833299193590, 1.999225269531025750 ) ) ;
#5852=FACE_OUTER_BOUND ( 'NONE', #8820, .T. ) ;
#5853=ORIENTED_EDGE ( 'NONE', *, *, #4946, .F. ) ;
#5854=CARTESIAN_POINT ( 'NONE',  ( -62.49999999999998579, 13.58333333333333215, 0.6339745962155627357 ) ) ;
#5855=CARTESIAN_POINT ( 'NONE',  ( -61.13531646874997705, 9.119791666325268054, 1.999225269531026417 ) ) ;
#5857=CARTESIAN_POINT ( 'NONE',  ( -62.49999999999998579, 12.05208333265053611, 0.6339745962155627357 ) ) ;
#5861=CARTESIAN_POINT ( 'NONE',  ( -62.43234176562499016, 13.74479166632526805, 2.248837904296538071 ) ) ;
#5862=ADVANCED_FACE ( 'NONE', ( #5101 ), #5156, .T. ) ;
#5864=( BOUNDED_CURVE ( )  B_SPLINE_CURVE ( 2, ( #3897, #5663, #1395, #7290, #2281, #4774, #9063, #4824, #620 ),
 .UNSPECIFIED., .F., .F. ) 
 B_SPLINE_CURVE_WITH_KNOTS ( ( 3, 2, 2, 2, 3 ),
 ( 0.8203125000000000000, 0.8229166666666666297, 0.8281250000000000000, 0.8333333333333333703, 0.8359375000000000000 ),
 .UNSPECIFIED. ) 
 CURVE ( )  GEOMETRIC_REPRESENTATION_ITEM ( )  RATIONAL_B_SPLINE_CURVE ( ( 0.9330127018922194093, 0.9330127018922194093, 1.000000000000000000, 0.8660254037844387076, 1.000000000000000000, 0.8660254037844387076, 1.000000000000000000, 0.9330127018922194093, 0.9330127018922194093 ) ) 
 REPRESENTATION_ITEM ( '' )  );
#5865=VERTEX_POINT ( 'NONE', #10110 ) ;
#5866=CARTESIAN_POINT ( 'NONE',  ( -61.56765823437498142, 12.43229166632526805, 0.7511620957034663704 ) ) ;
#5867=DIRECTION ( 'NONE',  ( -0.000000000000000000, -1.000000000000000000, -0.000000000000000000 ) ) ;
#5873=CARTESIAN_POINT ( 'NONE',  ( -62.99999999999998579, 11.10416666666666607, 0.9226497308103756012 ) ) ;
#5875=CARTESIAN_POINT ( 'NONE',  ( -61.56765823437498852, 9.098958332991935904, 2.248837904296538515 ) ) ;
#5878=CARTESIAN_POINT ( 'NONE',  ( -61.99999999999998579, 13.70312499965860198, 0.5015494609379544944 ) ) ;
#5879=CARTESIAN_POINT ( 'NONE',  ( -62.49999999999998579, 12.05208333265053611, 0.6339745962155627357 ) ) ;
#5880=VERTEX_POINT ( 'NONE', #835 ) ;
#5882=DIRECTION ( 'NONE',  ( -0.000000000000000000, -1.000000000000000000, -0.000000000000000000 ) ) ;
#5887=CARTESIAN_POINT ( 'NONE',  ( -61.13531646874998415, 15.80729166632526628, 1.999225269531026417 ) ) ;
#5892=CARTESIAN_POINT ( 'NONE',  ( -61.13531646874998415, 13.39062499965860020, 1.500000000000002220 ) ) ;
#5894=CARTESIAN_POINT ( 'NONE',  ( -61.56765823437498142, 8.119791666325268054, 0.7511620957034663704 ) ) ;
#5896=DIRECTION ( 'NONE',  ( -0.000000000000000000, -1.000000000000000000, -0.000000000000000000 ) ) ;
#5898=CARTESIAN_POINT ( 'NONE',  ( -61.13531646874998415, 9.411458332991934128, 1.000774730468978468 ) ) ;
#5902=CARTESIAN_POINT ( 'NONE',  ( -62.49999999999998579, 12.58333333333333393, 0.6339745962155627357 ) ) ;
#5904=CARTESIAN_POINT ( 'NONE',  ( -61.99999999999999289, 14.89062499965860020, 0.5015494609379544944 ) ) ;
#5906=CARTESIAN_POINT ( 'NONE',  ( -61.56765823437498852, 11.28645833299193590, 2.248837904296538515 ) ) ;
#5907=CARTESIAN_POINT ( 'NONE',  ( -62.43234176562499016, 15.80729166632526628, 2.248837904296538071 ) ) ;
#5909=VERTEX_POINT ( 'NONE', #7622 ) ;
#5910=CARTESIAN_POINT ( 'NONE',  ( -61.99999999999998579, 14.56249999999999822, 0.3452994616207497591 ) ) ;
#5911=CARTESIAN_POINT ( 'NONE',  ( -61.99999999999999289, 8.828124999658601979, 2.498450539062049724 ) ) ;
#5913=CARTESIAN_POINT ( 'NONE',  ( -62.99999999999998579, 13.84374999931720218, 1.500000000000001998 ) ) ;
#5914=ORIENTED_EDGE ( 'NONE', *, *, #703, .F. ) ;
#5917=CARTESIAN_POINT ( 'NONE',  ( -61.13531646874998415, 14.09895833299193413, 1.000774730468978468 ) ) ;
#5918=FACE_OUTER_BOUND ( 'NONE', #1626, .T. ) ;
#5919=EDGE_CURVE ( 'NONE', #3055, #9827, #7902, .T. ) ;
#5922=CARTESIAN_POINT ( 'NONE',  ( -62.43234176562498305, 12.47395833299193413, 0.7511620957034662593 ) ) ;
#5924=ORIENTED_EDGE ( 'NONE', *, *, #5823, .F. ) ;
#5926=CARTESIAN_POINT ( 'NONE',  ( -61.99999999999998579, 16.00000000000000000, 1.500000000000002220 ) ) ;
#5929=( BOUNDED_SURFACE ( )  B_SPLINE_SURFACE ( 1, 2, ( 
 ( #4718, #6620, #3115, #8125, #458, #3011, #1449, #1397, #513, #622, #3947, #3899, #4000, #9064, #10672, #6462, #4776, #9892, #7395, #198, #4348, #1549, #3273, #85, #6669, #1083, #5241, #4473, #2759, #3471, #10883, #3584, #10241, #1813, #2648, #2586, #7877, #1026, #4931, #3640, #3528, #6089, #7759, #7818, #10000, #720, #8330, #6033, #9475, #6984, #6867, #9417, #140, #2703, #2381, #258, #4410, #4101, #1924, #9165, #1870, #10362, #6145, #10189, #5184, #8592, #5972, #5770, #9530, #7499, #9361, #6930, #8644, #10301, #5297, #1757, #5131, #8535, #972, #8708, #915, #4296, #7706, #1267, #10590, #10415, #8987, #1329, #1983, #9821, #6205, #2989, #4699, #7266, #7932, #6323, #1203, #9706, #311, #2817, #7098, #6376, #7155, #5355, #10537, #3044, #5471, #9590, #8767, #9764, #2043, #1147, #3759, #2158, #2876, #4528, #2097, #3697, #4645, #2936, #8937, #2213, #10479, #5532, #8106, #5592, #6266, #437, #488, #3875, #9652, #8160, #8880, #10649, #5415, #6437, #8050, #1377, #4750, #548, #3821, #7037, #7209, #8819, #4584, #7990, #375, #4908, #10912, #648, #2365, #9039, #7377, #3097, #10028, #4860, #3147, #5802, #6653, #601, #751, #8308, #8210, #5019, #1430, #3251, #4027, #6493, #2410, #9981, #6544, #9199, #7482, #7533, #4807, #9929, #9875, #8418, #4966, #9145, #2261, #3984, #8265, #10756, #5857, #1582, #9251, #3302, #7426, #2315, #8367, #10808, #5643, #4136, #3928, #6698, #700, #10073, #3199, #5698, #9092, #1484, #1532, #2470, #6601, #5751, #4082, #10860, #1639, #7318, #10710, #1911, #5170, #5067, #10123, #10226, #9349, #2575, #6019, #8581, #8632, #8467, #10179, #9302, #6968, #957, #4336, #802, #852, #4179, #902, #1744, #1857, #9515, #3513, #1011, #7581, #4392, #3568, #5961, #5117, #10349, #6808, #2746, #74, #5226, #3459, #7747, #2632, #2522, #9405, #6132, #2689, #5282, #10961, #3350, #8523, #7804, #186, #6753, #7693, #4283, #23, #6074, #6916, #6856, #127, #10285, #9462, #1798, #5913, #1692, #4232, #7639, #3400, #359, #8751, #9805, #2863, #8692, #2974, #7197, #6308, #3032, #9635, #1132, #4514, #10578, #476, #10402, #9690, #243, #3628, #8806, #2029, #7917, #1188, #1311, #2801, #4630, #8922, #298, #7975, #2083, #9576, #6250, #7249, #10462, #5518, #1969, #10632, #1070, #7025, #2145, #8864, #5456, #6424, #3681, #5339, #4686, #8093, #7081, #2200, #4458, #6189, #3860, #1251, #8032, #7860, #5400, #4568, #3745, #7142, #10522, #2922, #422, #3807, #6360, #9748, #2249, #8145, #8197, #10793, #1567, #7306, #532, #5628, #9131, #3183, #9025, #1520, #6684, #9966, #9862, #3916, #4014, #3134, #7360, #6588, #2348, #2397, #1416, #3971, #3082, #736, #5737, #4894, #5578, #4793, #8975, #5686, #6531, #6638, #3289, #8295, #5788, #1366, #9183, #8353, #10745, #9913, #4121, #585, #7516, #4844 ),
 ( #4952, #10899, #7468, #10693, #10061, #682, #4066, #10847, #3231, #4735, #6480, #2302, #1470, #10015, #9079, #8253, #635, #7411, #6001, #5842, #4376, #7733, #8405, #5214, #1624, #9390, #112, #2678, #3334, #1727, #7623, #5102, #6737, #9239, #2509, #1785, #2562, #787, #5949, #9446, #889, #5001, #4166, #5157, #8452, #7567, #10164, #8564, #9288, #10944, #8507, #10111, #8, #1680, #3498, #945, #9335, #10214, #2614, #6899, #4270, #5898, #1843, #5052, #4324, #10270, #7679, #837, #3555, #3388, #2450, #6060, #8618, #61, #7789, #6794, #4217, #3444, #996, #170, #6842, #6952, #1896, #5266, #10445, #280, #6173, #2847, #2960, #1055, #6292, #10562, #10388, #9619, #7958, #228, #4499, #8906, #1117, #7180, #3613, #1293, #2732, #8672, #3789, #10506, #3730, #8077, #9560, #7010, #6344, #4441, #9728, #459, #2124, #7125, #5502, #3666, #2785, #7843, #1954, #4551, #4669, #5323, #8734, #7903, #2905, #340, #7063, #9676, #3843, #2068, #6234, #2012, #8791, #5386, #1173, #5440, #8845, #10332, #1231, #4616, #8016, #6115, #403, #9501, #7233, #7292, #10614, #7342, #8182, #8282, #4933, #9952, #4048, #3012, #10831, #10001, #1399, #4777, #2382, #2232, #9166, #6513, #664, #9893, #10775, #9065, #5562, #4828, #5771, #9114, #569, #10673, #2284, #10732, #7450, #3215, #6621, #3116, #1551, #8332, #3950, #5667, #721, #5612, #6405, #1450, #9790, #8235, #3166, #623, #8960, #4002, #2183, #1503, #7396, #3067, #6570, #2334, #1351, #4719, #8126, #5719, #4879, #6464, #515, #3900, #9846, #9006, #4254, #9375, #5934, #5825, #96, #9222, #2599, #45, #6775, #4152, #5199, #9273, #4102, #1770, #5982, #1712, #9429, #5038, #7551, #10930, #5144, #6881, #1606, #5085, #6670, #10046, #4201, #8436, #3320, #7606, #7718, #4984, #3429, #4309, #6720, #3374, #8490, #8388, #1665, #2662, #3482, #10254, #822, #8545, #6043, #10097, #7661, #929, #1826, #2493, #874, #10200, #8602, #773, #7501, #8345, #6828, #5878, #10884, #9320, #3274, #2432, #10149, #2546, #7941, #267, #1215, #6220, #7771, #2052, #1994, #8001, #8719, #10427, #6100, #4425, #155, #7110, #1937, #209, #2888, #3710, #8654, #8831, #5368, #5251, #2108, #9485, #323, #1097, #3538, #10489, #7047, #3596, #6276, #4537, #4598, #3650, #9661, #2832, #10313, #9601, #10549, #5425, #5309, #7826, #8777, #4483, #384, #3771, #7166, #7889, #6157, #6995, #2944, #6332, #1157, #9715, #5484, #981, #4358, #2716, #6938, #1882, #1037, #10372, #2770, #9542, #9990, #3054, #8892, #3155, #7384, #6501, #3206, #9831, #8947, #4708, #10764, #654, #10599, #9883, #446, #3830, #8996, #2221, #8115, #1386, #1492, #3000, #4816, #9102, #1338, #8169, #2272, #9777, #5600, #6390, #9050, #3991, #2168, #7438, #1276, #7219, #2322, #1439, #5653, #6610, #500, #5543, #4868, #3886, #5705, #2373, #8271 ) ),
 .UNSPECIFIED., .F., .F., .T. ) 
 B_SPLINE_SURFACE_WITH_KNOTS ( ( 2, 2 ),
 ( 3, 2, 2, 2, 2, 2, 2, 2, 2, 2, 2, 2, 2, 2, 2, 2, 2, 2, 2, 2, 2, 2, 2, 2, 2, 2, 2, 2, 2, 2, 2, 2, 2, 2, 2, 2, 2, 2, 2, 2, 2, 2, 2, 2, 2, 2, 2, 2, 2, 2, 2, 2, 2, 2, 2, 2, 2, 2, 2, 2, 2, 2, 2, 2, 2, 2, 2, 2, 2, 2, 2, 2, 2, 2, 2, 2, 2, 2, 2, 2, 2, 2, 2, 2, 2, 2, 2, 2, 2, 2, 2, 2, 2, 2, 2, 2, 2, 2, 2, 2, 2, 2, 2, 2, 2, 2, 2, 2, 2, 2, 2, 2, 2, 2, 2, 2, 2, 2, 2, 2, 2, 2, 2, 2, 2, 2, 2, 2, 2, 2, 2, 2, 2, 2, 2, 2, 2, 2, 2, 2, 2, 2, 2, 2, 2, 2, 2, 2, 2, 2, 2, 2, 2, 2, 2, 2, 2, 2, 2, 2, 2, 2, 2, 2, 2, 2, 2, 2, 2, 2, 2, 2, 2, 2, 2, 2, 2, 2, 2, 2, 2, 2, 2, 2, 2, 2, 2, 2, 2, 2, 2, 2, 3 ),
 ( 0.000000000000000000, 1.000000000000000000 ),
 ( 0.000000000000000000, 0.005208333333333333044, 0.01041666666666666609, 0.01562500000000000000, 0.02083333333333333218, 0.02604166666666666782, 0.03125000000000000000, 0.03645833333333333565, 0.04166666666666666435, 0.04687500000000000000, 0.05208333333333333565, 0.05729166666666666435, 0.06250000000000000000, 0.06770833333333332871, 0.07291666666666667129, 0.07812500000000000000, 0.08333333333333332871, 0.08854166666666667129, 0.09375000000000000000, 0.09895833333333332871, 0.1041666666666666713, 0.1093750000000000000, 0.1145833333333333287, 0.1197916666666666713, 0.1250000000000000000, 0.1302083333333333426, 0.1354166666666666574, 0.1406250000000000000, 0.1458333333333333426, 0.1510416666666666574, 0.1562500000000000000, 0.1614583333333333426, 0.1666666666666666574, 0.1718750000000000000, 0.1770833333333333426, 0.1822916666666666574, 0.1875000000000000000, 0.1927083333333333426, 0.1979166666666666574, 0.2031250000000000000, 0.2083333333333333426, 0.2135416666666666574, 0.2187500000000000000, 0.2239583333333333426, 0.2291666666666666574, 0.2343750000000000000, 0.2395833333333333426, 0.2447916666666666574, 0.2500000000000000000, 0.2552083333333333148, 0.2604166666666666852, 0.2656250000000000000, 0.2708333333333333148, 0.2760416666666666852, 0.2812500000000000000, 0.2864583333333333148, 0.2916666666666666852, 0.2968750000000000000, 0.3020833333333333148, 0.3072916666666666852, 0.3125000000000000000, 0.3177083333333333148, 0.3229166666666666852, 0.3281250000000000000, 0.3333333333333333148, 0.3385416666666666852, 0.3437500000000000000, 0.3489583333333333148, 0.3541666666666666852, 0.3593750000000000000, 0.3645833333333333148, 0.3697916666666666852, 0.3750000000000000000, 0.3802083333333333148, 0.3854166666666666852, 0.3906250000000000000, 0.3958333333333333148, 0.4010416666666666852, 0.4062500000000000000, 0.4114583333333333148, 0.4166666666666666852, 0.4218750000000000000, 0.4270833333333333148, 0.4322916666666666852, 0.4375000000000000000, 0.4427083333333333148, 0.4479166666666666852, 0.4531250000000000000, 0.4583333333333333148, 0.4635416666666666852, 0.4687500000000000000, 0.4739583333333333148, 0.4791666666666666852, 0.4843750000000000000, 0.4895833333333333148, 0.4947916666666666852, 0.5000000000000000000, 0.5052083333333333703, 0.5104166666666666297, 0.5156250000000000000, 0.5208333333333333703, 0.5260416666666666297, 0.5312500000000000000, 0.5364583333333333703, 0.5416666666666666297, 0.5468750000000000000, 0.5520833333333333703, 0.5572916666666666297, 0.5625000000000000000, 0.5677083333333333703, 0.5729166666666666297, 0.5781250000000000000, 0.5833333333333333703, 0.5885416666666666297, 0.5937500000000000000, 0.5989583333333333703, 0.6041666666666666297, 0.6093750000000000000, 0.6145833333333333703, 0.6197916666666666297, 0.6250000000000000000, 0.6302083333333333703, 0.6354166666666666297, 0.6406250000000000000, 0.6458333333333333703, 0.6510416666666666297, 0.6562500000000000000, 0.6614583333333333703, 0.6666666666666666297, 0.6718750000000000000, 0.6770833333333333703, 0.6822916666666666297, 0.6875000000000000000, 0.6927083333333333703, 0.6979166666666666297, 0.7031250000000000000, 0.7083333333333333703, 0.7135416666666666297, 0.7187500000000000000, 0.7239583333333333703, 0.7291666666666666297, 0.7343750000000000000, 0.7395833333333333703, 0.7447916666666666297, 0.7500000000000000000, 0.7552083333333333703, 0.7604166666666666297, 0.7656250000000000000, 0.7708333333333333703, 0.7760416666666666297, 0.7812500000000000000, 0.7864583333333333703, 0.7916666666666666297, 0.7968750000000000000, 0.8020833333333333703, 0.8072916666666666297, 0.8125000000000000000, 0.8177083333333333703, 0.8229166666666666297, 0.8281250000000000000, 0.8333333333333333703, 0.8385416666666666297, 0.8437500000000000000, 0.8489583333333333703, 0.8541666666666666297, 0.8593750000000000000, 0.8645833333333333703, 0.8697916666666666297, 0.8750000000000000000, 0.8802083333333333703, 0.8854166666666666297, 0.8906250000000000000, 0.8958333333333333703, 0.9010416666666666297, 0.9062500000000000000, 0.9114583333333333703, 0.9166666666666666297, 0.9218750000000000000, 0.9270833333333333703, 0.9322916666666666297, 0.9375000000000000000, 0.9427083333333333703, 0.9479166666666666297, 0.9531250000000000000, 0.9583333333333333703, 0.9635416666666666297, 0.9687500000000000000, 0.9739583333333333703, 0.9791666666666666297, 0.9843750000000000000, 0.9895833333333333703, 0.9947916666666666297, 1.000000000000000000 ),
 .UNSPECIFIED. ) 
 GEOMETRIC_REPRESENTATION_ITEM ( )  RATIONAL_B_SPLINE_SURFACE ( (
 ( 1.000000000000000000, 0.8660254037844387076, 1.000000000000000000, 0.8660254037844387076, 1.000000000000000000, 0.8660254037844387076, 1.000000000000000000, 0.8660254037844387076, 1.000000000000000000, 0.8660254037844387076, 1.000000000000000000, 0.8660254037844387076, 1.000000000000000000, 0.8660254037844387076, 1.000000000000000000, 0.8660254037844387076, 1.000000000000000000, 0.8660254037844387076, 1.000000000000000000, 0.8660254037844387076, 1.000000000000000000, 0.8660254037844387076, 1.000000000000000000, 0.8660254037844387076, 1.000000000000000000, 0.8660254037844387076, 1.000000000000000000, 0.8660254037844387076, 1.000000000000000000, 0.8660254037844387076, 1.000000000000000000, 0.8660254037844387076, 1.000000000000000000, 0.8660254037844387076, 1.000000000000000000, 0.8660254037844387076, 1.000000000000000000, 0.8660254037844387076, 1.000000000000000000, 0.8660254037844387076, 1.000000000000000000, 0.8660254037844387076, 1.000000000000000000, 0.8660254037844387076, 1.000000000000000000, 0.8660254037844387076, 1.000000000000000000, 0.8660254037844387076, 1.000000000000000000, 0.8660254037844387076, 1.000000000000000000, 0.8660254037844387076, 1.000000000000000000, 0.8660254037844387076, 1.000000000000000000, 0.8660254037844387076, 1.000000000000000000, 0.8660254037844387076, 1.000000000000000000, 0.8660254037844387076, 1.000000000000000000, 0.8660254037844387076, 1.000000000000000000, 0.8660254037844387076, 1.000000000000000000, 0.8660254037844387076, 1.000000000000000000, 0.8660254037844387076, 1.000000000000000000, 0.8660254037844387076, 1.000000000000000000, 0.8660254037844387076, 1.000000000000000000, 0.8660254037844387076, 1.000000000000000000, 0.8660254037844387076, 1.000000000000000000, 0.8660254037844387076, 1.000000000000000000, 0.8660254037844387076, 1.000000000000000000, 0.8660254037844387076, 1.000000000000000000, 0.8660254037844387076, 1.000000000000000000, 0.8660254037844387076, 1.000000000000000000, 0.8660254037844387076, 1.000000000000000000, 0.8660254037844387076, 1.000000000000000000, 0.8660254037844387076, 1.000000000000000000, 0.8660254037844387076, 1.000000000000000000, 0.8660254037844387076, 1.000000000000000000, 0.8660254037844387076, 1.000000000000000000, 0.8660254037844387076, 1.000000000000000000, 0.8660254037844387076, 1.000000000000000000, 0.8660254037844387076, 1.000000000000000000, 0.8660254037844387076, 1.000000000000000000, 0.8660254037844387076, 1.000000000000000000, 0.8660254037844387076, 1.000000000000000000, 0.8660254037844387076, 1.000000000000000000, 0.8660254037844387076, 1.000000000000000000, 0.8660254037844387076, 1.000000000000000000, 0.8660254037844387076, 1.000000000000000000, 0.8660254037844387076, 1.000000000000000000, 0.8660254037844387076, 1.000000000000000000, 0.8660254037844387076, 1.000000000000000000, 0.8660254037844387076, 1.000000000000000000, 0.8660254037844387076, 1.000000000000000000, 0.8660254037844387076, 1.000000000000000000, 0.8660254037844387076, 1.000000000000000000, 0.8660254037844387076, 1.000000000000000000, 0.8660254037844387076, 1.000000000000000000, 0.8660254037844387076, 1.000000000000000000, 0.8660254037844387076, 1.000000000000000000, 0.8660254037844387076, 1.000000000000000000, 0.8660254037844387076, 1.000000000000000000, 0.8660254037844387076, 1.000000000000000000, 0.8660254037844387076, 1.000000000000000000, 0.8660254037844387076, 1.000000000000000000, 0.8660254037844387076, 1.000000000000000000, 0.8660254037844387076, 1.000000000000000000, 0.8660254037844387076, 1.000000000000000000, 0.8660254037844387076, 1.000000000000000000, 0.8660254037844387076, 1.000000000000000000, 0.8660254037844387076, 1.000000000000000000, 0.8660254037844387076, 1.000000000000000000, 0.8660254037844387076, 1.000000000000000000, 0.8660254037844387076, 1.000000000000000000, 0.8660254037844387076, 1.000000000000000000, 0.8660254037844387076, 1.000000000000000000, 0.8660254037844387076, 1.000000000000000000, 0.8660254037844387076, 1.000000000000000000, 0.8660254037844387076, 1.000000000000000000, 0.8660254037844387076, 1.000000000000000000, 0.8660254037844387076, 1.000000000000000000, 0.8660254037844387076, 1.000000000000000000, 0.8660254037844387076, 1.000000000000000000, 0.8660254037844387076, 1.000000000000000000, 0.8660254037844387076, 1.000000000000000000, 0.8660254037844387076, 1.000000000000000000, 0.8660254037844387076, 1.000000000000000000, 0.8660254037844387076, 1.000000000000000000, 0.8660254037844387076, 1.000000000000000000, 0.8660254037844387076, 1.000000000000000000, 0.8660254037844387076, 1.000000000000000000, 0.8660254037844387076, 1.000000000000000000, 0.8660254037844387076, 1.000000000000000000, 0.8660254037844387076, 1.000000000000000000, 0.8660254037844387076, 1.000000000000000000, 0.8660254037844387076, 1.000000000000000000, 0.8660254037844387076, 1.000000000000000000, 0.8660254037844387076, 1.000000000000000000, 0.8660254037844387076, 1.000000000000000000, 0.8660254037844387076, 1.000000000000000000, 0.8660254037844387076, 1.000000000000000000, 0.8660254037844387076, 1.000000000000000000, 0.8660254037844387076, 1.000000000000000000, 0.8660254037844387076, 1.000000000000000000, 0.8660254037844387076, 1.000000000000000000, 0.8660254037844387076, 1.000000000000000000, 0.8660254037844387076, 1.000000000000000000, 0.8660254037844387076, 1.000000000000000000, 0.8660254037844387076, 1.000000000000000000, 0.8660254037844387076, 1.000000000000000000, 0.8660254037844387076, 1.000000000000000000, 0.8660254037844387076, 1.000000000000000000, 0.8660254037844387076, 1.000000000000000000, 0.8660254037844387076, 1.000000000000000000, 0.8660254037844387076, 1.000000000000000000, 0.8660254037844387076, 1.000000000000000000, 0.8660254037844387076, 1.000000000000000000, 0.8660254037844387076, 1.000000000000000000, 0.8660254037844387076, 1.000000000000000000, 0.8660254037844387076, 1.000000000000000000, 0.8660254037844387076, 1.000000000000000000, 0.8660254037844387076, 1.000000000000000000, 0.8660254037844387076, 1.000000000000000000, 0.8660254037844387076, 1.000000000000000000, 0.8660254037844387076, 1.000000000000000000, 0.8660254037844387076, 1.000000000000000000, 0.8660254037844387076, 1.000000000000000000, 0.8660254037844387076, 1.000000000000000000, 0.8660254037844387076, 1.000000000000000000, 0.8660254037844387076, 1.000000000000000000, 0.8660254037844387076, 1.000000000000000000, 0.8660254037844387076, 1.000000000000000000, 0.8660254037844387076, 1.000000000000000000, 0.8660254037844387076, 1.000000000000000000, 0.8660254037844387076, 1.000000000000000000, 0.8660254037844387076, 1.000000000000000000, 0.8660254037844387076, 1.000000000000000000, 0.8660254037844387076, 1.000000000000000000, 0.8660254037844387076, 1.000000000000000000, 0.8660254037844387076, 1.000000000000000000, 0.8660254037844387076, 1.000000000000000000, 0.8660254037844387076, 1.000000000000000000, 0.8660254037844387076, 1.000000000000000000, 0.8660254037844387076, 1.000000000000000000, 0.8660254037844387076, 1.000000000000000000, 0.8660254037844387076, 1.000000000000000000, 0.8660254037844387076, 1.000000000000000000, 0.8660254037844387076, 1.000000000000000000, 0.8660254037844387076, 1.000000000000000000, 0.8660254037844387076, 1.000000000000000000, 0.8660254037844387076, 1.000000000000000000, 0.8660254037844387076, 1.000000000000000000, 0.8660254037844387076, 1.000000000000000000, 0.8660254037844387076, 1.000000000000000000, 0.8660254037844387076, 1.000000000000000000, 0.8660254037844387076, 1.000000000000000000, 0.8660254037844387076, 1.000000000000000000, 0.8660254037844387076, 1.000000000000000000, 0.8660254037844387076, 1.000000000000000000, 0.8660254037844387076, 1.000000000000000000, 0.8660254037844387076, 1.000000000000000000, 0.8660254037844387076, 1.000000000000000000, 0.8660254037844387076, 1.000000000000000000, 0.8660254037844387076, 1.000000000000000000, 0.8660254037844387076, 1.000000000000000000, 0.8660254037844387076, 1.000000000000000000, 0.8660254037844387076, 1.000000000000000000, 0.8660254037844387076, 1.000000000000000000, 0.8660254037844387076, 1.000000000000000000, 0.8660254037844387076, 1.000000000000000000, 0.8660254037844387076, 1.000000000000000000, 0.8660254037844387076, 1.000000000000000000, 0.8660254037844387076, 1.000000000000000000, 0.8660254037844387076, 1.000000000000000000, 0.8660254037844387076, 1.000000000000000000, 0.8660254037844387076, 1.000000000000000000, 0.8660254037844387076, 1.000000000000000000, 0.8660254037844387076, 1.000000000000000000, 0.8660254037844387076, 1.000000000000000000, 0.8660254037844387076, 1.000000000000000000, 0.8660254037844387076, 1.000000000000000000, 0.8660254037844387076, 1.000000000000000000),
 ( 1.000000000000000000, 0.8660254037844387076, 1.000000000000000000, 0.8660254037844387076, 1.000000000000000000, 0.8660254037844387076, 1.000000000000000000, 0.8660254037844387076, 1.000000000000000000, 0.8660254037844387076, 1.000000000000000000, 0.8660254037844387076, 1.000000000000000000, 0.8660254037844387076, 1.000000000000000000, 0.8660254037844387076, 1.000000000000000000, 0.8660254037844387076, 1.000000000000000000, 0.8660254037844387076, 1.000000000000000000, 0.8660254037844387076, 1.000000000000000000, 0.8660254037844387076, 1.000000000000000000, 0.8660254037844387076, 1.000000000000000000, 0.8660254037844387076, 1.000000000000000000, 0.8660254037844387076, 1.000000000000000000, 0.8660254037844387076, 1.000000000000000000, 0.8660254037844387076, 1.000000000000000000, 0.8660254037844387076, 1.000000000000000000, 0.8660254037844387076, 1.000000000000000000, 0.8660254037844387076, 1.000000000000000000, 0.8660254037844387076, 1.000000000000000000, 0.8660254037844387076, 1.000000000000000000, 0.8660254037844387076, 1.000000000000000000, 0.8660254037844387076, 1.000000000000000000, 0.8660254037844387076, 1.000000000000000000, 0.8660254037844387076, 1.000000000000000000, 0.8660254037844387076, 1.000000000000000000, 0.8660254037844387076, 1.000000000000000000, 0.8660254037844387076, 1.000000000000000000, 0.8660254037844387076, 1.000000000000000000, 0.8660254037844387076, 1.000000000000000000, 0.8660254037844387076, 1.000000000000000000, 0.8660254037844387076, 1.000000000000000000, 0.8660254037844387076, 1.000000000000000000, 0.8660254037844387076, 1.000000000000000000, 0.8660254037844387076, 1.000000000000000000, 0.8660254037844387076, 1.000000000000000000, 0.8660254037844387076, 1.000000000000000000, 0.8660254037844387076, 1.000000000000000000, 0.8660254037844387076, 1.000000000000000000, 0.8660254037844387076, 1.000000000000000000, 0.8660254037844387076, 1.000000000000000000, 0.8660254037844387076, 1.000000000000000000, 0.8660254037844387076, 1.000000000000000000, 0.8660254037844387076, 1.000000000000000000, 0.8660254037844387076, 1.000000000000000000, 0.8660254037844387076, 1.000000000000000000, 0.8660254037844387076, 1.000000000000000000, 0.8660254037844387076, 1.000000000000000000, 0.8660254037844387076, 1.000000000000000000, 0.8660254037844387076, 1.000000000000000000, 0.8660254037844387076, 1.000000000000000000, 0.8660254037844387076, 1.000000000000000000, 0.8660254037844387076, 1.000000000000000000, 0.8660254037844387076, 1.000000000000000000, 0.8660254037844387076, 1.000000000000000000, 0.8660254037844387076, 1.000000000000000000, 0.8660254037844387076, 1.000000000000000000, 0.8660254037844387076, 1.000000000000000000, 0.8660254037844387076, 1.000000000000000000, 0.8660254037844387076, 1.000000000000000000, 0.8660254037844387076, 1.000000000000000000, 0.8660254037844387076, 1.000000000000000000, 0.8660254037844387076, 1.000000000000000000, 0.8660254037844387076, 1.000000000000000000, 0.8660254037844387076, 1.000000000000000000, 0.8660254037844387076, 1.000000000000000000, 0.8660254037844387076, 1.000000000000000000, 0.8660254037844387076, 1.000000000000000000, 0.8660254037844387076, 1.000000000000000000, 0.8660254037844387076, 1.000000000000000000, 0.8660254037844387076, 1.000000000000000000, 0.8660254037844387076, 1.000000000000000000, 0.8660254037844387076, 1.000000000000000000, 0.8660254037844387076, 1.000000000000000000, 0.8660254037844387076, 1.000000000000000000, 0.8660254037844387076, 1.000000000000000000, 0.8660254037844387076, 1.000000000000000000, 0.8660254037844387076, 1.000000000000000000, 0.8660254037844387076, 1.000000000000000000, 0.8660254037844387076, 1.000000000000000000, 0.8660254037844387076, 1.000000000000000000, 0.8660254037844387076, 1.000000000000000000, 0.8660254037844387076, 1.000000000000000000, 0.8660254037844387076, 1.000000000000000000, 0.8660254037844387076, 1.000000000000000000, 0.8660254037844387076, 1.000000000000000000, 0.8660254037844387076, 1.000000000000000000, 0.8660254037844387076, 1.000000000000000000, 0.8660254037844387076, 1.000000000000000000, 0.8660254037844387076, 1.000000000000000000, 0.8660254037844387076, 1.000000000000000000, 0.8660254037844387076, 1.000000000000000000, 0.8660254037844387076, 1.000000000000000000, 0.8660254037844387076, 1.000000000000000000, 0.8660254037844387076, 1.000000000000000000, 0.8660254037844387076, 1.000000000000000000, 0.8660254037844387076, 1.000000000000000000, 0.8660254037844387076, 1.000000000000000000, 0.8660254037844387076, 1.000000000000000000, 0.8660254037844387076, 1.000000000000000000, 0.8660254037844387076, 1.000000000000000000, 0.8660254037844387076, 1.000000000000000000, 0.8660254037844387076, 1.000000000000000000, 0.8660254037844387076, 1.000000000000000000, 0.8660254037844387076, 1.000000000000000000, 0.8660254037844387076, 1.000000000000000000, 0.8660254037844387076, 1.000000000000000000, 0.8660254037844387076, 1.000000000000000000, 0.8660254037844387076, 1.000000000000000000, 0.8660254037844387076, 1.000000000000000000, 0.8660254037844387076, 1.000000000000000000, 0.8660254037844387076, 1.000000000000000000, 0.8660254037844387076, 1.000000000000000000, 0.8660254037844387076, 1.000000000000000000, 0.8660254037844387076, 1.000000000000000000, 0.8660254037844387076, 1.000000000000000000, 0.8660254037844387076, 1.000000000000000000, 0.8660254037844387076, 1.000000000000000000, 0.8660254037844387076, 1.000000000000000000, 0.8660254037844387076, 1.000000000000000000, 0.8660254037844387076, 1.000000000000000000, 0.8660254037844387076, 1.000000000000000000, 0.8660254037844387076, 1.000000000000000000, 0.8660254037844387076, 1.000000000000000000, 0.8660254037844387076, 1.000000000000000000, 0.8660254037844387076, 1.000000000000000000, 0.8660254037844387076, 1.000000000000000000, 0.8660254037844387076, 1.000000000000000000, 0.8660254037844387076, 1.000000000000000000, 0.8660254037844387076, 1.000000000000000000, 0.8660254037844387076, 1.000000000000000000, 0.8660254037844387076, 1.000000000000000000, 0.8660254037844387076, 1.000000000000000000, 0.8660254037844387076, 1.000000000000000000, 0.8660254037844387076, 1.000000000000000000, 0.8660254037844387076, 1.000000000000000000, 0.8660254037844387076, 1.000000000000000000, 0.8660254037844387076, 1.000000000000000000, 0.8660254037844387076, 1.000000000000000000, 0.8660254037844387076, 1.000000000000000000, 0.8660254037844387076, 1.000000000000000000, 0.8660254037844387076, 1.000000000000000000, 0.8660254037844387076, 1.000000000000000000, 0.8660254037844387076, 1.000000000000000000, 0.8660254037844387076, 1.000000000000000000, 0.8660254037844387076, 1.000000000000000000, 0.8660254037844387076, 1.000000000000000000, 0.8660254037844387076, 1.000000000000000000, 0.8660254037844387076, 1.000000000000000000, 0.8660254037844387076, 1.000000000000000000, 0.8660254037844387076, 1.000000000000000000, 0.8660254037844387076, 1.000000000000000000, 0.8660254037844387076, 1.000000000000000000, 0.8660254037844387076, 1.000000000000000000, 0.8660254037844387076, 1.000000000000000000, 0.8660254037844387076, 1.000000000000000000, 0.8660254037844387076, 1.000000000000000000, 0.8660254037844387076, 1.000000000000000000, 0.8660254037844387076, 1.000000000000000000, 0.8660254037844387076, 1.000000000000000000, 0.8660254037844387076, 1.000000000000000000, 0.8660254037844387076, 1.000000000000000000, 0.8660254037844387076, 1.000000000000000000, 0.8660254037844387076, 1.000000000000000000, 0.8660254037844387076, 1.000000000000000000, 0.8660254037844387076, 1.000000000000000000, 0.8660254037844387076, 1.000000000000000000, 0.8660254037844387076, 1.000000000000000000, 0.8660254037844387076, 1.000000000000000000, 0.8660254037844387076, 1.000000000000000000, 0.8660254037844387076, 1.000000000000000000, 0.8660254037844387076, 1.000000000000000000, 0.8660254037844387076, 1.000000000000000000, 0.8660254037844387076, 1.000000000000000000, 0.8660254037844387076, 1.000000000000000000, 0.8660254037844387076, 1.000000000000000000, 0.8660254037844387076, 1.000000000000000000, 0.8660254037844387076, 1.000000000000000000, 0.8660254037844387076, 1.000000000000000000, 0.8660254037844387076, 1.000000000000000000, 0.8660254037844387076, 1.000000000000000000, 0.8660254037844387076, 1.000000000000000000, 0.8660254037844387076, 1.000000000000000000, 0.8660254037844387076, 1.000000000000000000, 0.8660254037844387076, 1.000000000000000000, 0.8660254037844387076, 1.000000000000000000, 0.8660254037844387076, 1.000000000000000000, 0.8660254037844387076, 1.000000000000000000, 0.8660254037844387076, 1.000000000000000000, 0.8660254037844387076, 1.000000000000000000, 0.8660254037844387076, 1.000000000000000000) ) ) 
 REPRESENTATION_ITEM ( '' )  SURFACE ( )  );
#5930=ORIENTED_EDGE ( 'NONE', *, *, #4471, .F. ) ;
#5931=VERTEX_POINT ( 'NONE', #2783 ) ;
#5932=CARTESIAN_POINT ( 'NONE',  ( -61.99999999999998579, 9.578124999658601979, 2.498450539062049724 ) ) ;
#5934=CARTESIAN_POINT ( 'NONE',  ( -62.43234176562499016, 12.55729166632526805, 2.248837904296538071 ) ) ;
#5935=CARTESIAN_POINT ( 'NONE',  ( -62.99999999999998579, 12.86458333265053611, 2.077350269189627952 ) ) ;
#5936=ORIENTED_EDGE ( 'NONE', *, *, #3812, .T. ) ;
#5938=ORIENTED_EDGE ( 'NONE', *, *, #6880, .F. ) ;
#5939=CARTESIAN_POINT ( 'NONE',  ( -62.49999999999998579, 11.55208333265053611, 0.6339745962155627357 ) ) ;
#5940=CARTESIAN_POINT ( 'NONE',  ( -61.13531646874998415, 15.55729166632526628, 1.999225269531026417 ) ) ;
#5944=CARTESIAN_POINT ( 'NONE',  ( -61.56765823437498142, 13.18229166632526805, 0.7511620957034663704 ) ) ;
#5945=CARTESIAN_POINT ( 'NONE',  ( -61.99999999999998579, 8.765624999658601979, 2.498450539062049724 ) ) ;
#5949=CARTESIAN_POINT ( 'NONE',  ( -61.56765823437498142, 8.932291666325268054, 0.7511620957034663704 ) ) ;
#5951=ORIENTED_EDGE ( 'NONE', *, *, #3403, .T. ) ;
#5954=CARTESIAN_POINT ( 'NONE',  ( -61.56765823437498142, 15.61979166632526628, 0.7511620957034663704 ) ) ;
#5955=CARTESIAN_POINT ( 'NONE',  ( -62.43234176562499016, 11.49479166632526805, 2.248837904296538071 ) ) ;
#5956=CARTESIAN_POINT ( 'NONE',  ( -61.13531646874998415, 15.14062499965860020, 1.500000000000002220 ) ) ;
#5957=CARTESIAN_POINT ( 'NONE',  ( -62.99999999999998579, 13.11458333265053433, 2.077350269189627952 ) ) ;
#5959=CARTESIAN_POINT ( 'NONE',  ( -62.99999999999998579, 15.60416666666666607, 0.9226497308103756012 ) ) ;
#5960=CARTESIAN_POINT ( 'NONE',  ( -62.43234176562498305, 8.973958332991934128, 0.7511620957034662593 ) ) ;
#5961=CARTESIAN_POINT ( 'NONE',  ( -60.99999999999998579, 13.19791666598386826, 2.077350269189628840 ) ) ;
#5964=FACE_OUTER_BOUND ( 'NONE', #9758, .T. ) ;
#5965=CARTESIAN_POINT ( 'NONE',  ( -61.56765823437498852, 11.53645833299193590, 2.248837904296538515 ) ) ;
#5966=CARTESIAN_POINT ( 'NONE',  ( -62.26794919243111082, 15.67633545031536713, 2.500000000000003109 ) ) ;
#5968=CARTESIAN_POINT ( 'NONE',  ( -62.99999999999998579, 12.87500000000000178, 1.500000000000001998 ) ) ;
#5969=CARTESIAN_POINT ( 'NONE',  ( -62.43234176562498305, 13.22395833299193413, 0.7511620957034662593 ) ) ;
#5972=CARTESIAN_POINT ( 'NONE',  ( -62.99999999999998579, 9.593749999317202182, 1.500000000000001998 ) ) ;
#5976=CARTESIAN_POINT ( 'NONE',  ( -60.99999999999998579, 14.77083333333333215, 0.9226497308103762673 ) ) ;
#5977=CARTESIAN_POINT ( 'NONE',  ( -61.13531646874998415, 11.55729166632526983, 1.999225269531026417 ) ) ;
#5980=CARTESIAN_POINT ( 'NONE',  ( -61.99999999999998579, 9.078124999658601979, 2.498450539062049724 ) ) ;
#5981=CARTESIAN_POINT ( 'NONE',  ( -61.73205080756886076, 14.19866454968462932, 2.500000000000003109 ) ) ;
#5982=CARTESIAN_POINT ( 'NONE',  ( -62.43234176562499016, 12.80729166632526805, 2.248837904296538071 ) ) ;
#5983=CARTESIAN_POINT ( 'NONE',  ( -61.49999999999998579, 13.20833333333333215, 2.366025403784441927 ) ) ;
#5984=ORIENTED_EDGE ( 'NONE', *, *, #4052, .T. ) ;
#5985=( BOUNDED_CURVE ( )  B_SPLINE_CURVE ( 2, ( #79, #1976, #5346, #3465, #6315, #8982, #9813, #9869, #6432 ),
 .UNSPECIFIED., .F., .T. ) 
 B_SPLINE_CURVE_WITH_KNOTS ( ( 3, 2, 2, 2, 3 ),
 ( 0.03906250000000002082, 0.04166666666666666435, 0.04687500000000000000, 0.05208333333333333565, 0.05468749999999997918 ),
 .UNSPECIFIED. ) 
 CURVE ( )  GEOMETRIC_REPRESENTATION_ITEM ( )  RATIONAL_B_SPLINE_CURVE ( ( 0.9330127018922192983, 0.9330127018922198534, 1.000000000000000000, 0.8660254037844387076, 1.000000000000000000, 0.8660254037844387076, 1.000000000000000000, 0.9330127018922198534, 0.9330127018922192983 ) ) 
 REPRESENTATION_ITEM ( '' )  );
#5993=CARTESIAN_POINT ( 'NONE',  ( -62.86468353124999453, 15.20312499965860020, 1.500000000000002220 ) ) ;
#5994=CARTESIAN_POINT ( 'NONE',  ( -62.26794919243111082, 9.926335450315368902, 2.500000000000003109 ) ) ;
#5997=CARTESIAN_POINT ( 'NONE',  ( -61.99999999999999289, 14.70312499965860020, 0.5015494609379544944 ) ) ;
#5998=CARTESIAN_POINT ( 'NONE',  ( -62.86468353124998032, 8.932291666325268054, 1.000774730468978246 ) ) ;
#6001=CARTESIAN_POINT ( 'NONE',  ( -62.86468353124999453, 8.515624999658601979, 1.500000000000002220 ) ) ;
#6003=PLANE ( 'NONE',  #390 ) ;
#6004=VERTEX_POINT ( 'NONE', #8843 ) ;
#6006=CARTESIAN_POINT ( 'NONE',  ( -61.99999999999998579, 11.15624999931720218, 2.500000000000002665 ) ) ;
#6009=CARTESIAN_POINT ( 'NONE',  ( -61.56765823437498852, 15.28645833299193590, 2.248837904296538515 ) ) ;
#6010=CARTESIAN_POINT ( 'NONE',  ( -61.99999999999998579, 11.39062499965859843, 0.5015494609379544944 ) ) ;
#6011=CARTESIAN_POINT ( 'NONE',  ( -61.99999999999999289, 8.765624999658601979, 2.498450539062049724 ) ) ;
#6013=CARTESIAN_POINT ( 'NONE',  ( -61.49999999999998579, 9.760416665983870033, 0.6339745962155628467 ) ) ;
#6015=CARTESIAN_POINT ( 'NONE',  ( -62.49999999999998579, 15.66666666666666607, 2.366025403784441483 ) ) ;
#6016=CARTESIAN_POINT ( 'NONE',  ( -61.56765823437498142, 8.682291666325268054, 0.7511620957034663704 ) ) ;
#6018=VECTOR ( 'NONE', #6740, 1000.000000000000000 ) ;
#6019=CARTESIAN_POINT ( 'NONE',  ( -61.49999999999998579, 12.76041666598386826, 0.6339745962155628467 ) ) ;
#6021=ORIENTED_EDGE ( 'NONE', *, *, #9712, .F. ) ;
#6024=CARTESIAN_POINT ( 'NONE',  ( -62.86468353124999453, 11.45312499965860020, 1.500000000000002220 ) ) ;
#6027=DIRECTION ( 'NONE',  ( 0.000000000000000000, 0.000000000000000000, 1.000000000000000000 ) ) ;
#6031=CARTESIAN_POINT ( 'NONE',  ( -61.99999999999998579, 12.57812499965860198, 2.498450539062049724 ) ) ;
#6032=DIRECTION ( 'NONE',  ( -0.000000000000000000, -1.000000000000000000, -0.000000000000000000 ) ) ;
#6033=CARTESIAN_POINT ( 'NONE',  ( -60.99999999999998579, 9.197916665983870033, 2.077350269189628840 ) ) ;
#6035=CARTESIAN_POINT ( 'NONE',  ( -61.99999999999998579, 13.56249999999999822, 0.5000000000000013323 ) ) ;
#6037=FACE_OUTER_BOUND ( 'NONE', #370, .T. ) ;
#6038=CARTESIAN_POINT ( 'NONE',  ( -61.99999999999998579, 11.76562499965860198, 2.498450539062049724 ) ) ;
#6041=CARTESIAN_POINT ( 'NONE',  ( -62.43234176562498305, 8.723958332991934128, 0.7511620957034662593 ) ) ;
#6042=CARTESIAN_POINT ( 'NONE',  ( -61.99999999999998579, 10.40624999931720218, 2.500000000000002665 ) ) ;
#6043=CARTESIAN_POINT ( 'NONE',  ( -61.56765823437498142, 13.43229166632526805, 0.7511620957034663704 ) ) ;
#6045=ORIENTED_EDGE ( 'NONE', *, *, #10296, .F. ) ;
#6048=CARTESIAN_POINT ( 'NONE',  ( -60.99999999999998579, 13.23958333265053611, 0.9226497308103762673 ) ) ;
#6049=CARTESIAN_POINT ( 'NONE',  ( -61.99999999999998579, 15.01562499965860198, 2.498450539062049724 ) ) ;
#6050=DIRECTION ( 'NONE',  ( -0.000000000000000000, -1.000000000000000000, -0.000000000000000000 ) ) ;
#6051=CARTESIAN_POINT ( 'NONE',  ( -61.99999999999998579, 26.00000000000000355, 1.500000000000002220 ) ) ;
#6052=EDGE_CURVE ( 'NONE', #424, #6502, #318, .T. ) ;
#6054=CARTESIAN_POINT ( 'NONE',  ( -62.86468353124999453, 14.03645833299193413, 1.999225269531025750 ) ) ;
#6055=CARTESIAN_POINT ( 'NONE',  ( -61.56765823437498852, 9.286458332991935904, 2.248837904296538515 ) ) ;
#6057=( BOUNDED_CURVE ( )  B_SPLINE_CURVE ( 2, ( #10053, #5730, #2500, #4886, #8396, #3282, #1673, #7615, #7560 ),
 .UNSPECIFIED., .F., .T. ) 
 B_SPLINE_CURVE_WITH_KNOTS ( ( 3, 2, 2, 2, 3 ),
 ( 0.4765625000000000000, 0.4791666666666666852, 0.4843750000000000000, 0.4895833333333333148, 0.4921875000000000000 ),
 .UNSPECIFIED. ) 
 CURVE ( )  GEOMETRIC_REPRESENTATION_ITEM ( )  RATIONAL_B_SPLINE_CURVE ( ( 0.9330127018922194093, 0.9330127018922194093, 1.000000000000000000, 0.8660254037844387076, 1.000000000000000000, 0.8660254037844387076, 1.000000000000000000, 0.9330127018922194093, 0.9330127018922194093 ) ) 
 REPRESENTATION_ITEM ( '' )  );
#6060=CARTESIAN_POINT ( 'NONE',  ( -61.13531646874998415, 9.619791666325268054, 1.999225269531026417 ) ) ;
#6061=CARTESIAN_POINT ( 'NONE',  ( -61.49999999999998579, 15.76041666598386826, 0.6339745962155628467 ) ) ;
#6063=CARTESIAN_POINT ( 'NONE',  ( -61.99999999999998579, 16.00000000000000000, 0.5000000000000041078 ) ) ;
#6066=CARTESIAN_POINT ( 'NONE',  ( -61.56765823437498142, 15.86979166632526628, 0.7511620957034663704 ) ) ;
#6067=CARTESIAN_POINT ( 'NONE',  ( -61.13531646874998415, 11.32812499965860020, 1.500000000000002220 ) ) ;
#6068=CARTESIAN_POINT ( 'NONE',  ( -61.13531646874997705, 9.057291666325266277, 1.999225269531026417 ) ) ;
#6071=CARTESIAN_POINT ( 'NONE',  ( -60.99999999999998579, 15.52083333333333215, 0.9226497308103762673 ) ) ;
#6072=CARTESIAN_POINT ( 'NONE',  ( -62.86468353124998032, 10.24479166632526628, 1.000774730468978024 ) ) ;
#6074=CARTESIAN_POINT ( 'NONE',  ( -60.99999999999998579, 13.69791666598386826, 2.077350269189628840 ) ) ;
#6078=AXIS2_PLACEMENT_3D ( 'NONE', #8608, #2604, #2498 ) ;
#6079=CARTESIAN_POINT ( 'NONE',  ( -61.99999999999998579, 11.68749999999999822, 2.500000000000002665 ) ) ;
#6080=CARTESIAN_POINT ( 'NONE',  ( -62.86468353124998032, 11.43229166632526805, 1.000774730468978024 ) ) ;
#6081=ORIENTED_EDGE ( 'NONE', *, *, #9667, .F. ) ;
#6082=CARTESIAN_POINT ( 'NONE',  ( -60.99999999999998579, 11.75000000000000000, 1.500000000000002220 ) ) ;
#6084=EDGE_CURVE ( 'NONE', #5526, #9814, #9329, .T. ) ;
#6086=CARTESIAN_POINT ( 'NONE',  ( -61.13531646874998415, 14.16145833299193413, 1.000774730468978468 ) ) ;
#6089=CARTESIAN_POINT ( 'NONE',  ( -62.99999999999998579, 9.072916665983868256, 0.9226497308103756012 ) ) ;
#6094=CARTESIAN_POINT ( 'NONE',  ( -62.49999999999998579, 13.33333333333333215, 0.6339745962155627357 ) ) ;
#6095=CARTESIAN_POINT ( 'NONE',  ( -62.86468353124998742, 11.22395833299193590, 1.999225269531025972 ) ) ;
#6098=CARTESIAN_POINT ( 'NONE',  ( -61.56765823437498142, 8.932291666325268054, 0.7511620957034663704 ) ) ;
#6100=CARTESIAN_POINT ( 'NONE',  ( -62.43234176562499016, 14.05729166632526805, 2.248837904296538071 ) ) ;
#6101=CARTESIAN_POINT ( 'NONE',  ( -62.99999999999998579, 12.09374999931720218, 1.500000000000001998 ) ) ;
#6103=CARTESIAN_POINT ( 'NONE',  ( -61.99999999999998579, 12.90624999931720218, 2.500000000000002665 ) ) ;
#6104=EDGE_CURVE ( 'NONE', #9827, #5253, #3653, .T. ) ;
#6107=CARTESIAN_POINT ( 'NONE',  ( -61.49999999999998579, 8.708333333333333925, 2.366025403784441927 ) ) ;
#6109=CARTESIAN_POINT ( 'NONE',  ( -61.49999999999998579, 12.54166666666666607, 0.6339745962155628467 ) ) ;
#6111=CARTESIAN_POINT ( 'NONE',  ( -62.43234176562498305, 13.47395833299193413, 0.7511620957034662593 ) ) ;
#6112=CARTESIAN_POINT ( 'NONE',  ( -62.86468353124998032, 8.182291666325269830, 1.000774730468978246 ) ) ;
#6113=CARTESIAN_POINT ( 'NONE',  ( -61.99999999999998579, 16.00000000000000000, 0.5000000000000041078 ) ) ;
#6115=CARTESIAN_POINT ( 'NONE',  ( -61.13531646874998415, 11.11979166632526805, 1.999225269531026417 ) ) ;
#6116=DIRECTION ( 'NONE',  ( -0.000000000000000000, -1.000000000000000000, -0.000000000000000000 ) ) ;
#6119=CARTESIAN_POINT ( 'NONE',  ( -61.99999999999998579, 12.68750000000000000, 2.500000000000002665 ) ) ;
#6120=CARTESIAN_POINT ( 'NONE',  ( -61.56765823437498142, 15.36979166632526805, 0.7511620957034663704 ) ) ;
#6121=CARTESIAN_POINT ( 'NONE',  ( -61.56765823437498142, 12.86979166632526805, 0.7511620957034663704 ) ) ;
#6122=CARTESIAN_POINT ( 'NONE',  ( -61.56765823437498852, 9.036458332991935904, 2.248837904296538515 ) ) ;
#6124=( BOUNDED_CURVE ( )  B_SPLINE_CURVE ( 2, ( #849, #10026, #4230, #2467, #3348, #6751, #800, #73, #3456, #7530, #7578, #5799, #9250, #10911, #8578, #900, #9403, #9348, #3398, #10960, #2628, #4178, #21, #5066, #6806, #10122, #6016, #10178, #4134, #1797, #8464, #6855, #2521, #5911, #4964, #5168, #1637, #5015, #8417, #3300, #5960, #10071, #4282, #9301, #8520, #1691, #9198, #5855, #2574, #1742, #5115, #7691, #750, #10859, #4079, #3247, #7480, #6651, #2409, #1580, #8365, #7857, #10458, #4455, #7972, #7746, #6965, #6305, #240, #7802, #10399, #5452, #124, #10346, #5397, #8748, #3511, #6247, #3625, #1186, #5336, #2743, #2860, #1068, #1966, #5278, #6185, #1129, #4511, #4564, #7914, #8804, #10283, #6914, #185, #1907, #4390, #1856, #2688, #1008, #6129, #6072, #2917, #9632, #9457, #355, #9513, #5224, #2026, #294, #7077, #8630, #8687, #2797, #3565, #3742, #7139, #7020, #9573, #10520, #3677, #9687, #2080, #955, #4334, #1364, #10575, #3028, #1307, #7193, #7406, #4790, #4731, #6420, #4011, #2971, #529, #3178, #3804, #1413, #10788, #3857, #2296, #5625, #419, #3129, #8141, #9075, #2246, #9803, #10743, #472, #3913, #10689, #1466, #8195, #8972, #3966, #9020, #6526, #5516, #4627, #8090, #2197, #4683, #9744, #6357, #8919, #7246, #10628, #581, #9908, #8029, #2344, #2141, #6584, #5575, #7304, #5682, #3079, #6477, #9858, #7355, #4840, #8248, #632, #9963, #8860, #1247, #3383, #6788, #5733, #1562, #10895, #7512, #5837, #9234, #7463, #7674, #1514, #10160, #3285, #886, #4061, #8399, #56, #676, #10209, #2557, #3440, #3, #5048, #1618, #4265, #4162, #8349, #10940, #1723, #10841, #783, #6680, #5782, #6838, #6733, #5098, #2444, #7563, #6633, #9127, #10056, #4996, #3329, #4945, #7618, #8448, #8503, #832, #4889, #10107, #4213, #732, #8291, #5944, #9331, #3226, #10010, #2392, #9284, #1676, #2503, #9176, #4115, #5892, #166, #9496, #1113, #6111, #9612, #9386, #8613, #7953, #7784, #8559, #5153, #7899, #1891, #2844, #7006, #3551, #4494, #5210, #5262, #4437, #6231, #9555, #2728, #8729, #10384, #277, #10266, #1781, #1839, #6948, #6054, #3492, #940, #2674, #992, #9441, #1949, #3662, #4319, #7121, #7729, #335, #4372, #10327, #7058, #108, #8667, #3723, #1049, #10439, #2007, #7838, #223, #5381, #3609, #8787, #1168, #2609, #2780, #6167, #5318, #4547, #5997, #6894, #3785, #10501, #397, #4609, #2900, #9672, #1228, #6287, #2063, #5436, #8841, #8012, #4226, #9297, #5851, #5110, #8413, #1575, #4174, #5956, #691, #5011, #4130, #5745, #896, #10955, #9344, #6692, #796, #10855, #4277, #7526, #10907, #3296, #9192, #845, #1687, #1737, #5062, #8516, #7574, #8460, #4960, #7686, #8361, #2517, #2570, #6647, #9139, #7631, #1528, #5907, #69, #3343, #9975, #5795, #6802, #3452, #6746, #10118, #3394, #3242, #16, #10174, #746, #2357, #4902, #8302 ),
 .UNSPECIFIED., .F., .T. ) 
 B_SPLINE_CURVE_WITH_KNOTS ( ( 3, 2, 2, 2, 2, 2, 2, 2, 2, 2, 2, 2, 2, 2, 2, 2, 2, 2, 2, 2, 2, 2, 2, 2, 2, 2, 2, 2, 2, 2, 2, 2, 2, 2, 2, 2, 2, 2, 2, 2, 2, 2, 2, 2, 2, 2, 2, 2, 2, 2, 2, 2, 2, 2, 2, 2, 2, 2, 2, 2, 2, 2, 2, 2, 2, 2, 2, 2, 2, 2, 2, 2, 2, 2, 2, 2, 2, 2, 2, 2, 2, 2, 2, 2, 2, 2, 2, 2, 2, 2, 2, 2, 2, 2, 2, 2, 2, 2, 2, 2, 2, 2, 2, 2, 2, 2, 2, 2, 2, 2, 2, 2, 2, 2, 2, 2, 2, 2, 2, 2, 2, 2, 2, 2, 2, 2, 2, 2, 2, 2, 2, 2, 2, 2, 2, 2, 2, 2, 2, 2, 2, 2, 2, 2, 2, 2, 2, 2, 2, 2, 2, 2, 2, 2, 2, 2, 2, 2, 2, 2, 2, 2, 2, 2, 2, 2, 2, 2, 2, 2, 2, 2, 2, 2, 2, 2, 2, 2, 2, 2, 2, 2, 2, 2, 2, 2, 2, 2, 2, 2, 2, 2, 3 ),
 ( 0.000000000000000000, 0.005208333333333333044, 0.01041666666666666609, 0.01562500000000000000, 0.02083333333333333218, 0.02604166666666666782, 0.03125000000000000000, 0.03645833333333333565, 0.04166666666666666435, 0.04687500000000000000, 0.05208333333333333565, 0.05729166666666666435, 0.06250000000000000000, 0.06770833333333332871, 0.07291666666666667129, 0.07812500000000000000, 0.08333333333333332871, 0.08854166666666667129, 0.09375000000000000000, 0.09895833333333332871, 0.1041666666666666713, 0.1093750000000000000, 0.1145833333333333287, 0.1197916666666666713, 0.1250000000000000000, 0.1302083333333333426, 0.1354166666666666574, 0.1406250000000000000, 0.1458333333333333426, 0.1510416666666666574, 0.1562500000000000000, 0.1614583333333333426, 0.1666666666666666574, 0.1718750000000000000, 0.1770833333333333426, 0.1822916666666666574, 0.1875000000000000000, 0.1927083333333333426, 0.1979166666666666574, 0.2031250000000000000, 0.2083333333333333426, 0.2135416666666666574, 0.2187500000000000000, 0.2239583333333333426, 0.2291666666666666574, 0.2343750000000000000, 0.2395833333333333426, 0.2447916666666666574, 0.2500000000000000000, 0.2552083333333333148, 0.2604166666666666852, 0.2656250000000000000, 0.2708333333333333148, 0.2760416666666666852, 0.2812500000000000000, 0.2864583333333333148, 0.2916666666666666852, 0.2968750000000000000, 0.3020833333333333148, 0.3072916666666666852, 0.3125000000000000000, 0.3177083333333333148, 0.3229166666666666852, 0.3281250000000000000, 0.3333333333333333148, 0.3385416666666666852, 0.3437500000000000000, 0.3489583333333333148, 0.3541666666666666852, 0.3593750000000000000, 0.3645833333333333148, 0.3697916666666666852, 0.3750000000000000000, 0.3802083333333333148, 0.3854166666666666852, 0.3906250000000000000, 0.3958333333333333148, 0.4010416666666666852, 0.4062500000000000000, 0.4114583333333333148, 0.4166666666666666852, 0.4218750000000000000, 0.4270833333333333148, 0.4322916666666666852, 0.4375000000000000000, 0.4427083333333333148, 0.4479166666666666852, 0.4531250000000000000, 0.4583333333333333148, 0.4635416666666666852, 0.4687500000000000000, 0.4739583333333333148, 0.4791666666666666852, 0.4843750000000000000, 0.4895833333333333148, 0.4947916666666666852, 0.5000000000000000000, 0.5052083333333333703, 0.5104166666666666297, 0.5156250000000000000, 0.5208333333333333703, 0.5260416666666666297, 0.5312500000000000000, 0.5364583333333333703, 0.5416666666666666297, 0.5468750000000000000, 0.5520833333333333703, 0.5572916666666666297, 0.5625000000000000000, 0.5677083333333333703, 0.5729166666666666297, 0.5781250000000000000, 0.5833333333333333703, 0.5885416666666666297, 0.5937500000000000000, 0.5989583333333333703, 0.6041666666666666297, 0.6093750000000000000, 0.6145833333333333703, 0.6197916666666666297, 0.6250000000000000000, 0.6302083333333333703, 0.6354166666666666297, 0.6406250000000000000, 0.6458333333333333703, 0.6510416666666666297, 0.6562500000000000000, 0.6614583333333333703, 0.6666666666666666297, 0.6718750000000000000, 0.6770833333333333703, 0.6822916666666666297, 0.6875000000000000000, 0.6927083333333333703, 0.6979166666666666297, 0.7031250000000000000, 0.7083333333333333703, 0.7135416666666666297, 0.7187500000000000000, 0.7239583333333333703, 0.7291666666666666297, 0.7343750000000000000, 0.7395833333333333703, 0.7447916666666666297, 0.7500000000000000000, 0.7552083333333333703, 0.7604166666666666297, 0.7656250000000000000, 0.7708333333333333703, 0.7760416666666666297, 0.7812500000000000000, 0.7864583333333333703, 0.7916666666666666297, 0.7968750000000000000, 0.8020833333333333703, 0.8072916666666666297, 0.8125000000000000000, 0.8177083333333333703, 0.8229166666666666297, 0.8281250000000000000, 0.8333333333333333703, 0.8385416666666666297, 0.8437500000000000000, 0.8489583333333333703, 0.8541666666666666297, 0.8593750000000000000, 0.8645833333333333703, 0.8697916666666666297, 0.8750000000000000000, 0.8802083333333333703, 0.8854166666666666297, 0.8906250000000000000, 0.8958333333333333703, 0.9010416666666666297, 0.9062500000000000000, 0.9114583333333333703, 0.9166666666666666297, 0.9218750000000000000, 0.9270833333333333703, 0.9322916666666666297, 0.9375000000000000000, 0.9427083333333333703, 0.9479166666666666297, 0.9531250000000000000, 0.9583333333333333703, 0.9635416666666666297, 0.9687500000000000000, 0.9739583333333333703, 0.9791666666666666297, 0.9843750000000000000, 0.9895833333333333703, 0.9947916666666666297, 1.000000000000000000 ),
 .UNSPECIFIED. ) 
 CURVE ( )  GEOMETRIC_REPRESENTATION_ITEM ( )  RATIONAL_B_SPLINE_CURVE ( ( 1.000000000000000000, 0.8660254037844387076, 1.000000000000000000, 0.8660254037844387076, 1.000000000000000000, 0.8660254037844387076, 1.000000000000000000, 0.8660254037844387076, 1.000000000000000000, 0.8660254037844387076, 1.000000000000000000, 0.8660254037844387076, 1.000000000000000000, 0.8660254037844387076, 1.000000000000000000, 0.8660254037844387076, 1.000000000000000000, 0.8660254037844387076, 1.000000000000000000, 0.8660254037844387076, 1.000000000000000000, 0.8660254037844387076, 1.000000000000000000, 0.8660254037844387076, 1.000000000000000000, 0.8660254037844387076, 1.000000000000000000, 0.8660254037844387076, 1.000000000000000000, 0.8660254037844387076, 1.000000000000000000, 0.8660254037844387076, 1.000000000000000000, 0.8660254037844387076, 1.000000000000000000, 0.8660254037844387076, 1.000000000000000000, 0.8660254037844387076, 1.000000000000000000, 0.8660254037844387076, 1.000000000000000000, 0.8660254037844387076, 1.000000000000000000, 0.8660254037844387076, 1.000000000000000000, 0.8660254037844387076, 1.000000000000000000, 0.8660254037844387076, 1.000000000000000000, 0.8660254037844387076, 1.000000000000000000, 0.8660254037844387076, 1.000000000000000000, 0.8660254037844387076, 1.000000000000000000, 0.8660254037844387076, 1.000000000000000000, 0.8660254037844387076, 1.000000000000000000, 0.8660254037844387076, 1.000000000000000000, 0.8660254037844387076, 1.000000000000000000, 0.8660254037844387076, 1.000000000000000000, 0.8660254037844387076, 1.000000000000000000, 0.8660254037844387076, 1.000000000000000000, 0.8660254037844387076, 1.000000000000000000, 0.8660254037844387076, 1.000000000000000000, 0.8660254037844387076, 1.000000000000000000, 0.8660254037844387076, 1.000000000000000000, 0.8660254037844387076, 1.000000000000000000, 0.8660254037844387076, 1.000000000000000000, 0.8660254037844387076, 1.000000000000000000, 0.8660254037844387076, 1.000000000000000000, 0.8660254037844387076, 1.000000000000000000, 0.8660254037844387076, 1.000000000000000000, 0.8660254037844387076, 1.000000000000000000, 0.8660254037844387076, 1.000000000000000000, 0.8660254037844387076, 1.000000000000000000, 0.8660254037844387076, 1.000000000000000000, 0.8660254037844387076, 1.000000000000000000, 0.8660254037844387076, 1.000000000000000000, 0.8660254037844387076, 1.000000000000000000, 0.8660254037844387076, 1.000000000000000000, 0.8660254037844387076, 1.000000000000000000, 0.8660254037844387076, 1.000000000000000000, 0.8660254037844387076, 1.000000000000000000, 0.8660254037844387076, 1.000000000000000000, 0.8660254037844387076, 1.000000000000000000, 0.8660254037844387076, 1.000000000000000000, 0.8660254037844387076, 1.000000000000000000, 0.8660254037844387076, 1.000000000000000000, 0.8660254037844387076, 1.000000000000000000, 0.8660254037844387076, 1.000000000000000000, 0.8660254037844387076, 1.000000000000000000, 0.8660254037844387076, 1.000000000000000000, 0.8660254037844387076, 1.000000000000000000, 0.8660254037844387076, 1.000000000000000000, 0.8660254037844387076, 1.000000000000000000, 0.8660254037844387076, 1.000000000000000000, 0.8660254037844387076, 1.000000000000000000, 0.8660254037844387076, 1.000000000000000000, 0.8660254037844387076, 1.000000000000000000, 0.8660254037844387076, 1.000000000000000000, 0.8660254037844387076, 1.000000000000000000, 0.8660254037844387076, 1.000000000000000000, 0.8660254037844387076, 1.000000000000000000, 0.8660254037844387076, 1.000000000000000000, 0.8660254037844387076, 1.000000000000000000, 0.8660254037844387076, 1.000000000000000000, 0.8660254037844387076, 1.000000000000000000, 0.8660254037844387076, 1.000000000000000000, 0.8660254037844387076, 1.000000000000000000, 0.8660254037844387076, 1.000000000000000000, 0.8660254037844387076, 1.000000000000000000, 0.8660254037844387076, 1.000000000000000000, 0.8660254037844387076, 1.000000000000000000, 0.8660254037844387076, 1.000000000000000000, 0.8660254037844387076, 1.000000000000000000, 0.8660254037844387076, 1.000000000000000000, 0.8660254037844387076, 1.000000000000000000, 0.8660254037844387076, 1.000000000000000000, 0.8660254037844387076, 1.000000000000000000, 0.8660254037844387076, 1.000000000000000000, 0.8660254037844387076, 1.000000000000000000, 0.8660254037844387076, 1.000000000000000000, 0.8660254037844387076, 1.000000000000000000, 0.8660254037844387076, 1.000000000000000000, 0.8660254037844387076, 1.000000000000000000, 0.8660254037844387076, 1.000000000000000000, 0.8660254037844387076, 1.000000000000000000, 0.8660254037844387076, 1.000000000000000000, 0.8660254037844387076, 1.000000000000000000, 0.8660254037844387076, 1.000000000000000000, 0.8660254037844387076, 1.000000000000000000, 0.8660254037844387076, 1.000000000000000000, 0.8660254037844387076, 1.000000000000000000, 0.8660254037844387076, 1.000000000000000000, 0.8660254037844387076, 1.000000000000000000, 0.8660254037844387076, 1.000000000000000000, 0.8660254037844387076, 1.000000000000000000, 0.8660254037844387076, 1.000000000000000000, 0.8660254037844387076, 1.000000000000000000, 0.8660254037844387076, 1.000000000000000000, 0.8660254037844387076, 1.000000000000000000, 0.8660254037844387076, 1.000000000000000000, 0.8660254037844387076, 1.000000000000000000, 0.8660254037844387076, 1.000000000000000000, 0.8660254037844387076, 1.000000000000000000, 0.8660254037844387076, 1.000000000000000000, 0.8660254037844387076, 1.000000000000000000, 0.8660254037844387076, 1.000000000000000000, 0.8660254037844387076, 1.000000000000000000, 0.8660254037844387076, 1.000000000000000000, 0.8660254037844387076, 1.000000000000000000, 0.8660254037844387076, 1.000000000000000000, 0.8660254037844387076, 1.000000000000000000, 0.8660254037844387076, 1.000000000000000000, 0.8660254037844387076, 1.000000000000000000, 0.8660254037844387076, 1.000000000000000000, 0.8660254037844387076, 1.000000000000000000, 0.8660254037844387076, 1.000000000000000000, 0.8660254037844387076, 1.000000000000000000, 0.8660254037844387076, 1.000000000000000000, 0.8660254037844387076, 1.000000000000000000, 0.8660254037844387076, 1.000000000000000000, 0.8660254037844387076, 1.000000000000000000, 0.8660254037844387076, 1.000000000000000000, 0.8660254037844387076, 1.000000000000000000, 0.8660254037844387076, 1.000000000000000000, 0.8660254037844387076, 1.000000000000000000, 0.8660254037844387076, 1.000000000000000000, 0.8660254037844387076, 1.000000000000000000, 0.8660254037844387076, 1.000000000000000000, 0.8660254037844387076, 1.000000000000000000, 0.8660254037844387076, 1.000000000000000000, 0.8660254037844387076, 1.000000000000000000, 0.8660254037844387076, 1.000000000000000000, 0.8660254037844387076, 1.000000000000000000, 0.8660254037844387076, 1.000000000000000000, 0.8660254037844387076, 1.000000000000000000, 0.8660254037844387076, 1.000000000000000000, 0.8660254037844387076, 1.000000000000000000, 0.8660254037844387076, 1.000000000000000000, 0.8660254037844387076, 1.000000000000000000, 0.8660254037844387076, 1.000000000000000000, 0.8660254037844387076, 1.000000000000000000, 0.8660254037844387076, 1.000000000000000000, 0.8660254037844387076, 1.000000000000000000, 0.8660254037844387076, 1.000000000000000000, 0.8660254037844387076, 1.000000000000000000, 0.8660254037844387076, 1.000000000000000000, 0.8660254037844387076, 1.000000000000000000, 0.8660254037844387076, 1.000000000000000000, 0.8660254037844387076, 1.000000000000000000, 0.8660254037844387076, 1.000000000000000000, 0.8660254037844387076, 1.000000000000000000, 0.8660254037844387076, 1.000000000000000000, 0.8660254037844387076, 1.000000000000000000, 0.8660254037844387076, 1.000000000000000000, 0.8660254037844387076, 1.000000000000000000, 0.8660254037844387076, 1.000000000000000000, 0.8660254037844387076, 1.000000000000000000, 0.8660254037844387076, 1.000000000000000000, 0.8660254037844387076, 1.000000000000000000, 0.8660254037844387076, 1.000000000000000000, 0.8660254037844387076, 1.000000000000000000, 0.8660254037844387076, 1.000000000000000000, 0.8660254037844387076, 1.000000000000000000, 0.8660254037844387076, 1.000000000000000000, 0.8660254037844387076, 1.000000000000000000, 0.8660254037844387076, 1.000000000000000000, 0.8660254037844387076, 1.000000000000000000, 0.8660254037844387076, 1.000000000000000000, 0.8660254037844387076, 1.000000000000000000, 0.8660254037844387076, 1.000000000000000000, 0.8660254037844387076, 1.000000000000000000, 0.8660254037844387076, 1.000000000000000000, 0.8660254037844387076, 1.000000000000000000, 0.8660254037844387076, 1.000000000000000000, 0.8660254037844387076, 1.000000000000000000, 0.8660254037844387076, 1.000000000000000000, 0.8660254037844387076, 1.000000000000000000, 0.8660254037844387076, 1.000000000000000000 ) ) 
 REPRESENTATION_ITEM ( '' )  );
#6125=ORIENTED_EDGE ( 'NONE', *, *, #3494, .F. ) ;
#6126=CARTESIAN_POINT ( 'NONE',  ( -61.49999999999998579, 15.45833333333333393, 2.366025403784441927 ) ) ;
#6127=ADVANCED_FACE ( 'NONE', ( #5501 ), #9113, .T. ) ;
#6129=CARTESIAN_POINT ( 'NONE',  ( -62.43234176562498305, 10.22395833299193413, 0.7511620957034662593 ) ) ;
#6131=CARTESIAN_POINT ( 'NONE',  ( -62.43234176562499016, 15.49479166632526628, 2.248837904296538071 ) ) ;
#6132=CARTESIAN_POINT ( 'NONE',  ( -60.99999999999998579, 13.44791666598387003, 2.077350269189628840 ) ) ;
#6136=CARTESIAN_POINT ( 'NONE',  ( -62.43234176562498305, 11.66145833299193590, 0.7511620957034662593 ) ) ;
#6137=CARTESIAN_POINT ( 'NONE',  ( -61.99999999999998579, 16.00000000000000000, 1.500000000000002220 ) ) ;
#6138=CARTESIAN_POINT ( 'NONE',  ( -61.99999999999998579, 16.00000000000000000, 1.500000000000002220 ) ) ;
#6140=CARTESIAN_POINT ( 'NONE',  ( -61.49999999999998579, 10.70833333333333393, 2.366025403784441927 ) ) ;
#6141=CARTESIAN_POINT ( 'NONE',  ( -61.99999999999998579, 16.00000000000000000, 0.5000000000000041078 ) ) ;
#6142=CARTESIAN_POINT ( 'NONE',  ( -61.99999999999998579, 13.95312499965860198, 0.5015494609379544944 ) ) ;
#6145=CARTESIAN_POINT ( 'NONE',  ( -61.49999999999998579, 9.510416665983870033, 0.6339745962155628467 ) ) ;
#6148=ADVANCED_FACE ( 'NONE', ( #5561 ), #9951, .T. ) ;
#6149=CARTESIAN_POINT ( 'NONE',  ( -62.49999999999998579, 15.30208333265053611, 0.6339745962155627357 ) ) ;
#6150=CARTESIAN_POINT ( 'NONE',  ( -62.86468353124999453, 11.20312499965860020, 1.500000000000002220 ) ) ;
#6153=ORIENTED_EDGE ( 'NONE', *, *, #697, .T. ) ;
#6154=CARTESIAN_POINT ( 'NONE',  ( -61.13531646874998415, 10.11979166632526805, 1.999225269531026417 ) ) ;
#6156=SHAPE_REPRESENTATION ( 'clamp screw', ( #2307 ), #9766 ) ;
#6157=CARTESIAN_POINT ( 'NONE',  ( -61.56765823437498852, 14.84895833299193413, 2.248837904296538515 ) ) ;
#6159=ORIENTED_EDGE ( 'NONE', *, *, #2324, .F. ) ;
#6162=CARTESIAN_POINT ( 'NONE',  ( -61.99999999999998579, 12.78124999931720218, 0.5000000000000013323 ) ) ;
#6163=CARTESIAN_POINT ( 'NONE',  ( -61.99999999999998579, 16.01562499965860198, 2.498450539062049724 ) ) ;
#6166=CARTESIAN_POINT ( 'NONE',  ( -62.99999999999998579, 8.895833333333333925, 2.077350269189627952 ) ) ;
#6167=CARTESIAN_POINT ( 'NONE',  ( -61.13531646874998415, 14.64062499965860020, 1.500000000000002220 ) ) ;
#6169=CARTESIAN_POINT ( 'NONE',  ( -62.86468353124998742, 9.473958332991934128, 1.999225269531025972 ) ) ;
#6172=VECTOR ( 'NONE', #1513, 1000.000000000000000 ) ;
#6173=CARTESIAN_POINT ( 'NONE',  ( -61.56765823437498142, 9.932291666325268054, 0.7511620957034663704 ) ) ;
#6174=CARTESIAN_POINT ( 'NONE',  ( -62.49999999999998579, 14.13541666598387003, 2.366025403784441483 ) ) ;
#6177=CARTESIAN_POINT ( 'NONE',  ( -62.49999999999998579, 11.41666666666666785, 2.366025403784441483 ) ) ;
#6178=CARTESIAN_POINT ( 'NONE',  ( -61.73205080756886076, 9.948664549684629321, 2.500000000000003109 ) ) ;
#6179=CARTESIAN_POINT ( 'NONE',  ( -62.86468353124999453, 11.95312499965860198, 1.500000000000002220 ) ) ;
#6181=CARTESIAN_POINT ( 'NONE',  ( -62.86468353124999453, 8.723958332991934128, 1.999225269531025750 ) ) ;
#6184=CYLINDRICAL_SURFACE ( 'NONE', #1736, 0.9999999999999981126 ) ;
#6185=CARTESIAN_POINT ( 'NONE',  ( -61.56765823437498142, 9.932291666325268054, 0.7511620957034663704 ) ) ;
#6186=AXIS2_PLACEMENT_3D ( 'NONE', #6510, #10671, #5557 ) ;
#6188=CARTESIAN_POINT ( 'NONE',  ( -62.86468353124998032, 15.93229166632526805, 1.000774730468978246 ) ) ;
#6189=CARTESIAN_POINT ( 'NONE',  ( -60.99999999999998579, 14.96874999931720218, 1.500000000000002220 ) ) ;
#6191=ORIENTED_EDGE ( 'NONE', *, *, #8005, .T. ) ;
#6194=CARTESIAN_POINT ( 'NONE',  ( -62.43234176562499016, 11.74479166632526805, 2.248837904296538071 ) ) ;
#6195=CARTESIAN_POINT ( 'NONE',  ( -62.43234176562499016, 8.494791666325268054, 2.248837904296538071 ) ) ;
#6197=ORIENTED_EDGE ( 'NONE', *, *, #5919, .T. ) ;
#6198=CARTESIAN_POINT ( 'NONE',  ( -62.99999999999998579, 12.89583333333333037, 2.077350269189627952 ) ) ;
#6201=CARTESIAN_POINT ( 'NONE',  ( -61.56765823437498852, 13.84895833299193413, 2.248837904296538515 ) ) ;
#6202=ADVANCED_FACE ( 'NONE', ( #10612 ), #5929, .T. ) ;
#6204=DIRECTION ( 'NONE',  ( -0.000000000000000000, -1.000000000000000000, -0.000000000000000000 ) ) ;
#6205=CARTESIAN_POINT ( 'NONE',  ( -62.99999999999998579, 10.09374999931720218, 1.500000000000001998 ) ) ;
#6207=ORIENTED_EDGE ( 'NONE', *, *, #320, .T. ) ;
#6208=CARTESIAN_POINT ( 'NONE',  ( -61.73205080756886076, 13.55133545031536890, 0.5000000000000014433 ) ) ;
#6210=CARTESIAN_POINT ( 'NONE',  ( -62.26794919243111082, 13.32366454968462754, 0.5000000000000013323 ) ) ;
#6213=CARTESIAN_POINT ( 'NONE',  ( -62.86468353124998742, 10.72395833299193413, 1.999225269531025972 ) ) ;
#6216=EDGE_LOOP ( 'NONE', ( #6045, #8319, #10087, #9943 ) ) ;
#6217=CARTESIAN_POINT ( 'NONE',  ( -61.99999999999998579, 9.703124999658601979, 0.5015494609379544944 ) ) ;
#6220=CARTESIAN_POINT ( 'NONE',  ( -61.13531646874998415, 13.91145833299193413, 1.000774730468978468 ) ) ;
#6222=ORIENTED_EDGE ( 'NONE', *, *, #6104, .F. ) ;
#6223=CARTESIAN_POINT ( 'NONE',  ( -61.99999999999998579, 16.00000000000000000, 2.500000000000000444 ) ) ;
#6224=VERTEX_POINT ( 'NONE', #4761 ) ;
#6225=CARTESIAN_POINT ( 'NONE',  ( -61.49999999999998579, 8.791666666666666075, 0.6339745962155628467 ) ) ;
#6226=CARTESIAN_POINT ( 'NONE',  ( -62.49999999999998579, 8.166666666666667851, 2.366025403784441483 ) ) ;
#6228=CARTESIAN_POINT ( 'NONE',  ( -61.99999999999998579, 11.06250000000000000, 0.5000000000000013323 ) ) ;
#6231=CARTESIAN_POINT ( 'NONE',  ( -61.99999999999999289, 13.82812499965860198, 2.498450539062049724 ) ) ;
#6232=CARTESIAN_POINT ( 'NONE',  ( -61.56765823437498852, 9.536458332991934128, 2.248837904296538515 ) ) ;
#6233=CARTESIAN_POINT ( 'NONE',  ( -62.49999999999998579, 11.30208333265053611, 0.6339745962155627357 ) ) ;
#6234=CARTESIAN_POINT ( 'NONE',  ( -61.13531646874998415, 10.89062499965860020, 1.500000000000002220 ) ) ;
#6236=CARTESIAN_POINT ( 'NONE',  ( -61.99999999999998579, 12.06250000000000000, 0.5000000000000013323 ) ) ;
#6239=VERTEX_POINT ( 'NONE', #10721 ) ;
#6240=CARTESIAN_POINT ( 'NONE',  ( -62.26794919243111082, 10.14508544963257108, 2.500000000000000888 ) ) ;
#6241=CARTESIAN_POINT ( 'NONE',  ( -61.13531646874998415, 13.05729166632526628, 1.999225269531026417 ) ) ;
#6242=CARTESIAN_POINT ( 'NONE',  ( -61.99999999999999289, 9.140624999658600203, 0.5015494609379544944 ) ) ;
#6243=CARTESIAN_POINT ( 'NONE',  ( -62.49999999999998579, 8.583333333333333925, 0.6339745962155627357 ) ) ;
#6245=CARTESIAN_POINT ( 'NONE',  ( -62.99999999999998579, 10.82291666598386826, 0.9226497308103756012 ) ) ;
#6247=CARTESIAN_POINT ( 'NONE',  ( -62.86468353124998032, 9.744791666325268054, 1.000774730468978024 ) ) ;
#6249=CARTESIAN_POINT ( 'NONE',  ( -61.13531646874998415, 15.30729166632526983, 1.999225269531026417 ) ) ;
#6250=CARTESIAN_POINT ( 'NONE',  ( -62.99999999999998579, 14.57291666598387181, 0.9226497308103756012 ) ) ;
#6252=ORIENTED_EDGE ( 'NONE', *, *, #4590, .F. ) ;
#6254=EDGE_LOOP ( 'NONE', ( #8419, #5373, #3675, #1057 ) ) ;
#6257=CARTESIAN_POINT ( 'NONE',  ( -61.13531646874997705, 13.05729166632526983, 1.999225269531026417 ) ) ;
#6258=CARTESIAN_POINT ( 'NONE',  ( -61.99999999999998579, 9.015624999658603755, 2.498450539062049724 ) ) ;
#6260=VERTEX_POINT ( 'NONE', #864 ) ;
#6261=CARTESIAN_POINT ( 'NONE',  ( -61.99999999999998579, 11.93750000000000000, 2.654700538379254571 ) ) ;
#6263=CARTESIAN_POINT ( 'NONE',  ( -62.86468353124999453, 14.51562499965860020, 1.500000000000002220 ) ) ;
#6266=CARTESIAN_POINT ( 'NONE',  ( -62.99999999999998579, 10.84374999931720218, 1.500000000000001998 ) ) ;
#6267=ORIENTED_EDGE ( 'NONE', *, *, #10288, .F. ) ;
#6270=CARTESIAN_POINT ( 'NONE',  ( -62.43234176562499016, 11.99479166632526628, 2.248837904296538071 ) ) ;
#6272=CARTESIAN_POINT ( 'NONE',  ( -62.86468353124998742, 10.78645833299193413, 1.999225269531025972 ) ) ;
#6276=CARTESIAN_POINT ( 'NONE',  ( -62.43234176562498305, 14.47395833299193413, 0.7511620957034662593 ) ) ;
#6282=CARTESIAN_POINT ( 'NONE',  ( -61.73205080756886076, 8.698664549684629321, 2.500000000000003109 ) ) ;
#6283=CARTESIAN_POINT ( 'NONE',  ( -60.99999999999998579, 8.520833333333333925, 0.9226497308103762673 ) ) ;
#6285=CARTESIAN_POINT ( 'NONE',  ( -61.99999999999998579, 14.15624999931720218, 2.500000000000002665 ) ) ;
#6286=CARTESIAN_POINT ( 'NONE',  ( -61.73205080756888208, 10.66741454900183328, 2.500000000000006661 ) ) ;
#6287=CARTESIAN_POINT ( 'NONE',  ( -61.13531646874998415, 14.89062499965860020, 1.500000000000002220 ) ) ;
#6288=CARTESIAN_POINT ( 'NONE',  ( -62.43234176562499016, 10.49479166632526983, 2.248837904296538071 ) ) ;
#6291=CARTESIAN_POINT ( 'NONE',  ( -62.26794919243111082, 9.676335450315370679, 2.500000000000003109 ) ) ;
#6292=CARTESIAN_POINT ( 'NONE',  ( -62.86468353124999453, 10.01562499965860198, 1.500000000000002220 ) ) ;
#6293=CARTESIAN_POINT ( 'NONE',  ( -61.99999999999998579, 8.000000000000000000, 1.500000000000002220 ) ) ;
#6297=( BOUNDED_CURVE ( )  B_SPLINE_CURVE ( 2, ( #9757, #4803, #2153, #5525, #369, #5409, #7150, #8929, #8101 ),
 .UNSPECIFIED., .F., .T. ) 
 B_SPLINE_CURVE_WITH_KNOTS ( ( 3, 2, 2, 2, 3 ),
 ( 0.2890624999999999445, 0.2916666666666666852, 0.2968750000000000000, 0.3020833333333333148, 0.3046874999999999445 ),
 .UNSPECIFIED. ) 
 CURVE ( )  GEOMETRIC_REPRESENTATION_ITEM ( )  RATIONAL_B_SPLINE_CURVE ( ( 0.9330127018922192983, 0.9330127018922178550, 1.000000000000000000, 0.8660254037844387076, 1.000000000000000000, 0.8660254037844387076, 1.000000000000000000, 0.9330127018922207416, 0.9330127018922192983 ) ) 
 REPRESENTATION_ITEM ( '' )  );
#6298=VERTEX_POINT ( 'NONE', #5078 ) ;
#6299=CARTESIAN_POINT ( 'NONE',  ( -62.49999999999998579, 10.05208333265053611, 0.6339745962155627357 ) ) ;
#6300=CARTESIAN_POINT ( 'NONE',  ( -61.99999999999998579, 12.39062499965860198, 0.5015494609379544944 ) ) ;
#6302=CARTESIAN_POINT ( 'NONE',  ( -61.99999999999999289, 10.14062499965860198, 0.5015494609379544944 ) ) ;
#6303=ORIENTED_EDGE ( 'NONE', *, *, #1166, .F. ) ;
#6305=CARTESIAN_POINT ( 'NONE',  ( -62.86468353124999453, 9.536458332991935904, 1.999225269531025750 ) ) ;
#6307=CARTESIAN_POINT ( 'NONE',  ( -61.13531646874998415, 15.05729166632526805, 1.999225269531026417 ) ) ;
#6308=CARTESIAN_POINT ( 'NONE',  ( -62.99999999999998579, 14.09374999931720218, 1.500000000000001998 ) ) ;
#6310=ORIENTED_EDGE ( 'NONE', *, *, #3988, .F. ) ;
#6311=CARTESIAN_POINT ( 'NONE',  ( -61.28647452029539267, 16.00000000000000000, 0.7993707187018740390 ) ) ;
#6312=ORIENTED_EDGE ( 'NONE', *, *, #9084, .T. ) ;
#6313=CARTESIAN_POINT ( 'NONE',  ( -62.86468353124998032, 13.18229166632526805, 1.000774730468978024 ) ) ;
#6314=CARTESIAN_POINT ( 'NONE',  ( -61.13531646874998415, 8.807291666325268054, 1.999225269531026417 ) ) ;
#6315=CARTESIAN_POINT ( 'NONE',  ( -62.99999999999998579, 8.375000000000000000, 1.500000000000001998 ) ) ;
#6316=EDGE_LOOP ( 'NONE', ( #5747, #6748, #3647, #10040 ) ) ;
#6317=CARTESIAN_POINT ( 'NONE',  ( -61.99999999999998579, 12.68750000000000000, 2.654700538379254571 ) ) ;
#6319=CARTESIAN_POINT ( 'NONE',  ( -61.13531646874998415, 13.86979166632526805, 1.999225269531026417 ) ) ;
#6323=CARTESIAN_POINT ( 'NONE',  ( -60.99999999999998579, 10.19791666598387181, 2.077350269189628840 ) ) ;
#6326=CARTESIAN_POINT ( 'NONE',  ( -62.99999999999998579, 15.34374999931720218, 1.500000000000001998 ) ) ;
#6327=CARTESIAN_POINT ( 'NONE',  ( -61.99999999999998579, 12.76562499965860198, 2.498450539062049724 ) ) ;
#6330=CARTESIAN_POINT ( 'NONE',  ( -62.86468353124998032, 9.744791666325268054, 1.000774730468978246 ) ) ;
#6332=CARTESIAN_POINT ( 'NONE',  ( -61.13531646874998415, 14.91145833299193413, 1.000774730468978468 ) ) ;
#6333=CARTESIAN_POINT ( 'NONE',  ( -61.99999999999998579, 16.00000000000000000, 1.500000000000002220 ) ) ;
#6334=EDGE_LOOP ( 'NONE', ( #4534, #7518, #8866, #10113 ) ) ;
#6337=CARTESIAN_POINT ( 'NONE',  ( -60.99999999999998579, 12.69791666598386826, 2.077350269189628840 ) ) ;
#6338=CARTESIAN_POINT ( 'NONE',  ( -60.99999999999998579, 8.500000000000000000, 1.500000000000002220 ) ) ;
#6340=DIRECTION ( 'NONE',  ( 0.000000000000000000, 0.000000000000000000, -1.000000000000000000 ) ) ;
#6341=CARTESIAN_POINT ( 'NONE',  ( -62.86468353124998032, 10.43229166632526983, 1.000774730468978246 ) ) ;
#6342=CARTESIAN_POINT ( 'NONE',  ( -61.73205080756886076, 12.02008544963257286, 0.5000000000000014433 ) ) ;
#6343=CARTESIAN_POINT ( 'NONE',  ( -62.99999999999998579, 9.645833333333330373, 2.077350269189627952 ) ) ;
#6344=CARTESIAN_POINT ( 'NONE',  ( -61.56765823437498142, 10.43229166632526983, 0.7511620957034663704 ) ) ;
#6345=CARTESIAN_POINT ( 'NONE',  ( -62.99999999999998579, 13.60416666666666785, 0.9226497308103756012 ) ) ;
#6348=CARTESIAN_POINT ( 'NONE',  ( -61.99999999999998579, 16.00000000000000000, 1.500000000000002220 ) ) ;
#6351=ORIENTED_EDGE ( 'NONE', *, *, #4590, .T. ) ;
#6352=CARTESIAN_POINT ( 'NONE',  ( -62.43234176562499016, 11.99479166632526628, 2.248837904296538071 ) ) ;
#6353=CARTESIAN_POINT ( 'NONE',  ( -62.43234176562499016, 9.994791666325268054, 2.248837904296538071 ) ) ;
#6354=CARTESIAN_POINT ( 'NONE',  ( -61.99999999999998579, 8.562500000000000000, 0.5000000000000013323 ) ) ;
#6357=CARTESIAN_POINT ( 'NONE',  ( -61.56765823437498852, 11.59895833299193590, 2.248837904296538515 ) ) ;
#6358=VECTOR ( 'NONE', #8447, 1000.000000000000000 ) ;
#6359=CARTESIAN_POINT ( 'NONE',  ( -61.99999999999998579, 15.14062499965860198, 0.5015494609379544944 ) ) ;
#6360=CARTESIAN_POINT ( 'NONE',  ( -60.99999999999998579, 15.23958333265053611, 0.9226497308103762673 ) ) ;
#6361=EDGE_LOOP ( 'NONE', ( #4925, #5615, #909, #1815 ) ) ;
#6364=( BOUNDED_CURVE ( )  B_SPLINE_CURVE ( 2, ( #7609, #4989, #878, #4257, #4204, #3432, #776, #3323, #6723 ),
 .UNSPECIFIED., .F., .T. ) 
 B_SPLINE_CURVE_WITH_KNOTS ( ( 3, 2, 2, 2, 3 ),
 ( 0.3359374999999999445, 0.3385416666666666852, 0.3437500000000000000, 0.3489583333333333148, 0.3515625000000000000 ),
 .UNSPECIFIED. ) 
 CURVE ( )  GEOMETRIC_REPRESENTATION_ITEM ( )  RATIONAL_B_SPLINE_CURVE ( ( 0.9330127018922192983, 0.9330127018922178550, 1.000000000000000000, 0.8660254037844387076, 1.000000000000000000, 0.8660254037844387076, 1.000000000000000000, 0.9330127018922194093, 0.9330127018922194093 ) ) 
 REPRESENTATION_ITEM ( '' )  );
#6366=CARTESIAN_POINT ( 'NONE',  ( -61.99999999999999289, 12.64062499965860198, 0.5015494609379544944 ) ) ;
#6367=CARTESIAN_POINT ( 'NONE',  ( -61.13531646874998415, 8.348958332991935904, 1.000774730468978468 ) ) ;
#6369=CARTESIAN_POINT ( 'NONE',  ( -61.73205080756886076, 11.80133545031536890, 0.5000000000000014433 ) ) ;
#6370=EDGE_LOOP ( 'NONE', ( #6777, #5853, #9481, #3325 ) ) ;
#6371=CARTESIAN_POINT ( 'NONE',  ( -62.99999999999998579, 12.35416666666666785, 0.9226497308103756012 ) ) ;
#6372=CARTESIAN_POINT ( 'NONE',  ( -62.26794919243110371, 8.645085449632569308, 2.500000000000000888 ) ) ;
#6373=FACE_OUTER_BOUND ( 'NONE', #6664, .T. ) ;
#6374=ADVANCED_FACE ( 'NONE', ( #9262 ), #10871, .T. ) ;
#6376=CARTESIAN_POINT ( 'NONE',  ( -62.99999999999998579, 10.32291666598387003, 0.9226497308103756012 ) ) ;
#6381=CARTESIAN_POINT ( 'NONE',  ( -62.86468353124999453, 12.20312499965860198, 1.500000000000002220 ) ) ;
#6385=VERTEX_POINT ( 'NONE', #5133 ) ;
#6387=CARTESIAN_POINT ( 'NONE',  ( -62.43234176562499016, 9.807291666325268054, 2.248837904296538071 ) ) ;
#6390=CARTESIAN_POINT ( 'NONE',  ( -62.86468353124998742, 15.78645833299193590, 1.999225269531025972 ) ) ;
#6393=FACE_OUTER_BOUND ( 'NONE', #319, .T. ) ;
#6397=CARTESIAN_POINT ( 'NONE',  ( -61.99999999999998579, 9.812500000000000000, 0.3452994616207497591 ) ) ;
#6399=CARTESIAN_POINT ( 'NONE',  ( -60.99999999999998579, 11.27083333333333393, 0.9226497308103762673 ) ) ;
#6400=CARTESIAN_POINT ( 'NONE',  ( -61.49999999999998579, 11.95833333333333215, 2.366025403784441927 ) ) ;
#6401=CARTESIAN_POINT ( 'NONE',  ( -61.99999999999998579, 16.00000000000000000, 1.500000000000002220 ) ) ;
#6402=CARTESIAN_POINT ( 'NONE',  ( -61.56765823437498852, 10.53645833299193413, 2.248837904296538515 ) ) ;
#6404=CARTESIAN_POINT ( 'NONE',  ( -61.99999999999998579, 15.90624999931719863, 2.500000000000002665 ) ) ;
#6405=CARTESIAN_POINT ( 'NONE',  ( -62.86468353124999453, 12.01562499965860198, 1.500000000000002220 ) ) ;
#6407=ORIENTED_EDGE ( 'NONE', *, *, #8312, .F. ) ;
#6411=DIRECTION ( 'NONE',  ( -0.000000000000000000, -1.000000000000000000, -0.000000000000000000 ) ) ;
#6414=CARTESIAN_POINT ( 'NONE',  ( -61.73205080756886076, 10.27008544963257286, 0.5000000000000014433 ) ) ;
#6415=CARTESIAN_POINT ( 'NONE',  ( -61.99999999999998579, 14.51562499965860020, 2.498450539062049724 ) ) ;
#6416=CARTESIAN_POINT ( 'NONE',  ( -61.13531646874997705, 10.80729166632526628, 1.999225269531026417 ) ) ;
#6417=CARTESIAN_POINT ( 'NONE',  ( -62.99999999999998579, 8.645833333333333925, 2.077350269189627952 ) ) ;
#6419=CARTESIAN_POINT ( 'NONE',  ( -61.99999999999998579, 16.00000000000000000, 0.5000000000000041078 ) ) ;
#6420=CARTESIAN_POINT ( 'NONE',  ( -61.13531646874997705, 10.91145833299193413, 1.000774730468978468 ) ) ;
#6422=CARTESIAN_POINT ( 'NONE',  ( -60.99999999999998579, 16.21874999931720396, 1.500000000000002220 ) ) ;
#6424=CARTESIAN_POINT ( 'NONE',  ( -62.49999999999998579, 14.80208333265053611, 0.6339745962155627357 ) ) ;
#6425=CARTESIAN_POINT ( 'NONE',  ( -61.99999999999998579, 16.00000000000000000, 1.500000000000002220 ) ) ;
#6427=DIRECTION ( 'NONE',  ( -0.000000000000000000, -1.000000000000000000, -0.000000000000000000 ) ) ;
#6430=CARTESIAN_POINT ( 'NONE',  ( -61.13531646874997705, 12.55729166632526805, 1.999225269531026417 ) ) ;
#6431=CARTESIAN_POINT ( 'NONE',  ( -61.99999999999998579, 9.140624999658601979, 0.5015494609379544944 ) ) ;
#6432=CARTESIAN_POINT ( 'NONE',  ( -61.99999999999997868, 8.437500000000000000, 2.500000000000002665 ) ) ;
#6433=VERTEX_POINT ( 'NONE', #8376 ) ;
#6434=CARTESIAN_POINT ( 'NONE',  ( -62.99999999999998579, 12.37500000000000000, 1.500000000000001998 ) ) ;
#6435=FACE_OUTER_BOUND ( 'NONE', #7943, .T. ) ;
#6436=CYLINDRICAL_SURFACE ( 'NONE', #2462, 0.9999999999999981126 ) ;
#6437=CARTESIAN_POINT ( 'NONE',  ( -61.99999999999998579, 11.03124999931720218, 0.3452994616207497591 ) ) ;
#6438=ORIENTED_EDGE ( 'NONE', *, *, #3516, .T. ) ;
#6439=( BOUNDED_CURVE ( )  B_SPLINE_CURVE ( 2, ( #10389, #890, #10165, #9391, #6953, #5158, #6061, #1786, #2679 ),
 .UNSPECIFIED., .F., .F. ) 
 B_SPLINE_CURVE_WITH_KNOTS ( ( 3, 2, 2, 2, 3 ),
 ( 0.9296875000000000000, 0.9322916666666666297, 0.9375000000000000000, 0.9427083333333333703, 0.9453125000000000000 ),
 .UNSPECIFIED. ) 
 CURVE ( )  GEOMETRIC_REPRESENTATION_ITEM ( )  RATIONAL_B_SPLINE_CURVE ( ( 0.9330127018922194093, 0.9330127018922194093, 1.000000000000000000, 0.8660254037844387076, 1.000000000000000000, 0.8660254037844387076, 1.000000000000000000, 0.9330127018922194093, 0.9330127018922194093 ) ) 
 REPRESENTATION_ITEM ( '' )  );
#6440=ADVANCED_BREP_SHAPE_REPRESENTATION ( '', ( #8688, #2307 ), #9766 ) ;
#6441=DIRECTION ( 'NONE',  ( 0.000000000000000000, 1.000000000000000000, 0.000000000000000000 ) ) ;
#6442=CARTESIAN_POINT ( 'NONE',  ( -61.13531646874998415, 12.84895833299193413, 1.000774730468978468 ) ) ;
#6449=CARTESIAN_POINT ( 'NONE',  ( -62.43234176562498305, 11.22395833299193590, 0.7511620957034662593 ) ) ;
#6455=AXIS2_PLACEMENT_3D ( 'NONE', #2696, #7925, #6027 ) ;
#6456=EDGE_LOOP ( 'NONE', ( #101, #10947, #4297, #2551, #10659, #1019 ) ) ;
#6457=CARTESIAN_POINT ( 'NONE',  ( -60.99999999999998579, 9.447916665983871809, 2.077350269189628840 ) ) ;
#6458=CARTESIAN_POINT ( 'NONE',  ( -62.99999999999998579, 10.37500000000000000, 1.500000000000001998 ) ) ;
#6460=CARTESIAN_POINT ( 'NONE',  ( -60.99999999999998579, 12.22916666666666607, 2.077350269189628840 ) ) ;
#6462=CARTESIAN_POINT ( 'NONE',  ( -61.99999999999998579, 8.531249999317203958, 0.3452994616207497591 ) ) ;
#6464=CARTESIAN_POINT ( 'NONE',  ( -61.13531646874998415, 12.41145833299193413, 1.000774730468978468 ) ) ;
#6468=CARTESIAN_POINT ( 'NONE',  ( -62.26794919243111082, 9.176335450315367126, 2.500000000000000888 ) ) ;
#6469=VECTOR ( 'NONE', #8838, 1000.000000000000000 ) ;
#6472=CARTESIAN_POINT ( 'NONE',  ( -61.99999999999998579, 13.89062499965860198, 0.5015494609379544944 ) ) ;
#6473=CARTESIAN_POINT ( 'NONE',  ( -62.43234176562498305, 9.911458332991934128, 0.7511620957034662593 ) ) ;
#6474=CARTESIAN_POINT ( 'NONE',  ( -61.49999999999998579, 11.67708333265053611, 2.366025403784441927 ) ) ;
#6477=CARTESIAN_POINT ( 'NONE',  ( -61.13531646874998415, 11.89062499965860198, 1.500000000000002220 ) ) ;
#6479=CARTESIAN_POINT ( 'NONE',  ( -61.99999999999998579, 16.00000000000000000, 2.500000000000000444 ) ) ;
#6480=CARTESIAN_POINT ( 'NONE',  ( -61.56765823437498852, 8.348958332991934128, 2.248837904296538515 ) ) ;
#6483=CARTESIAN_POINT ( 'NONE',  ( -61.99999999999998579, 15.15624999931720218, 2.500000000000002665 ) ) ;
#6484=ORIENTED_EDGE ( 'NONE', *, *, #535, .T. ) ;
#6485=CARTESIAN_POINT ( 'NONE',  ( -62.43234176562498305, 13.16145833299193413, 0.7511620957034662593 ) ) ;
#6486=EDGE_CURVE ( 'NONE', #10295, #4413, #6778, .T. ) ;
#6487=CARTESIAN_POINT ( 'NONE',  ( -62.86468353124999453, 9.703124999658601979, 1.500000000000002220 ) ) ;
#6490=CARTESIAN_POINT ( 'NONE',  ( -60.99999999999998579, 13.72916666666666785, 2.077350269189628840 ) ) ;
#6493=CARTESIAN_POINT ( 'NONE',  ( -60.99999999999998579, 11.69791666598386826, 2.077350269189628840 ) ) ;
#6496=CARTESIAN_POINT ( 'NONE',  ( -61.13531646874998415, 12.82812499965860198, 1.500000000000002220 ) ) ;
#6499=CARTESIAN_POINT ( 'NONE',  ( -61.99999999999998579, 11.95312499965860198, 0.5015494609379544944 ) ) ;
#6501=CARTESIAN_POINT ( 'NONE',  ( -62.86468353124998742, 15.28645833299193413, 1.999225269531025972 ) ) ;
#6502=VERTEX_POINT ( 'NONE', #8594 ) ;
#6505=ORIENTED_EDGE ( 'NONE', *, *, #1848, .T. ) ;
#6507=CARTESIAN_POINT ( 'NONE',  ( -62.99999999999998579, 10.10416666666666785, 0.9226497308103756012 ) ) ;
#6509=CARTESIAN_POINT ( 'NONE',  ( -61.99999999999998579, 16.00000000000000000, 1.500000000000002220 ) ) ;
#6510=CARTESIAN_POINT ( 'NONE',  ( -61.99999999999998579, 16.00000000000000000, 1.500000000000002220 ) ) ;
#6512=CARTESIAN_POINT ( 'NONE',  ( -62.99999999999998579, 15.86458333265053788, 2.077350269189627952 ) ) ;
#6513=CARTESIAN_POINT ( 'NONE',  ( -62.86468353124998742, 11.53645833299193413, 1.999225269531025972 ) ) ;
#6515=EDGE_LOOP ( 'NONE', ( #6125, #1300, #3486, #7185 ) ) ;
#6519=FACE_OUTER_BOUND ( 'NONE', #2031, .T. ) ;
#6520=EDGE_CURVE ( 'NONE', #6385, #7083, #10475, .T. ) ;
#6521=CARTESIAN_POINT ( 'NONE',  ( -61.13531646874998415, 13.57812499965860198, 1.500000000000002220 ) ) ;
#6522=CARTESIAN_POINT ( 'NONE',  ( -62.43234176562498305, 10.41145833299193413, 0.7511620957034662593 ) ) ;
#6525=DIRECTION ( 'NONE',  ( -0.000000000000000000, -1.000000000000000000, -0.000000000000000000 ) ) ;
#6526=CARTESIAN_POINT ( 'NONE',  ( -61.99999999999999289, 11.45312499965860020, 0.5015494609379544944 ) ) ;
#6527=CARTESIAN_POINT ( 'NONE',  ( -62.43234176562498305, 14.97395833299193590, 0.7511620957034662593 ) ) ;
#6530=CARTESIAN_POINT ( 'NONE',  ( -62.26794919243111082, 15.17633545031537246, 2.500000000000003109 ) ) ;
#6531=CARTESIAN_POINT ( 'NONE',  ( -60.99999999999998579, 15.94791666598386826, 2.077350269189628840 ) ) ;
#6536=CARTESIAN_POINT ( 'NONE',  ( -61.13531646874998415, 14.32812499965860020, 1.500000000000002220 ) ) ;
#6537=CARTESIAN_POINT ( 'NONE',  ( -62.43234176562498305, 10.16145833299193413, 0.7511620957034662593 ) ) ;
#6539=LINE ( 'NONE', #5796, #8723 ) ;
#6541=CARTESIAN_POINT ( 'NONE',  ( -62.49999999999998579, 13.33333333333333215, 0.6339745962155627357 ) ) ;
#6543=CARTESIAN_POINT ( 'NONE',  ( -61.49999999999998579, 8.958333333333333925, 2.366025403784441927 ) ) ;
#6544=CARTESIAN_POINT ( 'NONE',  ( -61.49999999999998579, 11.76041666598387003, 0.6339745962155628467 ) ) ;
#6546=CARTESIAN_POINT ( 'NONE',  ( -62.26794919243111082, 14.92633545031537068, 2.500000000000003109 ) ) ;
#6547=CARTESIAN_POINT ( 'NONE',  ( -61.13531646874998415, 13.34895833299193413, 1.000774730468978468 ) ) ;
#6548=DIRECTION ( 'NONE',  ( -0.000000000000000000, -1.000000000000000000, -0.000000000000000000 ) ) ;
#6553=CARTESIAN_POINT ( 'NONE',  ( -61.13531646874998415, 11.89062499965860198, 1.500000000000002220 ) ) ;
#6554=CARTESIAN_POINT ( 'NONE',  ( -61.49999999999998579, 12.26041666598386826, 0.6339745962155628467 ) ) ;
#6555=AXIS2_PLACEMENT_3D ( 'NONE', #2380, #9163, #9891 ) ;
#6561=( BOUNDED_CURVE ( )  B_SPLINE_CURVE ( 2, ( #1189, #3861, #5457, #4631, #9749, #2146, #7143, #8923, #1367 ),
 .UNSPECIFIED., .F., .T. ) 
 B_SPLINE_CURVE_WITH_KNOTS ( ( 3, 2, 2, 2, 3 ),
 ( 0.8046875000000000000, 0.8072916666666666297, 0.8125000000000000000, 0.8177083333333333703, 0.8203125000000000000 ),
 .UNSPECIFIED. ) 
 CURVE ( )  GEOMETRIC_REPRESENTATION_ITEM ( )  RATIONAL_B_SPLINE_CURVE ( ( 0.9330127018922194093, 0.9330127018922194093, 1.000000000000000000, 0.8660254037844387076, 1.000000000000000000, 0.8660254037844387076, 1.000000000000000000, 0.9330127018922194093, 0.9330127018922194093 ) ) 
 REPRESENTATION_ITEM ( '' )  );
#6564=CARTESIAN_POINT ( 'NONE',  ( -61.99999999999998579, 9.687499999999998224, 2.654700538379254571 ) ) ;
#6566=CARTESIAN_POINT ( 'NONE',  ( -60.99999999999998579, 14.94791666598386826, 2.077350269189628840 ) ) ;
#6567=CARTESIAN_POINT ( 'NONE',  ( -60.99999999999998579, 12.25000000000000000, 1.500000000000002220 ) ) ;
#6569=CARTESIAN_POINT ( 'NONE',  ( -62.99999999999998579, 15.82291666598386826, 0.9226497308103756012 ) ) ;
#6570=CARTESIAN_POINT ( 'NONE',  ( -62.86468353124999453, 12.26562499965860198, 1.500000000000002220 ) ) ;
#6572=CARTESIAN_POINT ( 'NONE',  ( -62.49999999999998579, 14.55208333265053611, 0.6339745962155627357 ) ) ;
#6575=VECTOR ( 'NONE', #1160, 1000.000000000000000 ) ;
#6579=CARTESIAN_POINT ( 'NONE',  ( -61.99999999999998579, 13.51562499965860198, 2.498450539062049724 ) ) ;
#6581=( GEOMETRIC_REPRESENTATION_CONTEXT ( 3 ) GLOBAL_UNCERTAINTY_ASSIGNED_CONTEXT ( ( #2363 ) ) GLOBAL_UNIT_ASSIGNED_CONTEXT ( ( #1638, #3349, #2362 ) ) REPRESENTATION_CONTEXT ( 'NONE', 'WORKASPACE' ) );
#6584=CARTESIAN_POINT ( 'NONE',  ( -62.86468353124999453, 11.78645833299193590, 1.999225269531025750 ) ) ;
#6585=CARTESIAN_POINT ( 'NONE',  ( -62.86468353124999453, 15.76562499965860198, 1.500000000000002220 ) ) ;
#6587=LINE ( 'NONE', #6479, #1581 ) ;
#6588=CARTESIAN_POINT ( 'NONE',  ( -61.49999999999998579, 15.67708333265053611, 2.366025403784441927 ) ) ;
#6591=LINE ( 'NONE', #9082, #867 ) ;
#6592=DIRECTION ( 'NONE',  ( -0.000000000000000000, -1.000000000000000000, -0.000000000000000000 ) ) ;
#6593=CARTESIAN_POINT ( 'NONE',  ( -62.86468353124999453, 13.70312499965860198, 1.500000000000002220 ) ) ;
#6594=CARTESIAN_POINT ( 'NONE',  ( -62.43234176562499016, 10.49479166632526983, 2.248837904296538071 ) ) ;
#6597=CARTESIAN_POINT ( 'NONE',  ( -62.49999999999998579, 14.16666666666666785, 2.366025403784441483 ) ) ;
#6601=CARTESIAN_POINT ( 'NONE',  ( -60.99999999999998579, 12.46874999931720396, 1.500000000000002220 ) ) ;
#6603=CARTESIAN_POINT ( 'NONE',  ( -61.49999999999998579, 9.541666666666667851, 0.6339745962155628467 ) ) ;
#6604=CARTESIAN_POINT ( 'NONE',  ( -61.99999999999998579, 14.51562499965860020, 2.498450539062049724 ) ) ;
#6607=CARTESIAN_POINT ( 'NONE',  ( -61.56765823437498852, 12.09895833299193413, 2.248837904296538515 ) ) ;
#6610=CARTESIAN_POINT ( 'NONE',  ( -62.86468353124998032, 15.99479166632526805, 1.000774730468978246 ) ) ;
#6611=ORIENTED_EDGE ( 'NONE', *, *, #6486, .T. ) ;
#6613=CARTESIAN_POINT ( 'NONE',  ( -62.49999999999998579, 11.08333333333333393, 0.6339745962155627357 ) ) ;
#6615=ORIENTED_EDGE ( 'NONE', *, *, #479, .F. ) ;
#6616=CARTESIAN_POINT ( 'NONE',  ( -61.99999999999998579, 9.406249999317202182, 2.500000000000002665 ) ) ;
#6617=CARTESIAN_POINT ( 'NONE',  ( -60.99999999999998579, 9.979166666666667851, 2.077350269189628840 ) ) ;
#6618=LINE ( 'NONE', #3063, #2996 ) ;
#6619=CYLINDRICAL_SURFACE ( 'NONE', #6555, 0.9999999999999981126 ) ;
#6620=CARTESIAN_POINT ( 'NONE',  ( -60.99999999999998579, 8.239583332650536107, 0.9226497308103762673 ) ) ;
#6621=CARTESIAN_POINT ( 'NONE',  ( -61.56765823437498852, 11.84895833299193413, 2.248837904296538515 ) ) ;
#6622=CARTESIAN_POINT ( 'NONE',  ( -62.99999999999998579, 10.60416666666666607, 0.9226497308103756012 ) ) ;
#6626=VERTEX_POINT ( 'NONE', #7935 ) ;
#6628=CARTESIAN_POINT ( 'NONE',  ( -60.99999999999998579, 13.69791666598387003, 2.077350269189628840 ) ) ;
#6629=CARTESIAN_POINT ( 'NONE',  ( -61.99999999999998579, 14.01562499965860376, 2.498450539062049724 ) ) ;
#6631=CARTESIAN_POINT ( 'NONE',  ( -61.73205080756886076, 11.77008544963257286, 0.5000000000000014433 ) ) ;
#6633=CARTESIAN_POINT ( 'NONE',  ( -61.13531646874997705, 12.86979166632526983, 1.999225269531026417 ) ) ;
#6634=CARTESIAN_POINT ( 'NONE',  ( -61.56765823437498142, 15.93229166632526628, 0.7511620957034663704 ) ) ;
#6635=CARTESIAN_POINT ( 'NONE',  ( -61.99999999999998579, 15.06249999999999822, 0.5000000000000013323 ) ) ;
#6637=DIRECTION ( 'NONE',  ( 0.000000000000000000, 0.000000000000000000, -1.000000000000000000 ) ) ;
#6638=CARTESIAN_POINT ( 'NONE',  ( -60.99999999999998579, 15.96874999931720218, 1.500000000000002220 ) ) ;
#6644=ADVANCED_FACE ( 'NONE', ( #7101 ), #5417, .T. ) ;
#6645=CARTESIAN_POINT ( 'NONE',  ( -61.56765823437498852, 13.78645833299193413, 2.248837904296538515 ) ) ;
#6646=CARTESIAN_POINT ( 'NONE',  ( -62.43234176562498305, 9.661458332991934128, 0.7511620957034662593 ) ) ;
#6647=CARTESIAN_POINT ( 'NONE',  ( -62.43234176562498305, 15.72395833299193590, 0.7511620957034662593 ) ) ;
#6650=CARTESIAN_POINT ( 'NONE',  ( -60.99999999999998579, 13.47916666666666785, 2.077350269189628840 ) ) ;
#6651=CARTESIAN_POINT ( 'NONE',  ( -61.99999999999999289, 9.328124999658600203, 2.498450539062049724 ) ) ;
#6653=CARTESIAN_POINT ( 'NONE',  ( -61.49999999999998579, 11.51041666598387003, 0.6339745962155628467 ) ) ;
#6654=CARTESIAN_POINT ( 'NONE',  ( -61.56765823437498142, 14.61979166632526805, 0.7511620957034663704 ) ) ;
#6655=CARTESIAN_POINT ( 'NONE',  ( -62.26794919243111082, 15.57366454968462932, 0.5000000000000013323 ) ) ;
#6656=( BOUNDED_CURVE ( )  B_SPLINE_CURVE ( 2, ( #9193, #747, #797, #3193, #4175, #4903, #10956, #7477, #7368 ),
 .UNSPECIFIED., .F., .T. ) 
 B_SPLINE_CURVE_WITH_KNOTS ( ( 3, 2, 2, 2, 3 ),
 ( 0.7734375000000000000, 0.7760416666666666297, 0.7812500000000000000, 0.7864583333333333703, 0.7890625000000000000 ),
 .UNSPECIFIED. ) 
 CURVE ( )  GEOMETRIC_REPRESENTATION_ITEM ( )  RATIONAL_B_SPLINE_CURVE ( ( 0.9330127018922194093, 0.9330127018922194093, 1.000000000000000000, 0.8660254037844387076, 1.000000000000000000, 0.8660254037844387076, 1.000000000000000000, 0.9330127018922194093, 0.9330127018922194093 ) ) 
 REPRESENTATION_ITEM ( '' )  );
#6657=ORIENTED_EDGE ( 'NONE', *, *, #2324, .T. ) ;
#6659=CARTESIAN_POINT ( 'NONE',  ( -61.56765823437498142, 11.43229166632526805, 0.7511620957034663704 ) ) ;
#6660=CARTESIAN_POINT ( 'NONE',  ( -61.49999999999998579, 11.51041666598387003, 0.6339745962155628467 ) ) ;
#6663=CARTESIAN_POINT ( 'NONE',  ( -61.73205080756886076, 14.80133545031537068, 0.5000000000000014433 ) ) ;
#6664=EDGE_LOOP ( 'NONE', ( #1795, #5276, #7904, #5938 ) ) ;
#6666=CARTESIAN_POINT ( 'NONE',  ( -60.99999999999998579, 10.72916666666666607, 2.077350269189628840 ) ) ;
#6667=DIRECTION ( 'NONE',  ( 0.000000000000000000, 0.000000000000000000, -1.000000000000000000 ) ) ;
#6668=CARTESIAN_POINT ( 'NONE',  ( -62.26794919243111082, 15.92633545031536890, 2.500000000000003109 ) ) ;
#6669=CARTESIAN_POINT ( 'NONE',  ( -60.99999999999998579, 8.718749999317203958, 1.500000000000002220 ) ) ;
#6670=CARTESIAN_POINT ( 'NONE',  ( -62.86468353124999453, 13.01562499965860198, 1.500000000000002220 ) ) ;
#6671=CARTESIAN_POINT ( 'NONE',  ( -62.99999999999998579, 10.62499999999999822, 1.500000000000001998 ) ) ;
#6676=CARTESIAN_POINT ( 'NONE',  ( -61.56765823437498142, 15.11979166632526805, 0.7511620957034663704 ) ) ;
#6680=CARTESIAN_POINT ( 'NONE',  ( -62.43234176562498305, 12.72395833299193413, 0.7511620957034662593 ) ) ;
#6681=CARTESIAN_POINT ( 'NONE',  ( -61.13531646874998415, 16.11979166632526628, 1.999225269531026417 ) ) ;
#6682=FACE_OUTER_BOUND ( 'NONE', #3598, .T. ) ;
#6683=DIRECTION ( 'NONE',  ( 0.000000000000000000, 0.000000000000000000, -1.000000000000000000 ) ) ;
#6684=CARTESIAN_POINT ( 'NONE',  ( -61.99999999999998579, 15.53124999931720218, 0.3452994616207497591 ) ) ;
#6690=CARTESIAN_POINT ( 'NONE',  ( -61.13531646874997705, 13.80729166632526983, 1.999225269531026417 ) ) ;
#6691=CARTESIAN_POINT ( 'NONE',  ( -62.43234176562499016, 10.24479166632526805, 2.248837904296538071 ) ) ;
#6692=CARTESIAN_POINT ( 'NONE',  ( -62.43234176562499016, 15.30729166632526805, 2.248837904296538071 ) ) ;
#6694=ORIENTED_EDGE ( 'NONE', *, *, #10652, .T. ) ;
#6695=CARTESIAN_POINT ( 'NONE',  ( -61.99999999999998579, 13.68750000000000178, 2.654700538379254571 ) ) ;
#6698=CARTESIAN_POINT ( 'NONE',  ( -61.99999999999998579, 12.28124999931720396, 0.3452994616207497591 ) ) ;
#6701=CARTESIAN_POINT ( 'NONE',  ( -61.13531646874998415, 13.84895833299193413, 1.000774730468978468 ) ) ;
#6705=CARTESIAN_POINT ( 'NONE',  ( -61.99999999999998579, 13.45312499965860376, 0.5015494609379544944 ) ) ;
#6712=( BOUNDED_CURVE ( )  B_SPLINE_CURVE ( 2, ( #7393, #9890, #1603, #1547, #2229, #768, #662, #3211, #4876 ),
 .UNSPECIFIED., .F., .T. ) 
 B_SPLINE_CURVE_WITH_KNOTS ( ( 3, 2, 2, 2, 3 ),
 ( 0.05468749999999997918, 0.05729166666666666435, 0.06250000000000000000, 0.06770833333333332871, 0.07031249999999995837 ),
 .UNSPECIFIED. ) 
 CURVE ( )  GEOMETRIC_REPRESENTATION_ITEM ( )  RATIONAL_B_SPLINE_CURVE ( ( 0.9330127018922192983, 0.9330127018922187432, 1.000000000000000000, 0.8660254037844387076, 1.000000000000000000, 0.8660254037844387076, 1.000000000000000000, 0.9330127018922204085, 0.9330127018922194093 ) ) 
 REPRESENTATION_ITEM ( '' )  );
#6714=CARTESIAN_POINT ( 'NONE',  ( -61.99999999999998579, 11.18749999999999822, 2.654700538379254571 ) ) ;
#6715=ORIENTED_EDGE ( 'NONE', *, *, #6520, .T. ) ;
#6717=CARTESIAN_POINT ( 'NONE',  ( -61.99999999999998579, 8.453124999658601979, 0.5015494609379544944 ) ) ;
#6718=CARTESIAN_POINT ( 'NONE',  ( -60.99999999999998579, 10.48958333265053611, 0.9226497308103762673 ) ) ;
#6719=AXIS2_PLACEMENT_3D ( 'NONE', #9861, #8974, #6637 ) ;
#6720=CARTESIAN_POINT ( 'NONE',  ( -62.43234176562498305, 13.22395833299193413, 0.7511620957034662593 ) ) ;
#6721=CARTESIAN_POINT ( 'NONE',  ( -62.49999999999998579, 12.88541666598386826, 2.366025403784441483 ) ) ;
#6723=CARTESIAN_POINT ( 'NONE',  ( -61.99999999999998579, 11.03124999931720218, 0.5000000000000013323 ) ) ;
#6725=AXIS2_PLACEMENT_3D ( 'NONE', #3758, #6204, #2815 ) ;
#6727=CARTESIAN_POINT ( 'NONE',  ( -61.99999999999998579, 12.81250000000000000, 0.5000000000000013323 ) ) ;
#6728=CARTESIAN_POINT ( 'NONE',  ( -62.86468353124999453, 15.70312499965860198, 1.500000000000002220 ) ) ;
#6730=CARTESIAN_POINT ( 'NONE',  ( -61.99999999999998579, 13.68749999999999822, 2.500000000000002665 ) ) ;
#6731=CARTESIAN_POINT ( 'NONE',  ( -61.99999999999998579, 8.062500000000000000, 0.5000000000000013323 ) ) ;
#6733=CARTESIAN_POINT ( 'NONE',  ( -62.86468353124999453, 12.78645833299193413, 1.999225269531025750 ) ) ;
#6734=CARTESIAN_POINT ( 'NONE',  ( -62.86468353124998742, 15.03645833299193590, 1.999225269531025972 ) ) ;
#6735=FACE_OUTER_BOUND ( 'NONE', #1682, .T. ) ;
#6736=CARTESIAN_POINT ( 'NONE',  ( -60.99999999999998579, 13.46874999931720218, 1.500000000000002220 ) ) ;
#6737=CARTESIAN_POINT ( 'NONE',  ( -62.43234176562499016, 8.807291666325268054, 2.248837904296538071 ) ) ;
#6738=CARTESIAN_POINT ( 'NONE',  ( -62.49999999999998579, 10.41666666666666785, 2.366025403784441483 ) ) ;
#6740=DIRECTION ( 'NONE',  ( -0.000000000000000000, -1.000000000000000000, -0.000000000000000000 ) ) ;
#6741=CARTESIAN_POINT ( 'NONE',  ( -61.73205080756885366, 8.051335450315370679, 0.5000000000000027756 ) ) ;
#6744=CARTESIAN_POINT ( 'NONE',  ( -62.43234176562498305, 15.66145833299193590, 0.7511620957034662593 ) ) ;
#6745=CARTESIAN_POINT ( 'NONE',  ( -61.56765823437498852, 11.78645833299193413, 2.248837904296538515 ) ) ;
#6746=CARTESIAN_POINT ( 'NONE',  ( -61.99999999999999289, 15.95312499965860198, 0.5015494609379544944 ) ) ;
#6748=ORIENTED_EDGE ( 'NONE', *, *, #3428, .T. ) ;
#6749=CARTESIAN_POINT ( 'NONE',  ( -60.99999999999998579, 15.25000000000000000, 1.500000000000002220 ) ) ;
#6750=EDGE_CURVE ( 'NONE', #7755, #8746, #10105, .T. ) ;
#6751=CARTESIAN_POINT ( 'NONE',  ( -62.86468353124998032, 8.244791666325268054, 1.000774730468978024 ) ) ;
#6753=CARTESIAN_POINT ( 'NONE',  ( -62.99999999999998579, 13.61458333265053611, 2.077350269189627952 ) ) ;
#6754=VERTEX_POINT ( 'NONE', #3186 ) ;
#6755=DIRECTION ( 'NONE',  ( -0.000000000000000000, -1.000000000000000000, -0.000000000000000000 ) ) ;
#6756=CARTESIAN_POINT ( 'NONE',  ( -61.99999999999998579, 13.39062499965860020, 0.5015494609379544944 ) ) ;
#6757=DIRECTION ( 'NONE',  ( 0.000000000000000000, 0.000000000000000000, -1.000000000000000000 ) ) ;
#6760=CARTESIAN_POINT ( 'NONE',  ( -62.86468353124998032, 12.49479166632526628, 1.000774730468978246 ) ) ;
#6761=CARTESIAN_POINT ( 'NONE',  ( -61.99999999999998579, 16.00000000000000000, 0.5000000000000041078 ) ) ;
#6762=ORIENTED_EDGE ( 'NONE', *, *, #2096, .F. ) ;
#6765=CYLINDRICAL_SURFACE ( 'NONE', #1434, 0.9999999999999981126 ) ;
#6766=EDGE_CURVE ( 'NONE', #7998, #1879, #6591, .T. ) ;
#6769=CIRCLE ( 'NONE', #1114, 0.9999999999999983347 ) ;
#6770=CARTESIAN_POINT ( 'NONE',  ( -61.99999999999998579, 11.68750000000000000, 2.654700538379254571 ) ) ;
#6771=APPLICATION_CONTEXT ( 'automotive_design' ) ;
#6773=CARTESIAN_POINT ( 'NONE',  ( -62.43234176562499016, 9.557291666325268054, 2.248837904296538071 ) ) ;
#6775=CARTESIAN_POINT ( 'NONE',  ( -61.56765823437498142, 12.68229166632526805, 0.7511620957034663704 ) ) ;
#6776=CARTESIAN_POINT ( 'NONE',  ( -61.99999999999998579, 10.56249999999999822, 0.5000000000000013323 ) ) ;
#6777=ORIENTED_EDGE ( 'NONE', *, *, #8053, .F. ) ;
#6778=( BOUNDED_CURVE ( )  B_SPLINE_CURVE ( 2, ( #5187, #9533, #1985, #10481, #10365, #6986, #260, #6208, #6035 ),
 .UNSPECIFIED., .F., .T. ) 
 B_SPLINE_CURVE_WITH_KNOTS ( ( 3, 2, 2, 2, 3 ),
 ( 0.6796875000000000000, 0.6822916666666666297, 0.6875000000000000000, 0.6927083333333333703, 0.6953125000000000000 ),
 .UNSPECIFIED. ) 
 CURVE ( )  GEOMETRIC_REPRESENTATION_ITEM ( )  RATIONAL_B_SPLINE_CURVE ( ( 0.9330127018922194093, 0.9330127018922194093, 1.000000000000000000, 0.8660254037844387076, 1.000000000000000000, 0.8660254037844387076, 1.000000000000000000, 0.9330127018922194093, 0.9330127018922194093 ) ) 
 REPRESENTATION_ITEM ( '' )  );
#6781=ORIENTED_EDGE ( 'NONE', *, *, #10973, .T. ) ;
#6782=CARTESIAN_POINT ( 'NONE',  ( -60.99999999999998579, 14.23958333265053611, 0.9226497308103762673 ) ) ;
#6783=CARTESIAN_POINT ( 'NONE',  ( -62.86468353124998742, 15.47395833299193413, 1.999225269531025972 ) ) ;
#6786=CARTESIAN_POINT ( 'NONE',  ( -61.99999999999998579, 8.812500000000000000, 0.5000000000000013323 ) ) ;
#6788=CARTESIAN_POINT ( 'NONE',  ( -61.56765823437498852, 12.09895833299193413, 2.248837904296538515 ) ) ;
#6789=EDGE_CURVE ( 'NONE', #7083, #8021, #8409, .T. ) ;
#6790=AXIS2_PLACEMENT_3D ( 'NONE', #2838, #5375, #8782 ) ;
#6791=CARTESIAN_POINT ( 'NONE',  ( -62.86468353124999453, 8.953124999658601979, 1.500000000000002220 ) ) ;
#6792=DIRECTION ( 'NONE',  ( -0.000000000000000000, -1.000000000000000000, -0.000000000000000000 ) ) ;
#6793=CARTESIAN_POINT ( 'NONE',  ( -61.99999999999998579, 13.40624999931720041, 2.500000000000002665 ) ) ;
#6794=CARTESIAN_POINT ( 'NONE',  ( -61.99999999999998579, 9.703124999658601979, 0.5015494609379544944 ) ) ;
#6799=VECTOR ( 'NONE', #4639, 1000.000000000000000 ) ;
#6800=CARTESIAN_POINT ( 'NONE',  ( -61.99999999999999289, 15.76562499965860198, 2.498450539062049724 ) ) ;
#6801=CARTESIAN_POINT ( 'NONE',  ( -62.43234176562498305, 11.41145833299193590, 0.7511620957034662593 ) ) ;
#6802=CARTESIAN_POINT ( 'NONE',  ( -61.13531646874997705, 15.91145833299193590, 1.000774730468978468 ) ) ;
#6805=CARTESIAN_POINT ( 'NONE',  ( -60.99999999999998579, 15.47916666666666430, 2.077350269189628840 ) ) ;
#6806=CARTESIAN_POINT ( 'NONE',  ( -61.13531646874998415, 8.640624999658601979, 1.500000000000002220 ) ) ;
#6808=CARTESIAN_POINT ( 'NONE',  ( -61.49999999999998579, 13.26041666598387003, 0.6339745962155628467 ) ) ;
#6810=VERTEX_POINT ( 'NONE', #2938 ) ;
#6814=CARTESIAN_POINT ( 'NONE',  ( -62.86468353124999453, 11.72395833299193413, 1.999225269531025750 ) ) ;
#6817=CARTESIAN_POINT ( 'NONE',  ( -62.43234176562499016, 13.55729166632526805, 2.248837904296538071 ) ) ;
#6818=CARTESIAN_POINT ( 'NONE',  ( -61.99999999999998579, 16.00000000000000000, 0.5000000000000041078 ) ) ;
#6819=EDGE_LOOP ( 'NONE', ( #1488, #157, #8970, #1871 ) ) ;
#6824=CARTESIAN_POINT ( 'NONE',  ( -61.13531646874998415, 11.80729166632526805, 1.999225269531026417 ) ) ;
#6826=CARTESIAN_POINT ( 'NONE',  ( -61.13531646874998415, 8.640624999658601979, 1.500000000000002220 ) ) ;
#6827=CARTESIAN_POINT ( 'NONE',  ( -62.26794919243111082, 13.89508544963257108, 2.500000000000003109 ) ) ;
#6828=CARTESIAN_POINT ( 'NONE',  ( -61.56765823437498142, 13.68229166632526805, 0.7511620957034663704 ) ) ;
#6830=ORIENTED_EDGE ( 'NONE', *, *, #1892, .F. ) ;
#6831=CARTESIAN_POINT ( 'NONE',  ( -62.26794919243111082, 9.323664549684631098, 0.4999999999999998890 ) ) ;
#6832=EDGE_LOOP ( 'NONE', ( #775, #2588, #8604, #2276 ) ) ;
#6833=CARTESIAN_POINT ( 'NONE',  ( -61.99999999999998579, 12.68750000000000000, 2.500000000000002665 ) ) ;
#6834=CARTESIAN_POINT ( 'NONE',  ( -61.13531646874998415, 14.82812499965860020, 1.500000000000002220 ) ) ;
#6836=CARTESIAN_POINT ( 'NONE',  ( -61.49999999999998579, 12.45833333333333393, 2.366025403784441927 ) ) ;
#6837=CARTESIAN_POINT ( 'NONE',  ( -62.26794919243111082, 12.39508544963257286, 2.500000000000003109 ) ) ;
#6838=CARTESIAN_POINT ( 'NONE',  ( -62.86468353124999453, 12.76562499965860198, 1.500000000000002220 ) ) ;
#6839=CARTESIAN_POINT ( 'NONE',  ( -62.86468353124998742, 8.473958332991934128, 1.999225269531025972 ) ) ;
#6840=CARTESIAN_POINT ( 'NONE',  ( -61.99999999999998579, 16.00000000000000000, 1.500000000000002220 ) ) ;
#6842=CARTESIAN_POINT ( 'NONE',  ( -62.43234176562499016, 9.807291666325268054, 2.248837904296538071 ) ) ;
#6844=FACE_OUTER_BOUND ( 'NONE', #8383, .T. ) ;
#6845=ORIENTED_EDGE ( 'NONE', *, *, #7319, .T. ) ;
#6847=DIRECTION ( 'NONE',  ( 0.000000000000000000, 0.000000000000000000, -1.000000000000000000 ) ) ;
#6849=CARTESIAN_POINT ( 'NONE',  ( -62.86468353124999453, 15.70312499965860198, 1.500000000000002220 ) ) ;
#6850=CARTESIAN_POINT ( 'NONE',  ( -62.86468353124998742, 11.22395833299193590, 1.999225269531025972 ) ) ;
#6851=CARTESIAN_POINT ( 'NONE',  ( -62.43234176562498305, 9.161458332991935904, 0.7511620957034662593 ) ) ;
#6853=ORIENTED_EDGE ( 'NONE', *, *, #7407, .F. ) ;
#6854=CARTESIAN_POINT ( 'NONE',  ( -61.99999999999998579, 14.68750000000000000, 2.654700538379254571 ) ) ;
#6855=CARTESIAN_POINT ( 'NONE',  ( -62.86468353124999453, 8.786458332991934128, 1.999225269531025750 ) ) ;
#6856=CARTESIAN_POINT ( 'NONE',  ( -60.99999999999998579, 13.73958333265053433, 0.9226497308103762673 ) ) ;
#6859=CARTESIAN_POINT ( 'NONE',  ( -61.99999999999998579, 11.56250000000000000, 0.5000000000000013323 ) ) ;
#6860=CARTESIAN_POINT ( 'NONE',  ( -61.99999999999999289, 11.76562499965860198, 2.498450539062049724 ) ) ;
#6862=CARTESIAN_POINT ( 'NONE',  ( -61.99999999999998579, 16.00000000000000000, 1.500000000000002220 ) ) ;
#6863=ORIENTED_EDGE ( 'NONE', *, *, #5076, .F. ) ;
#6865=CARTESIAN_POINT ( 'NONE',  ( -62.86468353124999453, 12.51562499965860198, 1.500000000000002220 ) ) ;
#6866=CARTESIAN_POINT ( 'NONE',  ( -61.99999999999998579, 13.81249999999999822, 0.5000000000000013323 ) ) ;
#6867=CARTESIAN_POINT ( 'NONE',  ( -61.49999999999998579, 9.260416665983870033, 0.6339745962155628467 ) ) ;
#6869=ORIENTED_EDGE ( 'NONE', *, *, #2316, .T. ) ;
#6871=VERTEX_POINT ( 'NONE', #65 ) ;
#6872=CARTESIAN_POINT ( 'NONE',  ( -62.99999999999998579, 12.35416666666666607, 0.9226497308103756012 ) ) ;
#6873=EDGE_CURVE ( 'NONE', #9265, #470, #5217, .T. ) ;
#6874=CARTESIAN_POINT ( 'NONE',  ( -62.86468353124998032, 11.43229166632526805, 1.000774730468978246 ) ) ;
#6875=VERTEX_POINT ( 'NONE', #3391 ) ;
#6876=CIRCLE ( 'NONE', #3678, 0.9999999999999983347 ) ;
#6877=CARTESIAN_POINT ( 'NONE',  ( -62.86468353124998032, 8.494791666325268054, 1.000774730468978246 ) ) ;
#6880=EDGE_CURVE ( 'NONE', #3615, #10979, #1788, .T. ) ;
#6881=CARTESIAN_POINT ( 'NONE',  ( -61.99999999999998579, 12.95312499965860198, 0.5015494609379544944 ) ) ;
#6882=CARTESIAN_POINT ( 'NONE',  ( -62.49999999999998579, 12.13541666598386826, 2.366025403784441483 ) ) ;
#6883=ORIENTED_EDGE ( 'NONE', *, *, #9294, .T. ) ;
#6888=ORIENTED_EDGE ( 'NONE', *, *, #2354, .T. ) ;
#6889=CARTESIAN_POINT ( 'NONE',  ( -62.99999999999998579, 10.85416666666666785, 0.9226497308103756012 ) ) ;
#6890=CARTESIAN_POINT ( 'NONE',  ( -62.43234176562498305, 14.91145833299193590, 0.7511620957034662593 ) ) ;
#6892=CARTESIAN_POINT ( 'NONE',  ( -60.99999999999998579, 12.46874999931720396, 1.500000000000002220 ) ) ;
#6893=CARTESIAN_POINT ( 'NONE',  ( -61.99999999999998579, 12.40624999931720218, 2.500000000000002665 ) ) ;
#6894=CARTESIAN_POINT ( 'NONE',  ( -62.43234176562498305, 14.72395833299193413, 0.7511620957034662593 ) ) ;
#6896=CARTESIAN_POINT ( 'NONE',  ( -62.86468353124999453, 9.203124999658600203, 1.500000000000002220 ) ) ;
#6897=CARTESIAN_POINT ( 'NONE',  ( -61.99999999999998579, 15.56249999999999822, 0.5000000000000013323 ) ) ;
#6899=CARTESIAN_POINT ( 'NONE',  ( -61.13531646874998415, 9.369791666325268054, 1.999225269531026417 ) ) ;
#6901=LINE ( 'NONE', #8619, #3761 ) ;
#6907=CARTESIAN_POINT ( 'NONE',  ( -62.43234176562499016, 15.24479166632526805, 2.248837904296538071 ) ) ;
#6908=CARTESIAN_POINT ( 'NONE',  ( -62.86468353124998032, 11.18229166632526983, 1.000774730468978246 ) ) ;
#6910=CARTESIAN_POINT ( 'NONE',  ( -62.43234176562498305, 8.661458332991934128, 0.7511620957034662593 ) ) ;
#6911=( BOUNDED_CURVE ( )  B_SPLINE_CURVE ( 2, ( #10447, #1174, #516, #6345, #1233, #3791, #3068, #9677, #8907 ),
 .UNSPECIFIED., .F., .F. ) 
 B_SPLINE_CURVE_WITH_KNOTS ( ( 3, 2, 2, 2, 3 ),
 ( 0.6953125000000000000, 0.6979166666666666297, 0.7031250000000000000, 0.7083333333333333703, 0.7109375000000000000 ),
 .UNSPECIFIED. ) 
 CURVE ( )  GEOMETRIC_REPRESENTATION_ITEM ( )  RATIONAL_B_SPLINE_CURVE ( ( 0.9330127018922194093, 0.9330127018922194093, 1.000000000000000000, 0.8660254037844387076, 1.000000000000000000, 0.8660254037844387076, 1.000000000000000000, 0.9330127018922194093, 0.9330127018922194093 ) ) 
 REPRESENTATION_ITEM ( '' )  );
#6912=VERTEX_POINT ( 'NONE', #1899 ) ;
#6913=CARTESIAN_POINT ( 'NONE',  ( -60.99999999999998579, 15.02083333333333393, 0.9226497308103762673 ) ) ;
#6914=CARTESIAN_POINT ( 'NONE',  ( -61.99999999999999289, 10.07812499965860198, 2.498450539062049724 ) ) ;
#6916=CARTESIAN_POINT ( 'NONE',  ( -60.99999999999998579, 13.71874999931720218, 1.500000000000002220 ) ) ;
#6919=CARTESIAN_POINT ( 'NONE',  ( -61.99999999999998579, 9.687500000000000000, 2.500000000000002665 ) ) ;
#6920=CARTESIAN_POINT ( 'NONE',  ( -61.56765823437498852, 11.28645833299193590, 2.248837904296538515 ) ) ;
#6921=DIRECTION ( 'NONE',  ( 0.000000000000000000, 0.000000000000000000, -1.000000000000000000 ) ) ;
#6926=CARTESIAN_POINT ( 'NONE',  ( -61.99999999999998579, 12.95312499965860198, 0.5015494609379544944 ) ) ;
#6928=CYLINDRICAL_SURFACE ( 'NONE', #6725, 0.9999999999999981126 ) ;
#6930=CARTESIAN_POINT ( 'NONE',  ( -60.99999999999998579, 9.697916665983870033, 2.077350269189628840 ) ) ;
#6931=ORIENTED_EDGE ( 'NONE', *, *, #7200, .T. ) ;
#6934=CARTESIAN_POINT ( 'NONE',  ( -61.13531646874998415, 11.59895833299193590, 1.000774730468978468 ) ) ;
#6936=CARTESIAN_POINT ( 'NONE',  ( -62.86468353124998032, 8.744791666325268054, 1.000774730468978246 ) ) ;
#6938=CARTESIAN_POINT ( 'NONE',  ( -62.43234176562499016, 15.05729166632526805, 2.248837904296538071 ) ) ;
#6939=CARTESIAN_POINT ( 'NONE',  ( -61.99999999999998579, 12.78124999931720218, 0.5000000000000013323 ) ) ;
#6940=ORIENTED_EDGE ( 'NONE', *, *, #9663, .F. ) ;
#6941=DIRECTION ( 'NONE',  ( -0.000000000000000000, -1.000000000000000000, -0.000000000000000000 ) ) ;
#6944=CARTESIAN_POINT ( 'NONE',  ( -62.26794919243111082, 10.92633545031537068, 2.500000000000003109 ) ) ;
#6945=CARTESIAN_POINT ( 'NONE',  ( -61.49999999999998579, 8.541666666666666075, 0.6339745962155628467 ) ) ;
#6946=CARTESIAN_POINT ( 'NONE',  ( -61.99999999999998579, 8.906249999317203958, 2.500000000000002665 ) ) ;
#6947=CARTESIAN_POINT ( 'NONE',  ( -60.99999999999998579, 10.77083333333333393, 0.9226497308103762673 ) ) ;
#6948=CARTESIAN_POINT ( 'NONE',  ( -62.86468353124999453, 14.01562499965860198, 1.500000000000002220 ) ) ;
#6949=CARTESIAN_POINT ( 'NONE',  ( -62.86468353124998742, 8.723958332991934128, 1.999225269531025972 ) ) ;
#6952=CARTESIAN_POINT ( 'NONE',  ( -61.99999999999998579, 9.828124999658600203, 2.498450539062049724 ) ) ;
#6953=CARTESIAN_POINT ( 'NONE',  ( -60.99999999999998579, 15.71874999931720218, 1.500000000000002220 ) ) ;
#6954=ORIENTED_EDGE ( 'NONE', *, *, #7550, .T. ) ;
#6959=CARTESIAN_POINT ( 'NONE',  ( -61.56765823437498852, 11.53645833299193590, 2.248837904296538515 ) ) ;
#6961=CARTESIAN_POINT ( 'NONE',  ( -62.86468353124998032, 8.432291666325268054, 1.000774730468978024 ) ) ;
#6964=CARTESIAN_POINT ( 'NONE',  ( -60.99999999999998579, 15.50000000000000000, 1.500000000000002220 ) ) ;
#6965=CARTESIAN_POINT ( 'NONE',  ( -62.86468353124999453, 9.515624999658600203, 1.500000000000002220 ) ) ;
#6967=CARTESIAN_POINT ( 'NONE',  ( -62.86468353124999453, 14.95312499965860020, 1.500000000000002220 ) ) ;
#6968=CARTESIAN_POINT ( 'NONE',  ( -62.49999999999998579, 12.88541666598386826, 2.366025403784441483 ) ) ;
#6969=CARTESIAN_POINT ( 'NONE',  ( -62.26794919243111082, 14.67633545031536890, 2.500000000000003109 ) ) ;
#6972=AXIS2_PLACEMENT_3D ( 'NONE', #4560, #10455, #7969 ) ;
#6975=CARTESIAN_POINT ( 'NONE',  ( -62.86468353124999453, 11.22395833299193590, 1.999225269531025750 ) ) ;
#6976=CYLINDRICAL_SURFACE ( 'NONE', #4039, 0.9999999999999981126 ) ;
#6977=CARTESIAN_POINT ( 'NONE',  ( -61.73205080756886076, 15.55133545031536713, 0.5000000000000014433 ) ) ;
#6979=CARTESIAN_POINT ( 'NONE',  ( -60.99999999999998579, 11.02083333333333570, 0.9226497308103762673 ) ) ;
#6980=AXIS2_PLACEMENT_3D ( 'NONE', #10838, #4009, #5045 ) ;
#6982=CARTESIAN_POINT ( 'NONE',  ( -61.13531646874998415, 14.11979166632526805, 1.999225269531026417 ) ) ;
#6984=CARTESIAN_POINT ( 'NONE',  ( -60.99999999999998579, 9.239583332650534331, 0.9226497308103762673 ) ) ;
#6986=CARTESIAN_POINT ( 'NONE',  ( -60.99999999999998579, 13.52083333333333215, 0.9226497308103762673 ) ) ;
#6989=CARTESIAN_POINT ( 'NONE',  ( -61.56765823437498852, 11.78645833299193413, 2.248837904296538515 ) ) ;
#6990=EDGE_CURVE ( 'NONE', #2594, #3363, #2565, .T. ) ;
#6992=CARTESIAN_POINT ( 'NONE',  ( -62.86468353124998032, 9.994791666325268054, 1.000774730468978246 ) ) ;
#6993=CARTESIAN_POINT ( 'NONE',  ( -61.99999999999998579, 16.00000000000000000, 1.500000000000002220 ) ) ;
#6995=CARTESIAN_POINT ( 'NONE',  ( -61.13531646874998415, 14.86979166632526805, 1.999225269531026417 ) ) ;
#6998=DIRECTION ( 'NONE',  ( 0.000000000000000000, 0.000000000000000000, -1.000000000000000000 ) ) ;
#7002=CARTESIAN_POINT ( 'NONE',  ( -62.49999999999998579, 8.083333333333332149, 0.6339745962155627357 ) ) ;
#7003=DIRECTION ( 'NONE',  ( 0.000000000000000000, 0.000000000000000000, -1.000000000000000000 ) ) ;
#7004=CARTESIAN_POINT ( 'NONE',  ( -61.99999999999998579, 10.68749999999999822, 2.500000000000002665 ) ) ;
#7005=CARTESIAN_POINT ( 'NONE',  ( -61.99999999999998579, 16.00000000000000000, 1.500000000000002220 ) ) ;
#7006=CARTESIAN_POINT ( 'NONE',  ( -61.99999999999999289, 13.70312499965860198, 0.5015494609379544944 ) ) ;
#7007=CARTESIAN_POINT ( 'NONE',  ( -62.86468353124998032, 9.182291666325268054, 1.000774730468978246 ) ) ;
#7008=CARTESIAN_POINT ( 'NONE',  ( -61.99999999999998579, 10.81250000000000000, 0.5000000000000013323 ) ) ;
#7010=CARTESIAN_POINT ( 'NONE',  ( -61.13531646874998415, 10.41145833299193413, 1.000774730468978468 ) ) ;
#7011=FACE_OUTER_BOUND ( 'NONE', #7592, .T. ) ;
#7013=CARTESIAN_POINT ( 'NONE',  ( -61.49999999999998579, 14.01041666598387003, 0.6339745962155628467 ) ) ;
#7014=CARTESIAN_POINT ( 'NONE',  ( -62.49999999999998579, 11.33333333333333393, 0.6339745962155627357 ) ) ;
#7015=CARTESIAN_POINT ( 'NONE',  ( -62.43234176562498305, 12.16145833299193413, 0.7511620957034662593 ) ) ;
#7016=CARTESIAN_POINT ( 'NONE',  ( -61.99999999999999289, 9.265624999658598426, 2.498450539062049724 ) ) ;
#7017=CARTESIAN_POINT ( 'NONE',  ( -61.99999999999997868, 9.781249999317202182, 0.5000000000000013323 ) ) ;
#7019=CARTESIAN_POINT ( 'NONE',  ( -62.49999999999998579, 15.91666666666666607, 2.366025403784441483 ) ) ;
#7020=CARTESIAN_POINT ( 'NONE',  ( -61.99999999999999289, 10.57812499965860198, 2.498450539062049724 ) ) ;
#7022=CARTESIAN_POINT ( 'NONE',  ( -62.86468353124998032, 14.93229166632526983, 1.000774730468978246 ) ) ;
#7025=CARTESIAN_POINT ( 'NONE',  ( -60.99999999999998579, 14.71874999931720218, 1.500000000000002220 ) ) ;
#7028=CARTESIAN_POINT ( 'NONE',  ( -62.49999999999998579, 11.58333333333333393, 0.6339745962155627357 ) ) ;
#7029=CARTESIAN_POINT ( 'NONE',  ( -62.43234176562498305, 10.91145833299193413, 0.7511620957034662593 ) ) ;
#7030=CARTESIAN_POINT ( 'NONE',  ( -62.43234176562499016, 8.744791666325268054, 2.248837904296538071 ) ) ;
#7032=ORIENTED_EDGE ( 'NONE', *, *, #9600, .T. ) ;
#7033=CARTESIAN_POINT ( 'NONE',  ( -62.99999999999998579, 11.35416666666666785, 0.9226497308103756012 ) ) ;
#7035=CARTESIAN_POINT ( 'NONE',  ( -62.43234176562499016, 13.80729166632526805, 2.248837904296538071 ) ) ;
#7037=CARTESIAN_POINT ( 'NONE',  ( -61.99999999999998579, 11.15624999931720396, 2.654700538379254571 ) ) ;
#7039=CARTESIAN_POINT ( 'NONE',  ( -61.99999999999998579, 13.93749999999999822, 2.500000000000002665 ) ) ;
#7041=CARTESIAN_POINT ( 'NONE',  ( -61.13531646874998415, 11.34895833299193413, 1.000774730468978468 ) ) ;
#7042=EDGE_CURVE ( 'NONE', #424, #2359, #1730, .T. ) ;
#7043=VERTEX_POINT ( 'NONE', #5106 ) ;
#7045=CARTESIAN_POINT ( 'NONE',  ( -62.86468353124999453, 10.51562499965860198, 1.500000000000002220 ) ) ;
#7046=CARTESIAN_POINT ( 'NONE',  ( -62.99999999999998579, 15.57291666598387003, 0.9226497308103756012 ) ) ;
#7047=CARTESIAN_POINT ( 'NONE',  ( -61.56765823437498142, 14.43229166632526983, 0.7511620957034663704 ) ) ;
#7048=CARTESIAN_POINT ( 'NONE',  ( -61.99999999999998579, 8.906249999317203958, 2.500000000000002665 ) ) ;
#7053=PLANE ( 'NONE',  #6790 ) ;
#7054=CARTESIAN_POINT ( 'NONE',  ( -60.99999999999998579, 9.020833333333333925, 0.9226497308103762673 ) ) ;
#7056=CARTESIAN_POINT ( 'NONE',  ( -61.99999999999998579, 12.40624999931720218, 2.500000000000002665 ) ) ;
#7058=CARTESIAN_POINT ( 'NONE',  ( -61.99999999999999289, 14.32812499965860020, 2.498450539062049724 ) ) ;
#7059=CARTESIAN_POINT ( 'NONE',  ( -61.99999999999998579, 10.01562499965860020, 2.498450539062049724 ) ) ;
#7060=DIRECTION ( 'NONE',  ( -0.000000000000000000, -1.000000000000000000, -0.000000000000000000 ) ) ;
#7061=EDGE_CURVE ( 'NONE', #10637, #8021, #2584, .T. ) ;
#7063=CARTESIAN_POINT ( 'NONE',  ( -62.43234176562499016, 10.80729166632526805, 2.248837904296538071 ) ) ;
#7064=CARTESIAN_POINT ( 'NONE',  ( -60.99999999999998579, 8.109374999658601979, 1.500000000000002220 ) ) ;
#7067=CARTESIAN_POINT ( 'NONE',  ( -61.49999999999998579, 15.20833333333333393, 2.366025403784441927 ) ) ;
#7068=( BOUNDED_CURVE ( )  B_SPLINE_CURVE ( 2, ( #2430, #2280, #9219, #6566, #8327, #9948, #10827, #9110, #5608 ),
 .UNSPECIFIED., .F., .T. ) 
 B_SPLINE_CURVE_WITH_KNOTS ( ( 3, 2, 2, 2, 3 ),
 ( 0.8359375000000000000, 0.8385416666666666297, 0.8437500000000000000, 0.8489583333333333703, 0.8515625000000000000 ),
 .UNSPECIFIED. ) 
 CURVE ( )  GEOMETRIC_REPRESENTATION_ITEM ( )  RATIONAL_B_SPLINE_CURVE ( ( 0.9330127018922194093, 0.9330127018922194093, 1.000000000000000000, 0.8660254037844387076, 1.000000000000000000, 0.8660254037844387076, 1.000000000000000000, 0.9330127018922194093, 0.9330127018922194093 ) ) 
 REPRESENTATION_ITEM ( '' )  );
#7069=CARTESIAN_POINT ( 'NONE',  ( -62.99999999999998579, 10.07291666598387003, 0.9226497308103756012 ) ) ;
#7070=CARTESIAN_POINT ( 'NONE',  ( -62.43234176562499016, 12.99479166632526805, 2.248837904296538071 ) ) ;
#7072=CARTESIAN_POINT ( 'NONE',  ( -62.43234176562499016, 8.244791666325268054, 2.248837904296538071 ) ) ;
#7075=VERTEX_POINT ( 'NONE', #8909 ) ;
#7076=CARTESIAN_POINT ( 'NONE',  ( -61.99999999999997868, 10.90624999931720218, 2.500000000000002665 ) ) ;
#7077=CARTESIAN_POINT ( 'NONE',  ( -61.56765823437498142, 10.43229166632526983, 0.7511620957034663704 ) ) ;
#7080=CARTESIAN_POINT ( 'NONE',  ( -62.86468353124999453, 15.70312499965860198, 1.500000000000002220 ) ) ;
#7081=CARTESIAN_POINT ( 'NONE',  ( -61.99999999999998579, 14.90624999931720218, 2.654700538379254571 ) ) ;
#7082=FACE_OUTER_BOUND ( 'NONE', #4518, .T. ) ;
#7083=VERTEX_POINT ( 'NONE', #10449 ) ;
#7085=LINE ( 'NONE', #3748, #1819 ) ;
#7087=ORIENTED_EDGE ( 'NONE', *, *, #6766, .F. ) ;
#7088=CARTESIAN_POINT ( 'NONE',  ( -61.56765823437498142, 12.36979166632526805, 0.7511620957034663704 ) ) ;
#7090=CARTESIAN_POINT ( 'NONE',  ( -62.43234176562498305, 8.911458332991934128, 0.7511620957034662593 ) ) ;
#7091=DIRECTION ( 'NONE',  ( 0.000000000000000000, 1.000000000000000000, 0.000000000000000000 ) ) ;
#7092=ORIENTED_EDGE ( 'NONE', *, *, #5919, .F. ) ;
#7093=CARTESIAN_POINT ( 'NONE',  ( -62.99999999999998579, 12.14583333333333393, 2.077350269189627952 ) ) ;
#7096=CARTESIAN_POINT ( 'NONE',  ( -61.13531646874998415, 14.41145833299193413, 1.000774730468978468 ) ) ;
#7097=CARTESIAN_POINT ( 'NONE',  ( -62.99999999999998579, 13.85416666666666785, 0.9226497308103756012 ) ) ;
#7098=CARTESIAN_POINT ( 'NONE',  ( -62.49999999999998579, 10.30208333265053611, 0.6339745962155627357 ) ) ;
#7099=VECTOR ( 'NONE', #5438, 1000.000000000000000 ) ;
#7101=FACE_OUTER_BOUND ( 'NONE', #1316, .T. ) ;
#7103=VECTOR ( 'NONE', #7721, 1000.000000000000000 ) ;
#7104=CARTESIAN_POINT ( 'NONE',  ( -62.43234176562499016, 12.24479166632526805, 2.248837904296538071 ) ) ;
#7106=ORIENTED_EDGE ( 'NONE', *, *, #792, .T. ) ;
#7107=CARTESIAN_POINT ( 'NONE',  ( -61.13531646874998415, 10.61979166632526983, 1.999225269531026417 ) ) ;
#7110=CARTESIAN_POINT ( 'NONE',  ( -61.13531646874998415, 14.11979166632526805, 1.999225269531026417 ) ) ;
#7115=ORIENTED_EDGE ( 'NONE', *, *, #9918, .T. ) ;
#7117=CARTESIAN_POINT ( 'NONE',  ( -62.99999999999998579, 8.854166666666667851, 0.9226497308103756012 ) ) ;
#7118=LINE ( 'NONE', #8009, #64 ) ;
#7119=CARTESIAN_POINT ( 'NONE',  ( -60.99999999999998579, 16.19791666598386826, 2.077350269189628840 ) ) ;
#7121=CARTESIAN_POINT ( 'NONE',  ( -62.43234176562498305, 14.22395833299193413, 0.7511620957034662593 ) ) ;
#7122=CARTESIAN_POINT ( 'NONE',  ( -61.13531646874998415, 10.34895833299193413, 1.000774730468978468 ) ) ;
#7125=CARTESIAN_POINT ( 'NONE',  ( -62.86468353124998742, 10.53645833299193413, 1.999225269531025972 ) ) ;
#7126=DIRECTION ( 'NONE',  ( 1.000000000000000000, 0.000000000000000000, -0.000000000000000000 ) ) ;
#7127=ORIENTED_EDGE ( 'NONE', *, *, #5472, .T. ) ;
#7128=CARTESIAN_POINT ( 'NONE',  ( -62.99999999999998579, 14.35416666666666785, 0.9226497308103756012 ) ) ;
#7131=CARTESIAN_POINT ( 'NONE',  ( -61.99999999999998579, 16.00000000000000000, 2.500000000000000444 ) ) ;
#7133=CARTESIAN_POINT ( 'NONE',  ( -61.13531646874998415, 12.09895833299193235, 1.000774730468978468 ) ) ;
#7134=CARTESIAN_POINT ( 'NONE',  ( -61.13531646874997705, 10.55729166632526805, 1.999225269531026417 ) ) ;
#7137=CARTESIAN_POINT ( 'NONE',  ( -60.99999999999998579, 8.489583332650536107, 0.9226497308103762673 ) ) ;
#7138=AXIS2_PLACEMENT_3D ( 'NONE', #6138, #1863, #1805 ) ;
#7139=CARTESIAN_POINT ( 'NONE',  ( -62.43234176562499016, 10.55729166632526983, 2.248837904296538071 ) ) ;
#7141=CARTESIAN_POINT ( 'NONE',  ( -61.13531646874998415, 15.32812499965860020, 1.500000000000002220 ) ) ;
#7142=CARTESIAN_POINT ( 'NONE',  ( -62.49999999999998579, 15.13541666598387003, 2.366025403784441483 ) ) ;
#7143=CARTESIAN_POINT ( 'NONE',  ( -61.49999999999998579, 14.76041666598386826, 0.6339745962155628467 ) ) ;
#7144=ORIENTED_EDGE ( 'NONE', *, *, #4382, .T. ) ;
#7146=( BOUNDED_CURVE ( )  B_SPLINE_CURVE ( 2, ( #3815, #7205, #4693, #3869, #3923, #2983, #3091, #6369, #543 ),
 .UNSPECIFIED., .F., .T. ) 
 B_SPLINE_CURVE_WITH_KNOTS ( ( 3, 2, 2, 2, 3 ),
 ( 0.4609375000000000000, 0.4635416666666666852, 0.4687500000000000000, 0.4739583333333333148, 0.4765625000000000000 ),
 .UNSPECIFIED. ) 
 CURVE ( )  GEOMETRIC_REPRESENTATION_ITEM ( )  RATIONAL_B_SPLINE_CURVE ( ( 0.9330127018922194093, 0.9330127018922194093, 1.000000000000000000, 0.8660254037844387076, 1.000000000000000000, 0.8660254037844387076, 1.000000000000000000, 0.9330127018922194093, 0.9330127018922194093 ) ) 
 REPRESENTATION_ITEM ( '' )  );
#7148=CARTESIAN_POINT ( 'NONE',  ( -61.13531646874998415, 12.82812499965860198, 1.500000000000002220 ) ) ;
#7149=CARTESIAN_POINT ( 'NONE',  ( -62.86468353124999453, 8.203124999658601979, 1.500000000000002220 ) ) ;
#7150=CARTESIAN_POINT ( 'NONE',  ( -62.49999999999998579, 10.63541666598387003, 2.366025403784441483 ) ) ;
#7152=CARTESIAN_POINT ( 'NONE',  ( -61.99999999999998579, 12.56250000000000178, 0.3452994616207497591 ) ) ;
#7153=CARTESIAN_POINT ( 'NONE',  ( -61.99999999999998579, 14.70312499965860020, 0.5015494609379544944 ) ) ;
#7155=CARTESIAN_POINT ( 'NONE',  ( -62.99999999999998579, 10.34374999931720218, 1.500000000000001998 ) ) ;
#7158=CARTESIAN_POINT ( 'NONE',  ( -61.99999999999998579, 10.40624999931720218, 2.500000000000002665 ) ) ;
#7159=CARTESIAN_POINT ( 'NONE',  ( -61.13531646874998415, 12.09895833299193235, 1.000774730468978468 ) ) ;
#7162=CARTESIAN_POINT ( 'NONE',  ( -61.56765823437498852, 10.84895833299193413, 2.248837904296538515 ) ) ;
#7166=CARTESIAN_POINT ( 'NONE',  ( -62.43234176562499016, 14.80729166632526805, 2.248837904296538071 ) ) ;
#7168=ORIENTED_EDGE ( 'NONE', *, *, #821, .F. ) ;
#7169=CARTESIAN_POINT ( 'NONE',  ( -62.99999999999998579, 9.375000000000000000, 1.500000000000001998 ) ) ;
#7172=CARTESIAN_POINT ( 'NONE',  ( -62.49999999999998579, 8.916666666666666075, 2.366025403784441483 ) ) ;
#7176=CARTESIAN_POINT ( 'NONE',  ( -62.86468353124998032, 9.682291666325266277, 1.000774730468978246 ) ) ;
#7179=CARTESIAN_POINT ( 'NONE',  ( -61.99999999999998579, 16.00000000000000000, 2.500000000000000444 ) ) ;
#7180=CARTESIAN_POINT ( 'NONE',  ( -61.99999999999998579, 10.20312499965860198, 0.5015494609379544944 ) ) ;
#7183=CARTESIAN_POINT ( 'NONE',  ( -61.99999999999998579, 14.03124999931720218, 0.5000000000000013323 ) ) ;
#7185=ORIENTED_EDGE ( 'NONE', *, *, #3260, .F. ) ;
#7186=CARTESIAN_POINT ( 'NONE',  ( -60.99999999999998579, 15.75000000000000000, 1.500000000000002220 ) ) ;
#7188=CARTESIAN_POINT ( 'NONE',  ( -61.56765823437498852, 12.03645833299193413, 2.248837904296538515 ) ) ;
#7189=CARTESIAN_POINT ( 'NONE',  ( -62.43234176562498305, 10.16145833299193413, 0.7511620957034662593 ) ) ;
#7190=DIRECTION ( 'NONE',  ( -0.000000000000000000, -1.000000000000000000, -0.000000000000000000 ) ) ;
#7192=CARTESIAN_POINT ( 'NONE',  ( -61.49999999999998579, 15.95833333333333215, 2.366025403784441927 ) ) ;
#7193=CARTESIAN_POINT ( 'NONE',  ( -61.99999999999999289, 10.82812499965860198, 2.498450539062049724 ) ) ;
#7196=CARTESIAN_POINT ( 'NONE',  ( -61.13531646874998415, 15.07812499965860020, 1.500000000000002220 ) ) ;
#7197=CARTESIAN_POINT ( 'NONE',  ( -62.99999999999998579, 14.07291666598387003, 0.9226497308103756012 ) ) ;
#7200=EDGE_CURVE ( 'NONE', #8261, #8575, #5507, .T. ) ;
#7201=CARTESIAN_POINT ( 'NONE',  ( -61.73205080756886076, 15.16741454900183328, 2.500000000000003109 ) ) ;
#7203=CARTESIAN_POINT ( 'NONE',  ( -61.13531646874998415, 13.32812499965860020, 1.500000000000002220 ) ) ;
#7204=CARTESIAN_POINT ( 'NONE',  ( -61.13531646874998415, 8.078124999658601979, 1.500000000000002220 ) ) ;
#7205=CARTESIAN_POINT ( 'NONE',  ( -61.73205080756886076, 11.69866454968463110, 2.500000000000003109 ) ) ;
#7207=CARTESIAN_POINT ( 'NONE',  ( -62.99999999999998579, 12.12500000000000000, 1.500000000000001998 ) ) ;
#7208=CARTESIAN_POINT ( 'NONE',  ( -60.99999999999998579, 14.97916666666666430, 2.077350269189628840 ) ) ;
#7209=CARTESIAN_POINT ( 'NONE',  ( -61.49999999999998579, 11.17708333265053611, 2.366025403784441927 ) ) ;
#7211=( BOUNDED_CURVE ( )  B_SPLINE_CURVE ( 2, ( #163, #10322, #8727, #4434, #8610, #4316, #2671, #7726, #6946 ),
 .UNSPECIFIED., .F., .T. ) 
 B_SPLINE_CURVE_WITH_KNOTS ( ( 3, 2, 2, 2, 3 ),
 ( 0.07031250000000001388, 0.07291666666666667129, 0.07812500000000000000, 0.08333333333333332871, 0.08593750000000000000 ),
 .UNSPECIFIED. ) 
 CURVE ( )  GEOMETRIC_REPRESENTATION_ITEM ( )  RATIONAL_B_SPLINE_CURVE ( ( 0.9330127018922192983, 0.9330127018922196314, 1.000000000000000000, 0.8660254037844387076, 1.000000000000000000, 0.8660254037844387076, 1.000000000000000000, 0.9330127018922194093, 0.9330127018922194093 ) ) 
 REPRESENTATION_ITEM ( '' )  );
#7213=CARTESIAN_POINT ( 'NONE',  ( -61.13531646874998415, 13.07812499965860198, 1.500000000000002220 ) ) ;
#7214=CARTESIAN_POINT ( 'NONE',  ( -61.99999999999998579, 15.93749999999999645, 2.500000000000002665 ) ) ;
#7216=CARTESIAN_POINT ( 'NONE',  ( -62.43234176562499016, 10.80729166632526805, 2.248837904296538071 ) ) ;
#7218=CARTESIAN_POINT ( 'NONE',  ( -62.99999999999998579, 12.59374999931720396, 1.500000000000001998 ) ) ;
#7219=CARTESIAN_POINT ( 'NONE',  ( -61.13531646874998415, 15.91145833299193590, 1.000774730468978468 ) ) ;
#7220=LINE ( 'NONE', #1216, #7673 ) ;
#7222=EDGE_CURVE ( 'NONE', #5865, #4030, #5671, .T. ) ;
#7224=ORIENTED_EDGE ( 'NONE', *, *, #1371, .F. ) ;
#7227=CARTESIAN_POINT ( 'NONE',  ( -61.49999999999998579, 10.29166666666666785, 0.6339745962155628467 ) ) ;
#7229=DIRECTION ( 'NONE',  ( -0.8660254037844418162, 0.4999999999999947264, -0.000000000000000000 ) ) ;
#7231=CARTESIAN_POINT ( 'NONE',  ( -62.86468353124999453, 10.45312499965860198, 1.500000000000002220 ) ) ;
#7232=DIRECTION ( 'NONE',  ( 0.000000000000000000, 0.000000000000000000, -1.000000000000000000 ) ) ;
#7233=CARTESIAN_POINT ( 'NONE',  ( -61.56765823437498142, 11.18229166632526805, 0.7511620957034663704 ) ) ;
#7234=CARTESIAN_POINT ( 'NONE',  ( -62.99999999999998579, 12.14583333333333393, 2.077350269189627952 ) ) ;
#7236=CARTESIAN_POINT ( 'NONE',  ( -60.99999999999998579, 13.96874999931720218, 1.500000000000002220 ) ) ;
#7240=CARTESIAN_POINT ( 'NONE',  ( -60.99999999999998579, 9.979166666666667851, 2.077350269189628840 ) ) ;
#7241=CARTESIAN_POINT ( 'NONE',  ( -62.86468353124998742, 14.47395833299193413, 1.999225269531025972 ) ) ;
#7242=CARTESIAN_POINT ( 'NONE',  ( -61.13531646874997705, 9.598958332991934128, 1.000774730468978468 ) ) ;
#7245=CARTESIAN_POINT ( 'NONE',  ( -62.99999999999998579, 15.87500000000000000, 1.500000000000001998 ) ) ;
#7246=CARTESIAN_POINT ( 'NONE',  ( -61.13531646874998415, 11.64062499965860198, 1.500000000000002220 ) ) ;
#7249=CARTESIAN_POINT ( 'NONE',  ( -62.99999999999998579, 14.59374999931720218, 1.500000000000001998 ) ) ;
#7250=CARTESIAN_POINT ( 'NONE',  ( -61.99999999999998579, 8.000000000000000000, 2.500000000000000444 ) ) ;
#7254=ORIENTED_EDGE ( 'NONE', *, *, #1855, .F. ) ;
#7256=EDGE_CURVE ( 'NONE', #7667, #3055, #2111, .T. ) ;
#7257=CARTESIAN_POINT ( 'NONE',  ( -62.86468353124999453, 13.45312499965860020, 1.500000000000002220 ) ) ;
#7258=CARTESIAN_POINT ( 'NONE',  ( -62.86468353124998742, 8.973958332991934128, 1.999225269531025972 ) ) ;
#7262=CARTESIAN_POINT ( 'NONE',  ( -60.99999999999998579, 12.47916666666666607, 2.077350269189628840 ) ) ;
#7263=CARTESIAN_POINT ( 'NONE',  ( -60.99999999999998579, 9.000000000000001776, 1.500000000000002220 ) ) ;
#7264=CARTESIAN_POINT ( 'NONE',  ( -61.99999999999998579, 16.00000000000000000, 1.500000000000002220 ) ) ;
#7266=CARTESIAN_POINT ( 'NONE',  ( -61.99999999999998579, 10.15624999931720218, 2.654700538379254571 ) ) ;
#7270=CARTESIAN_POINT ( 'NONE',  ( -61.56765823437498852, 12.53645833299193413, 2.248837904296538515 ) ) ;
#7271=CARTESIAN_POINT ( 'NONE',  ( -61.99999999999998579, 16.00000000000000000, 2.500000000000000444 ) ) ;
#7275=CARTESIAN_POINT ( 'NONE',  ( -62.86468353124999453, 11.51562499965860020, 1.500000000000002220 ) ) ;
#7276=( BOUNDED_CURVE ( )  B_SPLINE_CURVE ( 2, ( #2075, #6178, #2019, #7240, #4557, #8854, #1960, #7908, #7965 ),
 .UNSPECIFIED., .F., .T. ) 
 B_SPLINE_CURVE_WITH_KNOTS ( ( 3, 2, 2, 2, 3 ),
 ( 0.2421875000000000000, 0.2447916666666666574, 0.2500000000000000000, 0.2552083333333333148, 0.2578125000000000000 ),
 .UNSPECIFIED. ) 
 CURVE ( )  GEOMETRIC_REPRESENTATION_ITEM ( )  RATIONAL_B_SPLINE_CURVE ( ( 0.9330127018922194093, 0.9330127018922194093, 1.000000000000000000, 0.8660254037844387076, 1.000000000000000000, 0.8660254037844387076, 1.000000000000000000, 0.9330127018922194093, 0.9330127018922194093 ) ) 
 REPRESENTATION_ITEM ( '' )  );
#7277=DIRECTION ( 'NONE',  ( 0.000000000000000000, 0.000000000000000000, -1.000000000000000000 ) ) ;
#7280=CARTESIAN_POINT ( 'NONE',  ( -61.49999999999998579, 9.458333333333332149, 2.366025403784441927 ) ) ;
#7282=CARTESIAN_POINT ( 'NONE',  ( -62.49999999999998579, 11.16666666666666607, 2.366025403784441483 ) ) ;
#7286=CARTESIAN_POINT ( 'NONE',  ( -62.99999999999998579, 9.895833333333333925, 2.077350269189627952 ) ) ;
#7288=CARTESIAN_POINT ( 'NONE',  ( -62.99999999999998579, 9.572916665983870033, 0.9226497308103756012 ) ) ;
#7290=CARTESIAN_POINT ( 'NONE',  ( -62.99999999999998579, 14.82291666598386826, 0.9226497308103756012 ) ) ;
#7292=CARTESIAN_POINT ( 'NONE',  ( -61.99999999999998579, 11.20312499965860198, 0.5015494609379544944 ) ) ;
#7296=CARTESIAN_POINT ( 'NONE',  ( -61.99999999999998579, 9.062500000000000000, 0.5000000000000013323 ) ) ;
#7299=CARTESIAN_POINT ( 'NONE',  ( -61.13531646874998415, 13.55729166632526805, 1.999225269531026417 ) ) ;
#7300=CARTESIAN_POINT ( 'NONE',  ( -62.86468353124999453, 9.723958332991934128, 1.999225269531025750 ) ) ;
#7301=CARTESIAN_POINT ( 'NONE',  ( -61.73205080756886076, 11.66741454900183506, 2.500000000000000000 ) ) ;
#7302=VERTEX_POINT ( 'NONE', #625 ) ;
#7303=FACE_OUTER_BOUND ( 'NONE', #9915, .T. ) ;
#7304=CARTESIAN_POINT ( 'NONE',  ( -61.99999999999999289, 11.82812499965860198, 2.498450539062049724 ) ) ;
#7306=CARTESIAN_POINT ( 'NONE',  ( -62.49999999999998579, 15.38541666598387003, 2.366025403784441483 ) ) ;
#7307=CARTESIAN_POINT ( 'NONE',  ( -62.99999999999998579, 16.11458333265053255, 2.077350269189627952 ) ) ;
#7308=EDGE_LOOP ( 'NONE', ( #5119, #8224, #2147, #2601 ) ) ;
#7309=VERTEX_POINT ( 'NONE', #4005 ) ;
#7310=VECTOR ( 'NONE', #2035, 1000.000000000000000 ) ;
#7311=CARTESIAN_POINT ( 'NONE',  ( -61.99999999999999289, 13.39062499965860020, 0.5015494609379544944 ) ) ;
#7312=CARTESIAN_POINT ( 'NONE',  ( -61.13531646874998415, 9.328124999658600203, 1.500000000000002220 ) ) ;
#7313=LINE ( 'NONE', #10530, #5008 ) ;
#7315=CARTESIAN_POINT ( 'NONE',  ( -61.49999999999998579, 12.45833333333333393, 2.366025403784441927 ) ) ;
#7316=CYLINDRICAL_SURFACE ( 'NONE', #5540, 0.9999999999999981126 ) ;
#7318=CARTESIAN_POINT ( 'NONE',  ( -62.99999999999998579, 12.57291666598387003, 0.9226497308103756012 ) ) ;
#7319=EDGE_CURVE ( 'NONE', #5402, #6260, #7922, .T. ) ;
#7321=CARTESIAN_POINT ( 'NONE',  ( -61.99999999999998579, 12.14062499965860198, 0.5015494609379544944 ) ) ;
#7322=CARTESIAN_POINT ( 'NONE',  ( -61.99999999999998579, 16.00000000000000000, 1.500000000000002220 ) ) ;
#7323=ORIENTED_EDGE ( 'NONE', *, *, #1326, .T. ) ;
#7324=CIRCLE ( 'NONE', #10698, 0.9999999999999983347 ) ;
#7326=CARTESIAN_POINT ( 'NONE',  ( -61.99999999999998579, 11.07812499965860020, 2.498450539062049724 ) ) ;
#7327=CARTESIAN_POINT ( 'NONE',  ( -61.99999999999998579, 16.00000000000000000, 1.500000000000002220 ) ) ;
#7336=CARTESIAN_POINT ( 'NONE',  ( -62.26794919243111082, 9.792414549001835056, 0.4999999999999982792 ) ) ;
#7337=CARTESIAN_POINT ( 'NONE',  ( -60.99999999999998579, 10.22916666666666785, 2.077350269189628840 ) ) ;
#7339=CARTESIAN_POINT ( 'NONE',  ( -61.73205080756884655, 8.198664549684629321, 2.500000000000004885 ) ) ;
#7341=CARTESIAN_POINT ( 'NONE',  ( -61.99999999999998579, 15.40624999931720218, 2.500000000000002665 ) ) ;
#7342=CARTESIAN_POINT ( 'NONE',  ( -62.86468353124998032, 11.24479166632526805, 1.000774730468978246 ) ) ;
#7343=CARTESIAN_POINT ( 'NONE',  ( -61.06765823437498852, 8.039062499829300990, 1.500000000000002220 ) ) ;
#7344=VERTEX_POINT ( 'NONE', #5722 ) ;
#7347=AXIS2_PLACEMENT_3D ( 'NONE', #10206, #6050, #7003 ) ;
#7348=ORIENTED_EDGE ( 'NONE', *, *, #7696, .F. ) ;
#7349=DIRECTION ( 'NONE',  ( -0.000000000000000000, -1.000000000000000000, -0.000000000000000000 ) ) ;
#7350=CARTESIAN_POINT ( 'NONE',  ( -62.86468353124999453, 13.45312499965860020, 1.500000000000002220 ) ) ;
#7351=CARTESIAN_POINT ( 'NONE',  ( -61.13531646874997705, 10.59895833299193413, 1.000774730468978468 ) ) ;
#7352=CARTESIAN_POINT ( 'NONE',  ( -60.99999999999998579, 11.71874999931720218, 1.500000000000002220 ) ) ;
#7355=CARTESIAN_POINT ( 'NONE',  ( -61.56765823437498142, 11.93229166632526805, 0.7511620957034663704 ) ) ;
#7356=CARTESIAN_POINT ( 'NONE',  ( -61.56765823437498852, 14.84895833299193413, 2.248837904296538515 ) ) ;
#7358=EDGE_CURVE ( 'NONE', #9209, #4452, #10004, .T. ) ;
#7360=CARTESIAN_POINT ( 'NONE',  ( -61.99999999999998579, 15.65624999931720218, 2.654700538379254571 ) ) ;
#7364=CARTESIAN_POINT ( 'NONE',  ( -61.99999999999998579, 16.00000000000000000, 1.500000000000002220 ) ) ;
#7366=CARTESIAN_POINT ( 'NONE',  ( -61.99999999999999289, 14.76562499965860198, 2.498450539062049724 ) ) ;
#7367=CARTESIAN_POINT ( 'NONE',  ( -62.43234176562498305, 10.41145833299193413, 0.7511620957034662593 ) ) ;
#7368=CARTESIAN_POINT ( 'NONE',  ( -61.99999999999998579, 14.53124999931720041, 0.5000000000000013323 ) ) ;
#7369=ORIENTED_EDGE ( 'NONE', *, *, #2448, .T. ) ;
#7370=CARTESIAN_POINT ( 'NONE',  ( -60.99999999999998579, 14.02083333333333215, 0.9226497308103762673 ) ) ;
#7374=( BOUNDED_CURVE ( )  B_SPLINE_CURVE ( 2, ( #7758, #1869, #2041, #10361, #10300, #10478, #8707, #9474, #2758 ),
 .UNSPECIFIED., .F., .F. ) 
 B_SPLINE_CURVE_WITH_KNOTS ( ( 3, 2, 2, 2, 3 ),
 ( 0.3671875000000000000, 0.3697916666666666852, 0.3750000000000000000, 0.3802083333333333148, 0.3828125000000000000 ),
 .UNSPECIFIED. ) 
 CURVE ( )  GEOMETRIC_REPRESENTATION_ITEM ( )  RATIONAL_B_SPLINE_CURVE ( ( 0.9330127018922194093, 0.9330127018922194093, 1.000000000000000000, 0.8660254037844387076, 1.000000000000000000, 0.8660254037844387076, 1.000000000000000000, 0.9330127018922194093, 0.9330127018922194093 ) ) 
 REPRESENTATION_ITEM ( '' )  );
#7375=PRESENTATION_STYLE_ASSIGNMENT (( #4135 ) ) ;
#7377=CARTESIAN_POINT ( 'NONE',  ( -62.49999999999998579, 11.38541666598387003, 2.366025403784441483 ) ) ;
#7379=CARTESIAN_POINT ( 'NONE',  ( -61.13531646874998415, 14.30729166632526983, 1.999225269531026417 ) ) ;
#7382=CARTESIAN_POINT ( 'NONE',  ( -61.13531646874998415, 12.14062499965860198, 1.500000000000002220 ) ) ;
#7383=CARTESIAN_POINT ( 'NONE',  ( -61.99999999999998579, 16.00000000000000000, 0.5000000000000041078 ) ) ;
#7384=CARTESIAN_POINT ( 'NONE',  ( -62.86468353124999453, 15.26562499965860020, 1.500000000000002220 ) ) ;
#7391=CARTESIAN_POINT ( 'NONE',  ( -60.99999999999998579, 9.250000000000000000, 1.500000000000002220 ) ) ;
#7392=CARTESIAN_POINT ( 'NONE',  ( -61.99999999999998579, 16.00000000000000000, 0.5000000000000041078 ) ) ;
#7393=CARTESIAN_POINT ( 'NONE',  ( -61.99999999999997868, 8.437500000000000000, 2.500000000000002665 ) ) ;
#7395=CARTESIAN_POINT ( 'NONE',  ( -62.99999999999998579, 8.593749999317203958, 1.500000000000001998 ) ) ;
#7396=CARTESIAN_POINT ( 'NONE',  ( -62.43234176562498305, 12.22395833299193413, 0.7511620957034662593 ) ) ;
#7399=CARTESIAN_POINT ( 'NONE',  ( -61.49999999999998579, 9.177083332650536107, 2.366025403784441927 ) ) ;
#7401=CARTESIAN_POINT ( 'NONE',  ( -61.49999999999998579, 13.76041666598387003, 0.6339745962155628467 ) ) ;
#7402=CARTESIAN_POINT ( 'NONE',  ( -62.86468353124998032, 13.68229166632526983, 1.000774730468978246 ) ) ;
#7403=CARTESIAN_POINT ( 'NONE',  ( -61.49999999999998579, 13.79166666666666785, 0.6339745962155628467 ) ) ;
#7404=CARTESIAN_POINT ( 'NONE',  ( -62.26794919243110371, 8.073664549684629321, 0.4999999999999997780 ) ) ;
#7405=CARTESIAN_POINT ( 'NONE',  ( -62.26794919243111082, 14.17633545031537068, 2.500000000000003109 ) ) ;
#7406=CARTESIAN_POINT ( 'NONE',  ( -61.56765823437498852, 10.84895833299193413, 2.248837904296538515 ) ) ;
#7407=EDGE_CURVE ( 'NONE', #4570, #1925, #1668, .T. ) ;
#7408=CARTESIAN_POINT ( 'NONE',  ( -62.86468353124999453, 15.26562499965860020, 1.500000000000002220 ) ) ;
#7411=CARTESIAN_POINT ( 'NONE',  ( -62.86468353124998032, 8.494791666325268054, 1.000774730468978246 ) ) ;
#7414=CARTESIAN_POINT ( 'NONE',  ( -62.26794919243111082, 11.89508544963257286, 2.500000000000003109 ) ) ;
#7415=CARTESIAN_POINT ( 'NONE',  ( -61.49999999999998579, 8.041666666666667851, 0.6339745962155628467 ) ) ;
#7416=CARTESIAN_POINT ( 'NONE',  ( -62.86468353124998032, 14.18229166632526983, 1.000774730468978024 ) ) ;
#7417=CARTESIAN_POINT ( 'NONE',  ( -62.86468353124998742, 10.47395833299193413, 1.999225269531025972 ) ) ;
#7421=CARTESIAN_POINT ( 'NONE',  ( -61.99999999999998579, 13.18750000000000000, 2.654700538379254571 ) ) ;
#7423=CARTESIAN_POINT ( 'NONE',  ( -62.49999999999998579, 11.13541666598387003, 2.366025403784441483 ) ) ;
#7425=( NAMED_UNIT ( * ) SI_UNIT ( $, .STERADIAN. ) SOLID_ANGLE_UNIT ( ) );
#7426=CARTESIAN_POINT ( 'NONE',  ( -62.49999999999998579, 12.13541666598386826, 2.366025403784441483 ) ) ;
#7431=CARTESIAN_POINT ( 'NONE',  ( -61.56765823437498142, 13.61979166632526805, 0.7511620957034663704 ) ) ;
#7432=CYLINDRICAL_SURFACE ( 'NONE', #9191, 0.9999999999999981126 ) ;
#7433=( BOUNDED_CURVE ( )  B_SPLINE_CURVE ( 2, ( #4914, #10865, #3202, #7537, #1535, #10715, #4970, #705, #10915 ),
 .UNSPECIFIED., .F., .F. ) 
 B_SPLINE_CURVE_WITH_KNOTS ( ( 3, 2, 2, 2, 3 ),
 ( 0.4296875000000000555, 0.4322916666666666852, 0.4375000000000000000, 0.4427083333333333148, 0.4453125000000000000 ),
 .UNSPECIFIED. ) 
 CURVE ( )  GEOMETRIC_REPRESENTATION_ITEM ( )  RATIONAL_B_SPLINE_CURVE ( ( 0.9330127018922192983, 0.9330127018922207416, 1.000000000000000000, 0.8660254037844387076, 1.000000000000000000, 0.8660254037844387076, 1.000000000000000000, 0.9330127018922194093, 0.9330127018922194093 ) ) 
 REPRESENTATION_ITEM ( '' )  );
#7435=VECTOR ( 'NONE', #7229, 999.9999999999998863 ) ;
#7436=CARTESIAN_POINT ( 'NONE',  ( -61.99999999999998579, 11.70312499965860020, 0.5015494609379544944 ) ) ;
#7437=FACE_OUTER_BOUND ( 'NONE', #7879, .T. ) ;
#7438=CARTESIAN_POINT ( 'NONE',  ( -61.13531646874998415, 15.86979166632526628, 1.999225269531026417 ) ) ;
#7443=ORIENTED_EDGE ( 'NONE', *, *, #5823, .T. ) ;
#7444=CARTESIAN_POINT ( 'NONE',  ( -60.99999999999998579, 8.718749999317203958, 1.500000000000002220 ) ) ;
#7445=CARTESIAN_POINT ( 'NONE',  ( -61.99999999999998579, 9.187500000000000000, 2.654700538379254571 ) ) ;
#7446=CARTESIAN_POINT ( 'NONE',  ( -62.86468353124998032, 8.244791666325268054, 1.000774730468978246 ) ) ;
#7447=CARTESIAN_POINT ( 'NONE',  ( -60.99999999999998579, 8.250000000000000000, 1.500000000000002220 ) ) ;
#7449=CARTESIAN_POINT ( 'NONE',  ( -61.73205080756886076, 15.52008544963257108, 0.5000000000000014433 ) ) ;
#7450=CARTESIAN_POINT ( 'NONE',  ( -62.43234176562499016, 11.80729166632526805, 2.248837904296538071 ) ) ;
#7451=EDGE_CURVE ( 'NONE', #3127, #9814, #9433, .T. ) ;
#7452=COLOUR_RGB ( '',0.8941176470588234615, 0.8941176470588234615, 0.8941176470588234615 ) ;
#7453=CARTESIAN_POINT ( 'NONE',  ( -62.26794919243111082, 10.57366454968463110, 0.5000000000000013323 ) ) ;
#7454=ORIENTED_EDGE ( 'NONE', *, *, #10783, .F. ) ;
#7458=CARTESIAN_POINT ( 'NONE',  ( -61.13531646874998415, 13.80729166632526983, 1.999225269531026417 ) ) ;
#7461=CARTESIAN_POINT ( 'NONE',  ( -62.49999999999998579, 8.083333333333332149, 0.6339745962155627357 ) ) ;
#7463=CARTESIAN_POINT ( 'NONE',  ( -62.86468353124998032, 12.24479166632526805, 1.000774730468978024 ) ) ;
#7464=CARTESIAN_POINT ( 'NONE',  ( -62.43234176562499016, 15.05729166632526805, 2.248837904296538071 ) ) ;
#7467=DIRECTION ( 'NONE',  ( -0.000000000000000000, -1.000000000000000000, -0.000000000000000000 ) ) ;
#7468=CARTESIAN_POINT ( 'NONE',  ( -61.56765823437498142, 8.182291666325268054, 0.7511620957034663704 ) ) ;
#7472=DIRECTION ( 'NONE',  ( 0.000000000000000000, 0.000000000000000000, -1.000000000000000000 ) ) ;
#7474=CARTESIAN_POINT ( 'NONE',  ( -62.43234176562498305, 13.91145833299193413, 0.7511620957034662593 ) ) ;
#7475=CARTESIAN_POINT ( 'NONE',  ( -62.43234176562498305, 9.911458332991934128, 0.7511620957034662593 ) ) ;
#7476=CARTESIAN_POINT ( 'NONE',  ( -61.13531646874997705, 8.098958332991934128, 1.000774730468978468 ) ) ;
#7477=CARTESIAN_POINT ( 'NONE',  ( -61.73205080756886076, 14.52008544963257286, 0.5000000000000014433 ) ) ;
#7479=CARTESIAN_POINT ( 'NONE',  ( -60.99999999999998579, 13.77083333333333215, 0.9226497308103762673 ) ) ;
#7480=CARTESIAN_POINT ( 'NONE',  ( -62.43234176562499016, 9.307291666325268054, 2.248837904296538071 ) ) ;
#7482=CARTESIAN_POINT ( 'NONE',  ( -62.49999999999998579, 11.80208333265053611, 0.6339745962155627357 ) ) ;
#7483=CARTESIAN_POINT ( 'NONE',  ( -62.86468353124999453, 14.45312499965860020, 1.500000000000002220 ) ) ;
#7486=CARTESIAN_POINT ( 'NONE',  ( -61.99999999999998579, 12.20312499965860198, 0.5015494609379544944 ) ) ;
#7487=CARTESIAN_POINT ( 'NONE',  ( -61.99999999999998579, 16.00000000000000000, 1.500000000000002220 ) ) ;
#7491=( BOUNDED_CURVE ( )  B_SPLINE_CURVE ( 2, ( #1246, #239, #3624, #675, #9074, #3912, #4060, #7405, #579 ),
 .UNSPECIFIED., .F., .F. ) 
 B_SPLINE_CURVE_WITH_KNOTS ( ( 3, 2, 2, 2, 3 ),
 ( 0.7578125000000000000, 0.7604166666666666297, 0.7656250000000000000, 0.7708333333333333703, 0.7734375000000000000 ),
 .UNSPECIFIED. ) 
 CURVE ( )  GEOMETRIC_REPRESENTATION_ITEM ( )  RATIONAL_B_SPLINE_CURVE ( ( 0.9330127018922194093, 0.9330127018922194093, 1.000000000000000000, 0.8660254037844387076, 1.000000000000000000, 0.8660254037844387076, 1.000000000000000000, 0.9330127018922194093, 0.9330127018922194093 ) ) 
 REPRESENTATION_ITEM ( '' )  );
#7493=VERTEX_POINT ( 'NONE', #2666 ) ;
#7495=CARTESIAN_POINT ( 'NONE',  ( -61.49999999999998579, 11.54166666666666785, 0.6339745962155628467 ) ) ;
#7499=CARTESIAN_POINT ( 'NONE',  ( -61.99999999999998579, 9.656249999317200405, 2.654700538379254571 ) ) ;
#7501=CARTESIAN_POINT ( 'NONE',  ( -61.13531646874998415, 13.64062499965860198, 1.500000000000002220 ) ) ;
#7502=CARTESIAN_POINT ( 'NONE',  ( -62.49999999999998579, 10.66666666666666607, 2.366025403784441483 ) ) ;
#7503=ORIENTED_EDGE ( 'NONE', *, *, #9500, .T. ) ;
#7508=CARTESIAN_POINT ( 'NONE',  ( -62.86468353124998742, 14.72395833299193413, 1.999225269531025972 ) ) ;
#7509=CARTESIAN_POINT ( 'NONE',  ( -61.73205080756886076, 13.69866454968463110, 2.500000000000003109 ) ) ;
#7511=CARTESIAN_POINT ( 'NONE',  ( -61.99999999999998579, 16.00000000000000000, 1.500000000000002220 ) ) ;
#7512=CARTESIAN_POINT ( 'NONE',  ( -61.56765823437498142, 12.18229166632526628, 0.7511620957034663704 ) ) ;
#7513=CARTESIAN_POINT ( 'NONE',  ( -61.56765823437498852, 16.09895833299193768, 2.248837904296538515 ) ) ;
#7515=CYLINDRICAL_SURFACE ( 'NONE', #10807, 0.9999999999999981126 ) ;
#7516=CARTESIAN_POINT ( 'NONE',  ( -60.99999999999998579, 16.19791666598386826, 2.077350269189628840 ) ) ;
#7518=ORIENTED_EDGE ( 'NONE', *, *, #3408, .T. ) ;
#7520=CARTESIAN_POINT ( 'NONE',  ( -62.99999999999998579, 11.84374999931720218, 1.500000000000001998 ) ) ;
#7521=CARTESIAN_POINT ( 'NONE',  ( -60.99999999999998579, 8.020833333333332149, 0.9226497308103762673 ) ) ;
#7522=EDGE_CURVE ( 'NONE', #5087, #35, #3542, .T. ) ;
#7523=CARTESIAN_POINT ( 'NONE',  ( -61.13531646874997705, 14.55729166632526983, 1.999225269531026417 ) ) ;
#7524=CARTESIAN_POINT ( 'NONE',  ( -61.56765823437498852, 9.536458332991934128, 2.248837904296538515 ) ) ;
#7526=CARTESIAN_POINT ( 'NONE',  ( -61.13531646874998415, 15.39062499965860020, 1.500000000000002220 ) ) ;
#7527=CARTESIAN_POINT ( 'NONE',  ( -61.99999999999998579, 8.781249999317202182, 0.5000000000000013323 ) ) ;
#7529=CARTESIAN_POINT ( 'NONE',  ( -62.99999999999998579, 13.10416666666666607, 0.9226497308103756012 ) ) ;
#7530=CARTESIAN_POINT ( 'NONE',  ( -61.99999999999999289, 8.328124999658601979, 2.498450539062049724 ) ) ;
#7533=CARTESIAN_POINT ( 'NONE',  ( -62.99999999999998579, 11.82291666598387003, 0.9226497308103756012 ) ) ;
#7534=CARTESIAN_POINT ( 'NONE',  ( -61.99999999999998579, 11.28124999931720041, 0.5000000000000013323 ) ) ;
#7536=CARTESIAN_POINT ( 'NONE',  ( -61.13531646874998415, 14.32812499965860020, 1.500000000000002220 ) ) ;
#7537=CARTESIAN_POINT ( 'NONE',  ( -60.99999999999998579, 11.47916666666666785, 2.077350269189628840 ) ) ;
#7539=CARTESIAN_POINT ( 'NONE',  ( -62.43234176562499016, 13.30729166632526805, 2.248837904296538071 ) ) ;
#7541=EDGE_CURVE ( 'NONE', #6239, #4238, #6364, .T. ) ;
#7546=CARTESIAN_POINT ( 'NONE',  ( -62.99999999999998579, 11.62500000000000000, 1.500000000000001998 ) ) ;
#7548=CARTESIAN_POINT ( 'NONE',  ( -61.13531646874998415, 8.619791666325268054, 1.999225269531026417 ) ) ;
#7549=CARTESIAN_POINT ( 'NONE',  ( -61.99999999999998579, 26.00000000000000355, 4.000000000000004441 ) ) ;
#7550=EDGE_CURVE ( 'NONE', #1260, #6004, #5202, .T. ) ;
#7551=CARTESIAN_POINT ( 'NONE',  ( -61.13531646874998415, 12.89062499965860198, 1.500000000000002220 ) ) ;
#7552=CARTESIAN_POINT ( 'NONE',  ( -62.99999999999998579, 14.57291666598387003, 0.9226497308103756012 ) ) ;
#7554=( BOUNDED_CURVE ( )  B_SPLINE_CURVE ( 2, ( #6311, #4739, #8035, #9751, #5521 ),
 .UNSPECIFIED., .F., .T. ) 
 B_SPLINE_CURVE_WITH_KNOTS ( ( 3, 2, 3 ),
 ( 0.9725886266600324292, 0.9739583333333333703, 0.9765625000000000000 ),
 .UNSPECIFIED. ) 
 CURVE ( )  GEOMETRIC_REPRESENTATION_ITEM ( )  RATIONAL_B_SPLINE_CURVE ( ( 0.9480652127606670199, 0.9647668674900635732, 1.000000000000000000, 0.9330127018922194093, 0.9330127018922194093 ) ) 
 REPRESENTATION_ITEM ( '' )  );
#7556=ADVANCED_FACE ( 'NONE', ( #1279 ), #5428, .T. ) ;
#7559=CARTESIAN_POINT ( 'NONE',  ( -62.43234176562499016, 15.24479166632526805, 2.248837904296538071 ) ) ;
#7560=CARTESIAN_POINT ( 'NONE',  ( -61.99999999999998579, 11.93750000000000000, 2.500000000000002665 ) ) ;
#7561=CARTESIAN_POINT ( 'NONE',  ( -60.99999999999998579, 11.73958333265053611, 0.9226497308103762673 ) ) ;
#7563=CARTESIAN_POINT ( 'NONE',  ( -61.56765823437498852, 12.84895833299193413, 2.248837904296538515 ) ) ;
#7564=CARTESIAN_POINT ( 'NONE',  ( -62.86468353124998742, 15.28645833299193413, 1.999225269531025972 ) ) ;
#7567=CARTESIAN_POINT ( 'NONE',  ( -61.99999999999998579, 9.078124999658601979, 2.498450539062049724 ) ) ;
#7568=CYLINDRICAL_SURFACE ( 'NONE', #9093, 0.9999999999999981126 ) ;
#7572=CARTESIAN_POINT ( 'NONE',  ( -62.86468353124999453, 14.72395833299193413, 1.999225269531025750 ) ) ;
#7573=CARTESIAN_POINT ( 'NONE',  ( -61.99999999999998579, 11.01562499965859843, 2.498450539062049724 ) ) ;
#7574=CARTESIAN_POINT ( 'NONE',  ( -61.99999999999999289, 15.57812499965860198, 2.498450539062049724 ) ) ;
#7577=CARTESIAN_POINT ( 'NONE',  ( -62.49999999999998579, 14.83333333333333393, 0.6339745962155627357 ) ) ;
#7578=CARTESIAN_POINT ( 'NONE',  ( -61.56765823437498852, 8.348958332991934128, 2.248837904296538515 ) ) ;
#7579=FILL_AREA_STYLE ('',( #3146 ) ) ;
#7581=CARTESIAN_POINT ( 'NONE',  ( -62.49999999999998579, 13.13541666598387003, 2.366025403784441483 ) ) ;
#7583=CARTESIAN_POINT ( 'NONE',  ( -61.99999999999998579, 16.00000000000000000, 1.500000000000002220 ) ) ;
#7586=CARTESIAN_POINT ( 'NONE',  ( -62.43234176562498305, 14.16145833299193413, 0.7511620957034662593 ) ) ;
#7587=ORIENTED_EDGE ( 'NONE', *, *, #5031, .T. ) ;
#7589=CARTESIAN_POINT ( 'NONE',  ( -61.99999999999998579, 13.57812499965860020, 2.498450539062049724 ) ) ;
#7590=FACE_OUTER_BOUND ( 'NONE', #1278, .T. ) ;
#7592=EDGE_LOOP ( 'NONE', ( #9407, #6197, #4123, #5146 ) ) ;
#7593=PRODUCT ( 'clamp screw', 'clamp screw', '', ( #9688 ) ) ;
#7597=EDGE_CURVE ( 'NONE', #1245, #7701, #9488, .T. ) ;
#7600=CARTESIAN_POINT ( 'NONE',  ( -61.49999999999998579, 11.70833333333333215, 2.366025403784441927 ) ) ;
#7603=CARTESIAN_POINT ( 'NONE',  ( -62.86468353124999453, 8.765624999658601979, 1.500000000000002220 ) ) ;
#7606=CARTESIAN_POINT ( 'NONE',  ( -61.13531646874998415, 13.11979166632526805, 1.999225269531026417 ) ) ;
#7607=CARTESIAN_POINT ( 'NONE',  ( -62.26794919243111082, 9.395085449632572860, 2.500000000000000888 ) ) ;
#7609=CARTESIAN_POINT ( 'NONE',  ( -61.99999999999997868, 10.90624999931720218, 2.500000000000002665 ) ) ;
#7610=AXIS2_PLACEMENT_3D ( 'NONE', #7327, #2220, #3205 ) ;
#7612=CARTESIAN_POINT ( 'NONE',  ( -61.99999999999998579, 13.28124999931720041, 0.5000000000000013323 ) ) ;
#7613=CARTESIAN_POINT ( 'NONE',  ( -61.56765823437498852, 15.28645833299193590, 2.248837904296538515 ) ) ;
#7615=CARTESIAN_POINT ( 'NONE',  ( -62.26794919243111082, 11.92633545031536890, 2.500000000000003109 ) ) ;
#7617=CARTESIAN_POINT ( 'NONE',  ( -61.49999999999998579, 10.70833333333333393, 2.366025403784441927 ) ) ;
#7618=CARTESIAN_POINT ( 'NONE',  ( -62.86468353124998032, 12.99479166632526805, 1.000774730468978024 ) ) ;
#7619=CARTESIAN_POINT ( 'NONE',  ( -61.13531646874998415, 9.348958332991935904, 1.000774730468978468 ) ) ;
#7620=FACE_OUTER_BOUND ( 'NONE', #8539, .T. ) ;
#7621=( BOUNDED_CURVE ( )  B_SPLINE_CURVE ( 2, ( #5171, #8633, #7694, #3401, #75, #1071, #958, #1012, #4459 ),
 .UNSPECIFIED., .F., .T. ) 
 B_SPLINE_CURVE_WITH_KNOTS ( ( 3, 2, 2, 2, 3 ),
 ( 0.6328125000000000000, 0.6354166666666666297, 0.6406250000000000000, 0.6458333333333333703, 0.6484375000000000000 ),
 .UNSPECIFIED. ) 
 CURVE ( )  GEOMETRIC_REPRESENTATION_ITEM ( )  RATIONAL_B_SPLINE_CURVE ( ( 0.9330127018922194093, 0.9330127018922194093, 1.000000000000000000, 0.8660254037844387076, 1.000000000000000000, 0.8660254037844387076, 1.000000000000000000, 0.9330127018922194093, 0.9330127018922194093 ) ) 
 REPRESENTATION_ITEM ( '' )  );
#7622=CARTESIAN_POINT ( 'NONE',  ( -61.99999999999998579, 9.406249999317202182, 2.500000000000002665 ) ) ;
#7623=CARTESIAN_POINT ( 'NONE',  ( -62.86468353124999453, 8.765624999658601979, 1.500000000000002220 ) ) ;
#7624=DIRECTION ( 'NONE',  ( 0.000000000000000000, -0.000000000000000000, 1.000000000000000000 ) ) ;
#7626=DIRECTION ( 'NONE',  ( -0.000000000000000000, -1.000000000000000000, -0.000000000000000000 ) ) ;
#7629=CARTESIAN_POINT ( 'NONE',  ( -62.43234176562499016, 15.49479166632526628, 2.248837904296538071 ) ) ;
#7630=CARTESIAN_POINT ( 'NONE',  ( -61.56765823437498852, 10.78645833299193413, 2.248837904296538515 ) ) ;
#7631=CARTESIAN_POINT ( 'NONE',  ( -62.86468353124999453, 15.76562499965860198, 1.500000000000002220 ) ) ;
#7632=CARTESIAN_POINT ( 'NONE',  ( -61.99999999999997868, 9.656249999317202182, 2.500000000000002665 ) ) ;
#7633=ORIENTED_EDGE ( 'NONE', *, *, #8375, .T. ) ;
#7634=CARTESIAN_POINT ( 'NONE',  ( -61.49999999999998579, 14.70833333333333393, 2.366025403784441927 ) ) ;
#7639=CARTESIAN_POINT ( 'NONE',  ( -61.99999999999998579, 13.90624999931720218, 2.654700538379254571 ) ) ;
#7642=CARTESIAN_POINT ( 'NONE',  ( -61.13531646874997705, 11.09895833299193590, 1.000774730468978468 ) ) ;
#7644=ORIENTED_EDGE ( 'NONE', *, *, #4417, .F. ) ;
#7647=CARTESIAN_POINT ( 'NONE',  ( -61.56765823437498852, 12.84895833299193413, 2.248837904296538515 ) ) ;
#7651=ORIENTED_EDGE ( 'NONE', *, *, #9211, .F. ) ;
#7654=ORIENTED_EDGE ( 'NONE', *, *, #1614, .F. ) ;
#7657=CARTESIAN_POINT ( 'NONE',  ( -61.13531646874998415, 8.390624999658601979, 1.500000000000002220 ) ) ;
#7658=CARTESIAN_POINT ( 'NONE',  ( -60.99999999999998579, 14.27083333333333393, 0.9226497308103762673 ) ) ;
#7660=EDGE_CURVE ( 'NONE', #7344, #6810, #10602, .T. ) ;
#7661=CARTESIAN_POINT ( 'NONE',  ( -62.43234176562498305, 13.47395833299193413, 0.7511620957034662593 ) ) ;
#7663=ORIENTED_EDGE ( 'NONE', *, *, #6789, .T. ) ;
#7664=AXIS2_PLACEMENT_3D ( 'NONE', #737, #1521, #5738 ) ;
#7665=CARTESIAN_POINT ( 'NONE',  ( -61.99999999999998579, 16.00000000000000000, 2.500000000000000444 ) ) ;
#7667=VERTEX_POINT ( 'NONE', #1040 ) ;
#7668=CARTESIAN_POINT ( 'NONE',  ( -61.73205080756886076, 13.16741454900183328, 2.500000000000003109 ) ) ;
#7669=CARTESIAN_POINT ( 'NONE',  ( -61.99999999999998579, 15.51562499965860198, 2.498450539062049724 ) ) ;
#7671=DIRECTION ( 'NONE',  ( -0.000000000000000000, -1.000000000000000000, -0.000000000000000000 ) ) ;
#7672=CARTESIAN_POINT ( 'NONE',  ( -62.49999999999998579, 8.833333333333333925, 0.6339745962155627357 ) ) ;
#7673=VECTOR ( 'NONE', #2771, 1000.000000000000000 ) ;
#7674=CARTESIAN_POINT ( 'NONE',  ( -62.86468353124999453, 12.26562499965860198, 1.500000000000002220 ) ) ;
#7676=CARTESIAN_POINT ( 'NONE',  ( -61.99999999999998579, 8.265624999658601979, 2.498450539062049724 ) ) ;
#7677=FACE_OUTER_BOUND ( 'NONE', #10888, .T. ) ;
#7678=CARTESIAN_POINT ( 'NONE',  ( -61.99999999999998579, 16.00000000000000000, 1.500000000000002220 ) ) ;
#7679=CARTESIAN_POINT ( 'NONE',  ( -62.86468353124999453, 9.515624999658600203, 1.500000000000002220 ) ) ;
#7680=CARTESIAN_POINT ( 'NONE',  ( -62.26794919243111082, 14.04241454900183328, 0.5000000000000013323 ) ) ;
#7683=CARTESIAN_POINT ( 'NONE',  ( -61.49999999999998579, 12.92708333265053611, 2.366025403784441927 ) ) ;
#7684=CARTESIAN_POINT ( 'NONE',  ( -61.99999999999999289, 16.01562499965860198, 2.498450539062049724 ) ) ;
#7685=CARTESIAN_POINT ( 'NONE',  ( -61.13531646874998415, 10.57812499965860198, 1.500000000000002220 ) ) ;
#7686=CARTESIAN_POINT ( 'NONE',  ( -61.13531646874998415, 15.64062499965860198, 1.500000000000002220 ) ) ;
#7687=CARTESIAN_POINT ( 'NONE',  ( -61.99999999999998579, 13.03124999931720218, 0.5000000000000013323 ) ) ;
#7688=( BOUNDED_CURVE ( )  B_SPLINE_CURVE ( 2, ( #7835, #4368, #3659, #3605, #1836, #2777, #7895, #5994, #3548 ),
 .UNSPECIFIED., .F., .T. ) 
 B_SPLINE_CURVE_WITH_KNOTS ( ( 3, 2, 2, 2, 3 ),
 ( 0.2265625000000000000, 0.2291666666666666574, 0.2343750000000000000, 0.2395833333333333426, 0.2421875000000000000 ),
 .UNSPECIFIED. ) 
 CURVE ( )  GEOMETRIC_REPRESENTATION_ITEM ( )  RATIONAL_B_SPLINE_CURVE ( ( 0.9330127018922194093, 0.9330127018922194093, 1.000000000000000000, 0.8660254037844387076, 1.000000000000000000, 0.8660254037844387076, 1.000000000000000000, 0.9330127018922194093, 0.9330127018922194093 ) ) 
 REPRESENTATION_ITEM ( '' )  );
#7690=CARTESIAN_POINT ( 'NONE',  ( -61.99999999999998579, 15.06250000000000000, 0.3452994616207497591 ) ) ;
#7691=CARTESIAN_POINT ( 'NONE',  ( -61.99999999999999289, 9.203124999658601979, 0.5015494609379544944 ) ) ;
#7693=CARTESIAN_POINT ( 'NONE',  ( -62.49999999999998579, 13.63541666598387003, 2.366025403784441483 ) ) ;
#7694=CARTESIAN_POINT ( 'NONE',  ( -62.49999999999998579, 13.08333333333333215, 0.6339745962155627357 ) ) ;
#7695=ORIENTED_EDGE ( 'NONE', *, *, #1166, .T. ) ;
#7696=EDGE_CURVE ( 'NONE', #4700, #827, #8216, .T. ) ;
#7697=CARTESIAN_POINT ( 'NONE',  ( -60.99999999999998579, 9.750000000000000000, 1.500000000000002220 ) ) ;
#7698=CARTESIAN_POINT ( 'NONE',  ( -62.43234176562499016, 11.24479166632526805, 2.248837904296538071 ) ) ;
#7701=VERTEX_POINT ( 'NONE', #6103 ) ;
#7702=CARTESIAN_POINT ( 'NONE',  ( -61.99999999999998579, 12.93750000000000000, 2.500000000000002665 ) ) ;
#7703=CARTESIAN_POINT ( 'NONE',  ( -61.56765823437498142, 12.93229166632526805, 0.7511620957034663704 ) ) ;
#7706=CARTESIAN_POINT ( 'NONE',  ( -61.49999999999998579, 9.927083332650536107, 2.366025403784441927 ) ) ;
#7710=CARTESIAN_POINT ( 'NONE',  ( -61.49999999999998579, 14.79166666666666607, 0.6339745962155628467 ) ) ;
#7711=CARTESIAN_POINT ( 'NONE',  ( -61.13531646874998415, 11.82812499965860198, 1.500000000000002220 ) ) ;
#7714=CARTESIAN_POINT ( 'NONE',  ( -62.86468353124998742, 8.786458332991934128, 1.999225269531025972 ) ) ;
#7715=CARTESIAN_POINT ( 'NONE',  ( -61.49999999999998579, 14.29166666666666785, 0.6339745962155628467 ) ) ;
#7716=( BOUNDED_CURVE ( )  B_SPLINE_CURVE ( 2, ( #4496, #3841, #6233, #226, #3787, #400, #2903, #8075, #2010 ),
 .UNSPECIFIED., .F., .F. ) 
 B_SPLINE_CURVE_WITH_KNOTS ( ( 3, 2, 2, 2, 3 ),
 ( 0.3828124999999999445, 0.3854166666666666852, 0.3906250000000000000, 0.3958333333333333148, 0.3984375000000000000 ),
 .UNSPECIFIED. ) 
 CURVE ( )  GEOMETRIC_REPRESENTATION_ITEM ( )  RATIONAL_B_SPLINE_CURVE ( ( 0.9330127018922192983, 0.9330127018922178550, 1.000000000000000000, 0.8660254037844387076, 1.000000000000000000, 0.8660254037844387076, 1.000000000000000000, 0.9330127018922194093, 0.9330127018922194093 ) ) 
 REPRESENTATION_ITEM ( '' )  );
#7717=EDGE_CURVE ( 'NONE', #2979, #5370, #2892, .T. ) ;
#7718=CARTESIAN_POINT ( 'NONE',  ( -61.13531646874998415, 13.14062499965860198, 1.500000000000002220 ) ) ;
#7721=DIRECTION ( 'NONE',  ( -0.000000000000000000, -1.000000000000000000, -0.000000000000000000 ) ) ;
#7724=CARTESIAN_POINT ( 'NONE',  ( -61.99999999999998579, 11.53124999931720218, 0.5000000000000013323 ) ) ;
#7725=CARTESIAN_POINT ( 'NONE',  ( -61.99999999999998579, 14.89062499965860020, 0.5015494609379544944 ) ) ;
#7726=CARTESIAN_POINT ( 'NONE',  ( -62.26794919243111082, 8.895085449632571084, 2.500000000000003109 ) ) ;
#7729=CARTESIAN_POINT ( 'NONE',  ( -62.86468353124998032, 14.24479166632526983, 1.000774730468978024 ) ) ;
#7730=CARTESIAN_POINT ( 'NONE',  ( -62.86468353124998032, 8.432291666325266277, 1.000774730468978246 ) ) ;
#7731=DIRECTION ( 'NONE',  ( -0.000000000000000000, -1.000000000000000000, -0.000000000000000000 ) ) ;
#7733=CARTESIAN_POINT ( 'NONE',  ( -61.99999999999998579, 8.578124999658601979, 2.498450539062049724 ) ) ;
#7734=CARTESIAN_POINT ( 'NONE',  ( -61.99999999999998579, 10.06250000000000000, 0.5000000000000013323 ) ) ;
#7738=CARTESIAN_POINT ( 'NONE',  ( -61.13531646874997705, 15.84895833299193590, 1.000774730468978468 ) ) ;
#7739=EDGE_CURVE ( 'NONE', #4700, #8255, #10430, .T. ) ;
#7740=CARTESIAN_POINT ( 'NONE',  ( -61.13531646874998415, 10.82812499965860020, 1.500000000000002220 ) ) ;
#7742=CARTESIAN_POINT ( 'NONE',  ( -61.56765823437498142, 8.619791666325268054, 0.7511620957034663704 ) ) ;
#7745=CARTESIAN_POINT ( 'NONE',  ( -60.99999999999998579, 15.75000000000000000, 1.500000000000002220 ) ) ;
#7746=CARTESIAN_POINT ( 'NONE',  ( -62.86468353124998032, 9.494791666325268054, 1.000774730468978024 ) ) ;
#7747=CARTESIAN_POINT ( 'NONE',  ( -62.99999999999998579, 13.36458333265053433, 2.077350269189627952 ) ) ;
#7750=CARTESIAN_POINT ( 'NONE',  ( -62.49999999999998579, 11.66666666666666785, 2.366025403784441483 ) ) ;
#7751=CARTESIAN_POINT ( 'NONE',  ( -61.99999999999999289, 11.26562499965860020, 2.498450539062049724 ) ) ;
#7755=VERTEX_POINT ( 'NONE', #2274 ) ;
#7756=CARTESIAN_POINT ( 'NONE',  ( -62.26794919243111082, 12.82366454968462932, 0.5000000000000013323 ) ) ;
#7757=CARTESIAN_POINT ( 'NONE',  ( -62.86468353124998032, 12.74479166632526805, 1.000774730468978246 ) ) ;
#7758=CARTESIAN_POINT ( 'NONE',  ( -61.99999999999998579, 10.93750000000000000, 2.500000000000002665 ) ) ;
#7759=CARTESIAN_POINT ( 'NONE',  ( -62.99999999999998579, 9.093749999317203958, 1.500000000000001998 ) ) ;
#7764=CARTESIAN_POINT ( 'NONE',  ( -61.99999999999998579, 15.28124999931720218, 0.5000000000000013323 ) ) ;
#7765=CARTESIAN_POINT ( 'NONE',  ( -61.56765823437498852, 11.28645833299193590, 2.248837904296538515 ) ) ;
#7767=ORIENTED_EDGE ( 'NONE', *, *, #8905, .F. ) ;
#7769=CARTESIAN_POINT ( 'NONE',  ( -61.56765823437498852, 8.848958332991934128, 2.248837904296538515 ) ) ;
#7771=CARTESIAN_POINT ( 'NONE',  ( -61.56765823437498142, 13.93229166632526805, 0.7511620957034663704 ) ) ;
#7772=CARTESIAN_POINT ( 'NONE',  ( -62.99999999999998579, 9.364583332650536107, 2.077350269189627952 ) ) ;
#7775=CIRCLE ( 'NONE', #9919, 2.500000000000002220 ) ;
#7777=ORIENTED_EDGE ( 'NONE', *, *, #320, .F. ) ;
#7778=CARTESIAN_POINT ( 'NONE',  ( -61.99999999999998579, 10.81250000000000000, 0.5000000000000013323 ) ) ;
#7779=CARTESIAN_POINT ( 'NONE',  ( -62.49999999999998579, 8.666666666666666075, 2.366025403784441483 ) ) ;
#7780=DIRECTION ( 'NONE',  ( 0.000000000000000000, 0.000000000000000000, -1.000000000000000000 ) ) ;
#7782=( BOUNDED_CURVE ( )  B_SPLINE_CURVE ( 2, ( #9000, #3267, #660, #507, #7444, #3942, #1443, #8230, #5659 ),
 .UNSPECIFIED., .F., .T. ) 
 B_SPLINE_CURVE_WITH_KNOTS ( ( 3, 2, 2, 2, 3 ),
 ( 0.05468749999999996531, 0.05729166666666666435, 0.06250000000000000000, 0.06770833333333332871, 0.07031250000000001388 ),
 .UNSPECIFIED. ) 
 CURVE ( )  GEOMETRIC_REPRESENTATION_ITEM ( )  RATIONAL_B_SPLINE_CURVE ( ( 0.9330127018922194093, 0.9330127018922185211, 1.000000000000000000, 0.8660254037844387076, 1.000000000000000000, 0.8660254037844387076, 1.000000000000000000, 0.9330127018922189652, 0.9330127018922192983 ) ) 
 REPRESENTATION_ITEM ( '' )  );
#7784=CARTESIAN_POINT ( 'NONE',  ( -61.99999999999999289, 13.57812499965860198, 2.498450539062049724 ) ) ;
#7785=CARTESIAN_POINT ( 'NONE',  ( -62.86468353124998032, 9.432291666325268054, 1.000774730468978246 ) ) ;
#7787=CARTESIAN_POINT ( 'NONE',  ( -61.49999999999998579, 9.291666666666666075, 0.6339745962155628467 ) ) ;
#7789=CARTESIAN_POINT ( 'NONE',  ( -61.56765823437498142, 9.682291666325268054, 0.7511620957034663704 ) ) ;
#7790=AXIS2_PLACEMENT_3D ( 'NONE', #1841, #1894, #2730 ) ;
#7791=CARTESIAN_POINT ( 'NONE',  ( -61.99999999999998579, 14.15624999931720218, 2.500000000000002665 ) ) ;
#7792=ORIENTED_EDGE ( 'NONE', *, *, #9135, .T. ) ;
#7794=CARTESIAN_POINT ( 'NONE',  ( -61.99999999999997868, 11.28124999931720041, 0.5000000000000013323 ) ) ;
#7795=CARTESIAN_POINT ( 'NONE',  ( -61.13531646874997705, 15.05729166632526805, 1.999225269531026417 ) ) ;
#7796=CARTESIAN_POINT ( 'NONE',  ( -62.43234176562499016, 11.24479166632526805, 2.248837904296538071 ) ) ;
#7797=CARTESIAN_POINT ( 'NONE',  ( -61.56765823437498852, 8.536458332991934128, 2.248837904296538515 ) ) ;
#7801=CARTESIAN_POINT ( 'NONE',  ( -61.99999999999998579, 15.31250000000000000, 0.3452994616207497591 ) ) ;
#7802=CARTESIAN_POINT ( 'NONE',  ( -61.99999999999999289, 9.578124999658600203, 2.498450539062049724 ) ) ;
#7804=CARTESIAN_POINT ( 'NONE',  ( -62.99999999999998579, 13.57291666598387359, 0.9226497308103756012 ) ) ;
#7805=CARTESIAN_POINT ( 'NONE',  ( -61.99999999999998579, 8.906249999317202182, 2.500000000000002665 ) ) ;
#7810=CARTESIAN_POINT ( 'NONE',  ( -61.13531646874997705, 12.09895833299193235, 1.000774730468978468 ) ) ;
#7814=CARTESIAN_POINT ( 'NONE',  ( -61.99999999999998579, 10.93750000000000000, 2.654700538379254571 ) ) ;
#7815=CARTESIAN_POINT ( 'NONE',  ( -62.99999999999998579, 10.10416666666666785, 0.9226497308103756012 ) ) ;
#7816=CARTESIAN_POINT ( 'NONE',  ( -61.13531646874998415, 13.89062499965860198, 1.500000000000002220 ) ) ;
#7818=CARTESIAN_POINT ( 'NONE',  ( -62.99999999999998579, 9.114583332650537884, 2.077350269189627952 ) ) ;
#7822=CARTESIAN_POINT ( 'NONE',  ( -61.99999999999998579, 11.01562499965859843, 2.498450539062049724 ) ) ;
#7824=CARTESIAN_POINT ( 'NONE',  ( -61.13531646874998415, 10.66145833299193413, 1.000774730468978468 ) ) ;
#7825=CARTESIAN_POINT ( 'NONE',  ( -62.99999999999998579, 15.59374999931720218, 1.500000000000001998 ) ) ;
#7826=CARTESIAN_POINT ( 'NONE',  ( -61.99999999999998579, 14.70312499965860020, 0.5015494609379544944 ) ) ;
#7827=CARTESIAN_POINT ( 'NONE',  ( -61.49999999999998579, 8.260416665983870033, 0.6339745962155628467 ) ) ;
#7829=DIRECTION ( 'NONE',  ( -0.000000000000000000, -1.000000000000000000, -0.000000000000000000 ) ) ;
#7832=CARTESIAN_POINT ( 'NONE',  ( -61.49999999999998579, 12.76041666598386826, 0.6339745962155628467 ) ) ;
#7833=ADVANCED_FACE ( 'NONE', ( #10766 ), #2325, .T. ) ;
#7834=CARTESIAN_POINT ( 'NONE',  ( -62.43234176562498305, 15.91145833299193590, 0.7511620957034662593 ) ) ;
#7835=CARTESIAN_POINT ( 'NONE',  ( -61.99999999999998579, 9.812500000000000000, 0.5000000000000013323 ) ) ;
#7838=CARTESIAN_POINT ( 'NONE',  ( -62.43234176562498305, 14.47395833299193413, 0.7511620957034662593 ) ) ;
#7839=CARTESIAN_POINT ( 'NONE',  ( -62.43234176562499016, 9.244791666325268054, 2.248837904296538071 ) ) ;
#7840=CARTESIAN_POINT ( 'NONE',  ( -61.99999999999998579, 16.00000000000000000, 1.500000000000002220 ) ) ;
#7841=CARTESIAN_POINT ( 'NONE',  ( -62.99999999999998579, 9.625000000000000000, 1.500000000000001998 ) ) ;
#7843=CARTESIAN_POINT ( 'NONE',  ( -61.13531646874998415, 10.61979166632526983, 1.999225269531026417 ) ) ;
#7844=FACE_OUTER_BOUND ( 'NONE', #9018, .T. ) ;
#7847=CARTESIAN_POINT ( 'NONE',  ( -61.49999999999998579, 13.01041666598386826, 0.6339745962155628467 ) ) ;
#7848=( BOUNDED_CURVE ( )  B_SPLINE_CURVE ( 2, ( #7687, #2740, #4227, #5221, #10175, #5957, #8574, #10222, #2624 ),
 .UNSPECIFIED., .F., .T. ) 
 B_SPLINE_CURVE_WITH_KNOTS ( ( 3, 2, 2, 2, 3 ),
 ( 0.6015625000000000000, 0.6041666666666666297, 0.6093750000000000000, 0.6145833333333333703, 0.6171875000000000000 ),
 .UNSPECIFIED. ) 
 CURVE ( )  GEOMETRIC_REPRESENTATION_ITEM ( )  RATIONAL_B_SPLINE_CURVE ( ( 0.9330127018922194093, 0.9330127018922194093, 1.000000000000000000, 0.8660254037844387076, 1.000000000000000000, 0.8660254037844387076, 1.000000000000000000, 0.9330127018922194093, 0.9330127018922194093 ) ) 
 REPRESENTATION_ITEM ( '' )  );
#7850=CARTESIAN_POINT ( 'NONE',  ( -62.86468353124998032, 15.18229166632526805, 1.000774730468978024 ) ) ;
#7851=CARTESIAN_POINT ( 'NONE',  ( -62.43234176562498305, 12.66145833299193413, 0.7511620957034662593 ) ) ;
#7853=CARTESIAN_POINT ( 'NONE',  ( -61.99999999999999289, 8.515624999658601979, 2.498450539062049724 ) ) ;
#7856=CARTESIAN_POINT ( 'NONE',  ( -61.73205080756884655, 8.520085449632571084, 0.4999999999999994449 ) ) ;
#7857=CARTESIAN_POINT ( 'NONE',  ( -61.13531646874997705, 9.411458332991935904, 1.000774730468978468 ) ) ;
#7859=CARTESIAN_POINT ( 'NONE',  ( -61.13531646874998415, 15.84895833299193413, 1.000774730468978468 ) ) ;
#7860=CARTESIAN_POINT ( 'NONE',  ( -62.49999999999998579, 15.05208333265053611, 0.6339745962155627357 ) ) ;
#7862=ORIENTED_EDGE ( 'NONE', *, *, #602, .F. ) ;
#7868=CARTESIAN_POINT ( 'NONE',  ( -62.43234176562499016, 11.99479166632526628, 2.248837904296538071 ) ) ;
#7869=CARTESIAN_POINT ( 'NONE',  ( -61.99999999999998579, 8.265624999658601979, 2.498450539062049724 ) ) ;
#7872=CARTESIAN_POINT ( 'NONE',  ( -61.99999999999998579, 10.56250000000000000, 0.3452994616207497591 ) ) ;
#7874=EDGE_CURVE ( 'NONE', #2754, #9906, #613, .T. ) ;
#7875=CARTESIAN_POINT ( 'NONE',  ( -62.86468353124998742, 14.03645833299193590, 1.999225269531025972 ) ) ;
#7876=CARTESIAN_POINT ( 'NONE',  ( -62.49999999999998579, 13.83333333333333215, 0.6339745962155627357 ) ) ;
#7877=CARTESIAN_POINT ( 'NONE',  ( -60.99999999999998579, 8.968749999317203958, 1.500000000000002220 ) ) ;
#7879=EDGE_LOOP ( 'NONE', ( #763, #8809, #3416, #10374 ) ) ;
#7883=CARTESIAN_POINT ( 'NONE',  ( -62.86468353124999453, 10.70312499965860020, 1.500000000000002220 ) ) ;
#7887=CARTESIAN_POINT ( 'NONE',  ( -61.13531646874998415, 9.869791666325269830, 1.999225269531026417 ) ) ;
#7888=CARTESIAN_POINT ( 'NONE',  ( -61.99999999999998579, 15.90624999931719863, 2.500000000000002665 ) ) ;
#7889=CARTESIAN_POINT ( 'NONE',  ( -61.99999999999998579, 14.82812499965860020, 2.498450539062049724 ) ) ;
#7893=ORIENTED_EDGE ( 'NONE', *, *, #646, .F. ) ;
#7894=CARTESIAN_POINT ( 'NONE',  ( -60.99999999999998579, 8.729166666666666075, 2.077350269189628840 ) ) ;
#7895=CARTESIAN_POINT ( 'NONE',  ( -62.49999999999998579, 9.916666666666667851, 2.366025403784441483 ) ) ;
#7897=EDGE_CURVE ( 'NONE', #5429, #1066, #9055, .T. ) ;
#7899=CARTESIAN_POINT ( 'NONE',  ( -61.13531646874998415, 13.64062499965860198, 1.500000000000002220 ) ) ;
#7900=CARTESIAN_POINT ( 'NONE',  ( -61.56765823437498142, 10.61979166632526805, 0.7511620957034663704 ) ) ;
#7901=CARTESIAN_POINT ( 'NONE',  ( -61.99999999999998579, 11.56250000000000000, 0.5000000000000013323 ) ) ;
#7902=LINE ( 'NONE', #7179, #2643 ) ;
#7903=CARTESIAN_POINT ( 'NONE',  ( -62.86468353124998032, 10.74479166632526628, 1.000774730468978246 ) ) ;
#7904=ORIENTED_EDGE ( 'NONE', *, *, #3790, .T. ) ;
#7907=CARTESIAN_POINT ( 'NONE',  ( -61.49999999999998579, 11.17708333265053611, 2.366025403784441927 ) ) ;
#7908=CARTESIAN_POINT ( 'NONE',  ( -61.73205080756886076, 10.05133545031537068, 0.5000000000000014433 ) ) ;
#7909=CARTESIAN_POINT ( 'NONE',  ( -61.99999999999998579, 12.51562499965860198, 2.498450539062049724 ) ) ;
#7910=CARTESIAN_POINT ( 'NONE',  ( -61.13531646874998415, 9.078124999658601979, 1.500000000000002220 ) ) ;
#7913=CARTESIAN_POINT ( 'NONE',  ( -62.99999999999998579, 10.86458333265053611, 2.077350269189627952 ) ) ;
#7914=CARTESIAN_POINT ( 'NONE',  ( -62.86468353124999453, 10.01562499965860198, 1.500000000000002220 ) ) ;
#7916=CARTESIAN_POINT ( 'NONE',  ( -61.99999999999998579, 15.51562499965860198, 2.498450539062049724 ) ) ;
#7917=CARTESIAN_POINT ( 'NONE',  ( -62.99999999999998579, 14.36458333265053611, 2.077350269189627952 ) ) ;
#7918=CARTESIAN_POINT ( 'NONE',  ( -61.99999999999998579, 14.68750000000000000, 2.500000000000002665 ) ) ;
#7919=VERTEX_POINT ( 'NONE', #2375 ) ;
#7920=FACE_OUTER_BOUND ( 'NONE', #8894, .T. ) ;
#7922=( BOUNDED_CURVE ( )  B_SPLINE_CURVE ( 2, ( #1554, #5616, #7399, #10778, #3170, #9008, #9955, #1402, #4882 ),
 .UNSPECIFIED., .F., .T. ) 
 B_SPLINE_CURVE_WITH_KNOTS ( ( 3, 2, 2, 2, 3 ),
 ( 0.1171875000000000278, 0.1197916666666666713, 0.1250000000000000000, 0.1302083333333333426, 0.1328125000000000000 ),
 .UNSPECIFIED. ) 
 CURVE ( )  GEOMETRIC_REPRESENTATION_ITEM ( )  RATIONAL_B_SPLINE_CURVE ( ( 0.9330127018922194093, 0.9330127018922200755, 1.000000000000000000, 0.8660254037844387076, 1.000000000000000000, 0.8660254037844387076, 1.000000000000000000, 0.9330127018922194093, 0.9330127018922194093 ) ) 
 REPRESENTATION_ITEM ( '' )  );
#7923=CARTESIAN_POINT ( 'NONE',  ( -61.56765823437498852, 12.53645833299193413, 2.248837904296538515 ) ) ;
#7924=CARTESIAN_POINT ( 'NONE',  ( -61.13531646874998415, 8.328124999658601979, 1.500000000000002220 ) ) ;
#7925=DIRECTION ( 'NONE',  ( 0.000000000000000000, 1.000000000000000000, 0.000000000000000000 ) ) ;
#7926=EDGE_LOOP ( 'NONE', ( #3777, #4207, #7224 ) ) ;
#7927=CARTESIAN_POINT ( 'NONE',  ( -62.49999999999998579, 11.91666666666666607, 2.366025403784441483 ) ) ;
#7928=CARTESIAN_POINT ( 'NONE',  ( -62.49999999999998579, 10.08333333333333215, 0.6339745962155627357 ) ) ;
#7929=CARTESIAN_POINT ( 'NONE',  ( -62.86468353124998742, 14.78645833299193413, 1.999225269531025972 ) ) ;
#7931=CARTESIAN_POINT ( 'NONE',  ( -61.99999999999998579, 13.43749999999999822, 2.500000000000002665 ) ) ;
#7932=CARTESIAN_POINT ( 'NONE',  ( -61.49999999999998579, 10.17708333265053611, 2.366025403784441927 ) ) ;
#7935=CARTESIAN_POINT ( 'NONE',  ( -61.99999999999998579, 11.15624999931720218, 2.500000000000002665 ) ) ;
#7937=CARTESIAN_POINT ( 'NONE',  ( -62.43234176562499016, 11.74479166632526805, 2.248837904296538071 ) ) ;
#7939=CARTESIAN_POINT ( 'NONE',  ( -62.43234176562498305, 10.72395833299193413, 0.7511620957034662593 ) ) ;
#7941=CARTESIAN_POINT ( 'NONE',  ( -61.56765823437498852, 13.84895833299193413, 2.248837904296538515 ) ) ;
#7943=EDGE_LOOP ( 'NONE', ( #6888, #8736, #4355, #9225 ) ) ;
#7944=CARTESIAN_POINT ( 'NONE',  ( -61.73205080756886076, 10.55133545031537068, 0.5000000000000014433 ) ) ;
#7945=ADVANCED_FACE ( 'NONE', ( #6393 ), #9780, .T. ) ;
#7948=CARTESIAN_POINT ( 'NONE',  ( -62.99999999999998579, 15.09374999931720218, 1.500000000000001998 ) ) ;
#7949=CARTESIAN_POINT ( 'NONE',  ( -62.99999999999998579, 8.604166666666666075, 0.9226497308103756012 ) ) ;
#7951=CARTESIAN_POINT ( 'NONE',  ( -61.73205080756886076, 16.16741454900183328, 2.500000000000003109 ) ) ;
#7953=CARTESIAN_POINT ( 'NONE',  ( -62.43234176562499016, 13.55729166632526805, 2.248837904296538071 ) ) ;
#7954=CARTESIAN_POINT ( 'NONE',  ( -61.99999999999998579, 10.26562499965860376, 2.498450539062049724 ) ) ;
#7956=CARTESIAN_POINT ( 'NONE',  ( -61.49999999999998579, 11.92708333265053611, 2.366025403784441927 ) ) ;
#7958=CARTESIAN_POINT ( 'NONE',  ( -61.56765823437498852, 10.09895833299193413, 2.248837904296538515 ) ) ;
#7959=CARTESIAN_POINT ( 'NONE',  ( -62.26794919243111082, 12.17633545031537068, 2.500000000000003109 ) ) ;
#7960=ORIENTED_EDGE ( 'NONE', *, *, #7717, .T. ) ;
#7961=CARTESIAN_POINT ( 'NONE',  ( -60.99999999999998579, 13.98958333265053611, 0.9226497308103762673 ) ) ;
#7963=AXIS2_PLACEMENT_3D ( 'NONE', #6993, #2943, #10371 ) ;
#7965=CARTESIAN_POINT ( 'NONE',  ( -61.99999999999998579, 10.06250000000000000, 0.5000000000000013323 ) ) ;
#7966=CARTESIAN_POINT ( 'NONE',  ( -61.13531646874998415, 12.34895833299193413, 1.000774730468978468 ) ) ;
#7967=VECTOR ( 'NONE', #164, 1000.000000000000000 ) ;
#7968=CARTESIAN_POINT ( 'NONE',  ( -62.86468353124999453, 9.453124999658600203, 1.500000000000002220 ) ) ;
#7969=DIRECTION ( 'NONE',  ( 0.000000000000000000, 0.000000000000000000, 1.000000000000000000 ) ) ;
#7970=ORIENTED_EDGE ( 'NONE', *, *, #4185, .T. ) ;
#7971=CARTESIAN_POINT ( 'NONE',  ( -62.99999999999998579, 15.89583333333333037, 2.077350269189627952 ) ) ;
#7972=CARTESIAN_POINT ( 'NONE',  ( -62.43234176562498305, 9.473958332991935904, 0.7511620957034662593 ) ) ;
#7974=CARTESIAN_POINT ( 'NONE',  ( -61.99999999999998579, 14.89062499965860020, 0.5015494609379544944 ) ) ;
#7975=CARTESIAN_POINT ( 'NONE',  ( -61.49999999999998579, 14.51041666598387003, 0.6339745962155628467 ) ) ;
#7981=CARTESIAN_POINT ( 'NONE',  ( -62.43234176562498305, 12.41145833299193413, 0.7511620957034662593 ) ) ;
#7982=CARTESIAN_POINT ( 'NONE',  ( -61.56765823437498142, 8.869791666325268054, 0.7511620957034663704 ) ) ;
#7984=CARTESIAN_POINT ( 'NONE',  ( -60.99999999999998579, 12.77083333333333393, 0.9226497308103762673 ) ) ;
#7988=CARTESIAN_POINT ( 'NONE',  ( -62.86468353124998742, 14.53645833299193413, 1.999225269531025972 ) ) ;
#7989=CARTESIAN_POINT ( 'NONE',  ( -62.99999999999998579, 13.89583333333333215, 2.077350269189627952 ) ) ;
#7990=CARTESIAN_POINT ( 'NONE',  ( -60.99999999999998579, 11.23958333265053788, 0.9226497308103762673 ) ) ;
#7991=ORIENTED_EDGE ( 'NONE', *, *, #10276, .T. ) ;
#7995=CARTESIAN_POINT ( 'NONE',  ( -62.86468353124998742, 12.22395833299193413, 1.999225269531025972 ) ) ;
#7998=VERTEX_POINT ( 'NONE', #10978 ) ;
#7999=CARTESIAN_POINT ( 'NONE',  ( -61.13531646874998415, 9.619791666325268054, 1.999225269531026417 ) ) ;
#8001=CARTESIAN_POINT ( 'NONE',  ( -62.86468353124998032, 13.99479166632526983, 1.000774730468978246 ) ) ;
#8005=EDGE_CURVE ( 'NONE', #918, #8888, #1810, .T. ) ;
#8008=CARTESIAN_POINT ( 'NONE',  ( -62.49999999999998579, 8.333333333333333925, 0.6339745962155627357 ) ) ;
#8009=CARTESIAN_POINT ( 'NONE',  ( -61.99999999999998579, 16.00000000000000000, 2.500000000000000444 ) ) ;
#8011=DIRECTION ( 'NONE',  ( 0.000000000000000000, 0.000000000000000000, 1.000000000000000000 ) ) ;
#8012=CARTESIAN_POINT ( 'NONE',  ( -62.43234176562498305, 14.97395833299193590, 0.7511620957034662593 ) ) ;
#8013=ADVANCED_FACE ( 'NONE', ( #5135 ), #6765, .T. ) ;
#8014=CARTESIAN_POINT ( 'NONE',  ( -62.86468353124998742, 9.973958332991932352, 1.999225269531025972 ) ) ;
#8015=CARTESIAN_POINT ( 'NONE',  ( -62.49999999999998579, 9.583333333333332149, 0.6339745962155627357 ) ) ;
#8016=CARTESIAN_POINT ( 'NONE',  ( -61.56765823437498852, 11.09895833299193590, 2.248837904296538515 ) ) ;
#8017=FACE_OUTER_BOUND ( 'NONE', #1661, .T. ) ;
#8019=CARTESIAN_POINT ( 'NONE',  ( -62.26794919243111082, 14.42633545031536890, 2.500000000000003109 ) ) ;
#8021=VERTEX_POINT ( 'NONE', #9366 ) ;
#8022=CARTESIAN_POINT ( 'NONE',  ( -62.26794919243111082, 10.39508544963257286, 2.500000000000003109 ) ) ;
#8023=CARTESIAN_POINT ( 'NONE',  ( -62.86468353124998032, 13.18229166632526805, 1.000774730468978246 ) ) ;
#8024=CARTESIAN_POINT ( 'NONE',  ( -62.86468353124998032, 10.68229166632526628, 1.000774730468978024 ) ) ;
#8025=DIRECTION ( 'NONE',  ( -0.000000000000000000, -1.000000000000000000, -0.000000000000000000 ) ) ;
#8027=CARTESIAN_POINT ( 'NONE',  ( -61.49999999999998579, 15.79166666666666607, 0.6339745962155628467 ) ) ;
#8028=AXIS2_PLACEMENT_3D ( 'NONE', #10215, #3556, #8508 ) ;
#8029=CARTESIAN_POINT ( 'NONE',  ( -62.43234176562498305, 11.72395833299193590, 0.7511620957034662593 ) ) ;
#8031=CARTESIAN_POINT ( 'NONE',  ( -61.56765823437498852, 15.28645833299193590, 2.248837904296538515 ) ) ;
#8032=CARTESIAN_POINT ( 'NONE',  ( -61.99999999999998579, 15.03124999931720041, 0.3452994616207497591 ) ) ;
#8033=CARTESIAN_POINT ( 'NONE',  ( -62.49999999999998579, 16.05208333265053255, 0.6339745962155627357 ) ) ;
#8035=CARTESIAN_POINT ( 'NONE',  ( -61.49999999999998579, 16.01041666598386826, 0.6339745962155628467 ) ) ;
#8038=EDGE_CURVE ( 'NONE', #7493, #1608, #5136, .T. ) ;
#8039=CARTESIAN_POINT ( 'NONE',  ( -61.99999999999999289, 13.26562499965859843, 2.498450539062049724 ) ) ;
#8040=CARTESIAN_POINT ( 'NONE',  ( -61.99999999999998579, 8.515624999658601979, 2.498450539062049724 ) ) ;
#8043=CARTESIAN_POINT ( 'NONE',  ( -60.99999999999998579, 11.77083333333333393, 0.9226497308103762673 ) ) ;
#8045=CARTESIAN_POINT ( 'NONE',  ( -62.43234176562499016, 14.55729166632526983, 2.248837904296538071 ) ) ;
#8046=ADVANCED_FACE ( 'NONE', ( #6037 ), #9421, .T. ) ;
#8047=CARTESIAN_POINT ( 'NONE',  ( -62.99999999999998579, 14.34374999931720041, 1.500000000000001998 ) ) ;
#8050=CARTESIAN_POINT ( 'NONE',  ( -62.49999999999998579, 11.05208333265053611, 0.6339745962155627357 ) ) ;
#8052=CARTESIAN_POINT ( 'NONE',  ( -61.99999999999998579, 16.00000000000000000, 1.500000000000002220 ) ) ;
#8053=EDGE_CURVE ( 'NONE', #2251, #2222, #5080, .T. ) ;
#8055=CARTESIAN_POINT ( 'NONE',  ( -61.99999999999998579, 12.64062499965860198, 0.5015494609379544944 ) ) ;
#8057=ORIENTED_EDGE ( 'NONE', *, *, #8550, .T. ) ;
#8058=CARTESIAN_POINT ( 'NONE',  ( -62.43234176562499016, 10.55729166632526983, 2.248837904296538071 ) ) ;
#8059=( BOUNDED_CURVE ( )  B_SPLINE_CURVE ( 2, ( #253, #2211, #10755, #10806, #3872, #2986, #9926, #6372, #3144 ),
 .UNSPECIFIED., .F., .T. ) 
 B_SPLINE_CURVE_WITH_KNOTS ( ( 3, 2, 2, 2, 3 ),
 ( 0.03906250000000003469, 0.04166666666666666435, 0.04687500000000000000, 0.05208333333333333565, 0.05468749999999996531 ),
 .UNSPECIFIED. ) 
 CURVE ( )  GEOMETRIC_REPRESENTATION_ITEM ( )  RATIONAL_B_SPLINE_CURVE ( ( 0.9330127018922194093, 0.9330127018922202975, 1.000000000000000000, 0.8660254037844387076, 1.000000000000000000, 0.8660254037844387076, 1.000000000000000000, 0.9330127018922202975, 0.9330127018922194093 ) ) 
 REPRESENTATION_ITEM ( '' )  );
#8065=CARTESIAN_POINT ( 'NONE',  ( -61.99999999999998579, 10.43750000000000000, 2.500000000000002665 ) ) ;
#8066=EDGE_LOOP ( 'NONE', ( #1669, #9940, #7792, #5347 ) ) ;
#8068=CARTESIAN_POINT ( 'NONE',  ( -61.99999999999998579, 12.65624999931720396, 2.500000000000002665 ) ) ;
#8069=CARTESIAN_POINT ( 'NONE',  ( -62.99999999999998579, 10.14583333333333393, 2.077350269189627952 ) ) ;
#8074=CARTESIAN_POINT ( 'NONE',  ( -61.99999999999998579, 9.765624999658600203, 2.498450539062049724 ) ) ;
#8075=CARTESIAN_POINT ( 'NONE',  ( -62.26794919243111082, 11.39508544963257108, 2.500000000000003109 ) ) ;
#8076=CARTESIAN_POINT ( 'NONE',  ( -61.73205080756886076, 15.41741454900183328, 2.500000000000003109 ) ) ;
#8077=CARTESIAN_POINT ( 'NONE',  ( -61.13531646874998415, 10.36979166632526805, 1.999225269531026417 ) ) ;
#8079=LINE ( 'NONE', #7064, #10316 ) ;
#8080=ORIENTED_EDGE ( 'NONE', *, *, #9014, .F. ) ;
#8083=CARTESIAN_POINT ( 'NONE',  ( -61.99999999999998579, 8.406249999317203958, 2.500000000000003109 ) ) ;
#8085=CARTESIAN_POINT ( 'NONE',  ( -61.49999999999998579, 15.70833333333333037, 2.366025403784441927 ) ) ;
#8086=CARTESIAN_POINT ( 'NONE',  ( -62.86468353124998032, 11.93229166632526628, 1.000774730468978246 ) ) ;
#8087=CARTESIAN_POINT ( 'NONE',  ( -61.13531646874997705, 10.30729166632526983, 1.999225269531026417 ) ) ;
#8090=CARTESIAN_POINT ( 'NONE',  ( -62.86468353124999453, 11.51562499965860020, 1.500000000000002220 ) ) ;
#8092=CARTESIAN_POINT ( 'NONE',  ( -62.86468353124999453, 15.45312499965860020, 1.500000000000002220 ) ) ;
#8093=CARTESIAN_POINT ( 'NONE',  ( -62.49999999999998579, 14.88541666598386826, 2.366025403784441483 ) ) ;
#8099=CARTESIAN_POINT ( 'NONE',  ( -62.43234176562498305, 12.66145833299193413, 0.7511620957034662593 ) ) ;
#8100=CARTESIAN_POINT ( 'NONE',  ( -62.86468353124998032, 8.682291666325268054, 1.000774730468978246 ) ) ;
#8101=CARTESIAN_POINT ( 'NONE',  ( -61.99999999999997868, 10.65624999931720218, 2.500000000000002665 ) ) ;
#8102=ORIENTED_EDGE ( 'NONE', *, *, #6750, .F. ) ;
#8103=CARTESIAN_POINT ( 'NONE',  ( -62.49999999999998579, 12.33333333333333393, 0.6339745962155627357 ) ) ;
#8104=CARTESIAN_POINT ( 'NONE',  ( -62.26794919243111082, 11.14508544963257286, 2.500000000000003109 ) ) ;
#8105=CARTESIAN_POINT ( 'NONE',  ( -61.99999999999998579, 14.40624999931720218, 2.500000000000002665 ) ) ;
#8106=CARTESIAN_POINT ( 'NONE',  ( -62.49999999999998579, 10.80208333265053611, 0.6339745962155627357 ) ) ;
#8107=EDGE_LOOP ( 'NONE', ( #3683, #9678, #7960, #6438 ) ) ;
#8109=CARTESIAN_POINT ( 'NONE',  ( -62.86468353124998032, 12.18229166632526805, 1.000774730468978246 ) ) ;
#8111=CARTESIAN_POINT ( 'NONE',  ( -61.56765823437498852, 11.59895833299193590, 2.248837904296538515 ) ) ;
#8115=CARTESIAN_POINT ( 'NONE',  ( -62.43234176562499016, 15.55729166632526628, 2.248837904296538071 ) ) ;
#8116=CARTESIAN_POINT ( 'NONE',  ( -61.49999999999998579, 9.010416665983868256, 0.6339745962155628467 ) ) ;
#8118=CARTESIAN_POINT ( 'NONE',  ( -62.99999999999998579, 11.14583333333333393, 2.077350269189627952 ) ) ;
#8119=ORIENTED_EDGE ( 'NONE', *, *, #8038, .T. ) ;
#8121=CARTESIAN_POINT ( 'NONE',  ( -60.99999999999998579, 9.729166666666667851, 2.077350269189628840 ) ) ;
#8123=CARTESIAN_POINT ( 'NONE',  ( -60.99999999999998579, 12.02083333333333215, 0.9226497308103762673 ) ) ;
#8124=CARTESIAN_POINT ( 'NONE',  ( -61.13531646874998415, 10.59895833299193413, 1.000774730468978468 ) ) ;
#8125=CARTESIAN_POINT ( 'NONE',  ( -61.99999999999998579, 8.281249999317203958, 0.3452994616207497591 ) ) ;
#8126=CARTESIAN_POINT ( 'NONE',  ( -61.56765823437498852, 12.34895833299193413, 2.248837904296538515 ) ) ;
#8127=CARTESIAN_POINT ( 'NONE',  ( -61.99999999999998579, 12.65624999931720396, 2.500000000000002665 ) ) ;
#8130=CARTESIAN_POINT ( 'NONE',  ( -62.99999999999998579, 9.104166666666666075, 0.9226497308103756012 ) ) ;
#8134=CARTESIAN_POINT ( 'NONE',  ( -60.99999999999998579, 15.77083333333332860, 0.9226497308103762673 ) ) ;
#8135=CARTESIAN_POINT ( 'NONE',  ( -61.56765823437498142, 13.61979166632526805, 0.7511620957034663704 ) ) ;
#8137=CARTESIAN_POINT ( 'NONE',  ( -61.13531646874998415, 10.82812499965860020, 1.500000000000002220 ) ) ;
#8138=CARTESIAN_POINT ( 'NONE',  ( -61.99999999999997868, 11.65624999931720218, 2.500000000000002665 ) ) ;
#8139=EDGE_LOOP ( 'NONE', ( #3920, #2523, #10765, #9369 ) ) ;
#8140=LINE ( 'NONE', #9962, #6172 ) ;
#8141=CARTESIAN_POINT ( 'NONE',  ( -61.56765823437498142, 11.18229166632526805, 0.7511620957034663704 ) ) ;
#8142=AXIS2_PLACEMENT_3D ( 'NONE', #9305, #965, #6921 ) ;
#8144=CYLINDRICAL_SURFACE ( 'NONE', #6719, 0.9999999999999981126 ) ;
#8145=CARTESIAN_POINT ( 'NONE',  ( -62.49999999999998579, 15.30208333265053611, 0.6339745962155627357 ) ) ;
#8147=ORIENTED_EDGE ( 'NONE', *, *, #2709, .F. ) ;
#8151=CARTESIAN_POINT ( 'NONE',  ( -61.99999999999999289, 13.51562499965860198, 2.498450539062049724 ) ) ;
#8152=CARTESIAN_POINT ( 'NONE',  ( -61.13531646874998415, 9.348958332991935904, 1.000774730468978468 ) ) ;
#8153=VECTOR ( 'NONE', #10044, 1000.000000000000000 ) ;
#8155=ORIENTED_EDGE ( 'NONE', *, *, #5061, .F. ) ;
#8156=CARTESIAN_POINT ( 'NONE',  ( -62.49999999999998579, 12.83333333333333393, 0.6339745962155627357 ) ) ;
#8157=CARTESIAN_POINT ( 'NONE',  ( -62.26794919243111082, 11.04241454900183150, 0.5000000000000013323 ) ) ;
#8159=AXIS2_PLACEMENT_3D ( 'NONE', #4843, #7467, #8196 ) ;
#8160=CARTESIAN_POINT ( 'NONE',  ( -60.99999999999998579, 10.94791666598386826, 2.077350269189628840 ) ) ;
#8162=CARTESIAN_POINT ( 'NONE',  ( -62.43234176562499016, 12.74479166632526805, 2.248837904296538071 ) ) ;
#8166=CARTESIAN_POINT ( 'NONE',  ( -62.86468353124998032, 11.74479166632526628, 1.000774730468978246 ) ) ;
#8167=CARTESIAN_POINT ( 'NONE',  ( -62.99999999999998579, 12.57291666598387003, 0.9226497308103756012 ) ) ;
#8169=CARTESIAN_POINT ( 'NONE',  ( -61.99999999999998579, 15.70312499965860198, 0.5015494609379544944 ) ) ;
#8172=STYLED_ITEM ( 'NONE', ( #7375 ), #6440 ) ;
#8173=EDGE_LOOP ( 'NONE', ( #3749, #18, #7115, #122 ) ) ;
#8175=CARTESIAN_POINT ( 'NONE',  ( -61.99999999999998579, 10.06249999999999822, 0.3452994616207497591 ) ) ;
#8180=EDGE_CURVE ( 'NONE', #5034, #3952, #9773, .T. ) ;
#8182=CARTESIAN_POINT ( 'NONE',  ( -62.86468353124999453, 11.26562499965860020, 1.500000000000002220 ) ) ;
#8183=CARTESIAN_POINT ( 'NONE',  ( -62.99999999999998579, 9.093749999317203958, 1.500000000000001998 ) ) ;
#8185=DIRECTION ( 'NONE',  ( -0.000000000000000000, -1.000000000000000000, -0.000000000000000000 ) ) ;
#8189=CARTESIAN_POINT ( 'NONE',  ( -60.99999999999998579, 14.19791666598386826, 2.077350269189628840 ) ) ;
#8190=CARTESIAN_POINT ( 'NONE',  ( -61.56765823437498852, 13.28645833299193413, 2.248837904296538515 ) ) ;
#8191=CARTESIAN_POINT ( 'NONE',  ( -62.86468353124998032, 9.682291666325266277, 1.000774730468978024 ) ) ;
#8192=CARTESIAN_POINT ( 'NONE',  ( -62.99999999999998579, 8.125000000000000000, 1.500000000000001998 ) ) ;
#8194=CARTESIAN_POINT ( 'NONE',  ( -62.26794919243110371, 8.292414549001831503, 0.4999999999999997780 ) ) ;
#8195=CARTESIAN_POINT ( 'NONE',  ( -61.13531646874997705, 11.36979166632526628, 1.999225269531026417 ) ) ;
#8196=DIRECTION ( 'NONE',  ( 0.000000000000000000, 0.000000000000000000, -1.000000000000000000 ) ) ;
#8197=CARTESIAN_POINT ( 'NONE',  ( -62.99999999999998579, 15.32291666598387003, 0.9226497308103756012 ) ) ;
#8199=ORIENTED_EDGE ( 'NONE', *, *, #4849, .T. ) ;
#8201=DIRECTION ( 'NONE',  ( 0.000000000000000000, 1.000000000000000000, 0.000000000000000000 ) ) ;
#8202=CARTESIAN_POINT ( 'NONE',  ( -61.99999999999999289, 14.26562499965860020, 2.498450539062049724 ) ) ;
#8203=CARTESIAN_POINT ( 'NONE',  ( -61.13531646874998415, 10.34895833299193413, 1.000774730468978468 ) ) ;
#8204=CARTESIAN_POINT ( 'NONE',  ( -61.99999999999998579, 13.56249999999999822, 0.5000000000000013323 ) ) ;
#8206=CARTESIAN_POINT ( 'NONE',  ( -62.49999999999998579, 13.41666666666666785, 2.366025403784441483 ) ) ;
#8207=CARTESIAN_POINT ( 'NONE',  ( -62.49999999999998579, 13.38541666598387003, 2.366025403784441483 ) ) ;
#8210=CARTESIAN_POINT ( 'NONE',  ( -62.99999999999998579, 11.59374999931720218, 1.500000000000001998 ) ) ;
#8211=AXIS2_PLACEMENT_3D ( 'NONE', #2733, #6116, #5054 ) ;
#8213=DIRECTION ( 'NONE',  ( -0.000000000000000000, -1.000000000000000000, -0.000000000000000000 ) ) ;
#8214=CARTESIAN_POINT ( 'NONE',  ( -61.56765823437498852, 14.28645833299193413, 2.248837904296538515 ) ) ;
#8216=( BOUNDED_CURVE ( )  B_SPLINE_CURVE ( 2, ( #8065, #1102, #3833, #5372, #2948, #8780, #2112, #7944, #4430 ),
 .UNSPECIFIED., .F., .T. ) 
 B_SPLINE_CURVE_WITH_KNOTS ( ( 3, 2, 2, 2, 3 ),
 ( 0.3046875000000000000, 0.3072916666666666852, 0.3125000000000000000, 0.3177083333333333148, 0.3203125000000000000 ),
 .UNSPECIFIED. ) 
 CURVE ( )  GEOMETRIC_REPRESENTATION_ITEM ( )  RATIONAL_B_SPLINE_CURVE ( ( 0.9330127018922194093, 0.9330127018922194093, 1.000000000000000000, 0.8660254037844387076, 1.000000000000000000, 0.8660254037844387076, 1.000000000000000000, 0.9330127018922194093, 0.9330127018922194093 ) ) 
 REPRESENTATION_ITEM ( '' )  );
#8220=CARTESIAN_POINT ( 'NONE',  ( -61.99999999999998579, 12.07812499965860020, 2.498450539062049724 ) ) ;
#8224=ORIENTED_EDGE ( 'NONE', *, *, #9254, .F. ) ;
#8228=EDGE_CURVE ( 'NONE', #8833, #9827, #1396, .T. ) ;
#8230=CARTESIAN_POINT ( 'NONE',  ( -61.73205080756886787, 8.770085449632572860, 0.5000000000000006661 ) ) ;
#8231=CARTESIAN_POINT ( 'NONE',  ( -62.99999999999998579, 9.875000000000000000, 1.500000000000001998 ) ) ;
#8233=CYLINDRICAL_SURFACE ( 'NONE', #8314, 0.9999999999999981126 ) ;
#8234=CARTESIAN_POINT ( 'NONE',  ( -61.49999999999998579, 15.51041666598387003, 0.6339745962155628467 ) ) ;
#8235=CARTESIAN_POINT ( 'NONE',  ( -61.99999999999998579, 12.07812499965860020, 2.498450539062049724 ) ) ;
#8236=CARTESIAN_POINT ( 'NONE',  ( -62.26794919243112503, 10.67633545031536890, 2.500000000000000000 ) ) ;
#8239=CARTESIAN_POINT ( 'NONE',  ( -61.99999999999998579, 16.00000000000000000, 1.500000000000002220 ) ) ;
#8242=ORIENTED_EDGE ( 'NONE', *, *, #1384, .T. ) ;
#8244=CARTESIAN_POINT ( 'NONE',  ( -61.13531646874998415, 13.59895833299193413, 1.000774730468978468 ) ) ;
#8245=CARTESIAN_POINT ( 'NONE',  ( -62.43234176562499016, 9.744791666325268054, 2.248837904296538071 ) ) ;
#8247=CARTESIAN_POINT ( 'NONE',  ( -62.26794919243110371, 8.395085449632571084, 2.500000000000000888 ) ) ;
#8248=CARTESIAN_POINT ( 'NONE',  ( -62.43234176562498305, 11.97395833299193413, 0.7511620957034662593 ) ) ;
#8249=CARTESIAN_POINT ( 'NONE',  ( -61.99999999999998579, 8.140624999658601979, 0.5015494609379544944 ) ) ;
#8251=CARTESIAN_POINT ( 'NONE',  ( -62.99999999999998579, 13.59374999931720218, 1.500000000000001998 ) ) ;
#8253=CARTESIAN_POINT ( 'NONE',  ( -61.99999999999998579, 8.453124999658601979, 0.5015494609379544944 ) ) ;
#8255=VERTEX_POINT ( 'NONE', #7158 ) ;
#8258=CARTESIAN_POINT ( 'NONE',  ( -62.86468353124999453, 13.72395833299193590, 1.999225269531025750 ) ) ;
#8259=CARTESIAN_POINT ( 'NONE',  ( -61.99999999999998579, 9.765624999658600203, 2.498450539062049724 ) ) ;
#8261=VERTEX_POINT ( 'NONE', #8823 ) ;
#8262=CARTESIAN_POINT ( 'NONE',  ( -62.99999999999998579, 14.37499999999999822, 1.500000000000001998 ) ) ;
#8263=CARTESIAN_POINT ( 'NONE',  ( -62.49999999999998579, 11.05208333265053611, 0.6339745962155627357 ) ) ;
#8264=( LENGTH_UNIT ( ) NAMED_UNIT ( * ) SI_UNIT ( .MILLI., .METRE. ) );
#8265=CARTESIAN_POINT ( 'NONE',  ( -61.49999999999998579, 12.01041666598387003, 0.6339745962155628467 ) ) ;
#8266=CARTESIAN_POINT ( 'NONE',  ( -62.86468353124998742, 14.47395833299193413, 1.999225269531025972 ) ) ;
#8267=ORIENTED_EDGE ( 'NONE', *, *, #5763, .T. ) ;
#8269=CARTESIAN_POINT ( 'NONE',  ( -62.43234176562499016, 11.55729166632526805, 2.248837904296538071 ) ) ;
#8271=CARTESIAN_POINT ( 'NONE',  ( -61.13531646874998415, 16.14062499965860198, 1.500000000000002220 ) ) ;
#8274=( BOUNDED_CURVE ( )  B_SPLINE_CURVE ( 2, ( #9905, #5731, #10839, #9125, #4112, #2295, #3223, #5680, #1512 ),
 .UNSPECIFIED., .F., .T. ) 
 B_SPLINE_CURVE_WITH_KNOTS ( ( 3, 2, 2, 2, 3 ),
 ( 0.8046875000000000000, 0.8072916666666666297, 0.8125000000000000000, 0.8177083333333333703, 0.8203125000000000000 ),
 .UNSPECIFIED. ) 
 CURVE ( )  GEOMETRIC_REPRESENTATION_ITEM ( )  RATIONAL_B_SPLINE_CURVE ( ( 0.9330127018922194093, 0.9330127018922194093, 1.000000000000000000, 0.8660254037844387076, 1.000000000000000000, 0.8660254037844387076, 1.000000000000000000, 0.9330127018922194093, 0.9330127018922194093 ) ) 
 REPRESENTATION_ITEM ( '' )  );
#8277=CARTESIAN_POINT ( 'NONE',  ( -61.49999999999998579, 9.958333333333332149, 2.366025403784441927 ) ) ;
#8279=CARTESIAN_POINT ( 'NONE',  ( -60.99999999999998579, 12.27083333333333570, 0.9226497308103762673 ) ) ;
#8282=CARTESIAN_POINT ( 'NONE',  ( -62.86468353124998742, 11.28645833299193590, 1.999225269531025972 ) ) ;
#8283=CARTESIAN_POINT ( 'NONE',  ( -61.99999999999998579, 14.53124999931720041, 0.5000000000000013323 ) ) ;
#8286=ORIENTED_EDGE ( 'NONE', *, *, #7358, .F. ) ;
#8287=DIRECTION ( 'NONE',  ( 0.000000000000000000, 0.000000000000000000, -1.000000000000000000 ) ) ;
#8288=CARTESIAN_POINT ( 'NONE',  ( -61.99999999999998579, 13.39062499965860020, 0.5015494609379544944 ) ) ;
#8290=DIRECTION ( 'NONE',  ( -0.000000000000000000, -1.000000000000000000, -0.000000000000000000 ) ) ;
#8291=CARTESIAN_POINT ( 'NONE',  ( -61.13531646874997705, 13.16145833299193413, 1.000774730468978468 ) ) ;
#8292=CARTESIAN_POINT ( 'NONE',  ( -61.13531646874998415, 15.16145833299193590, 1.000774730468978468 ) ) ;
#8293=CARTESIAN_POINT ( 'NONE',  ( -61.99999999999998579, 13.90624999931720218, 2.500000000000002665 ) ) ;
#8294=CARTESIAN_POINT ( 'NONE',  ( -62.26794919243111082, 13.54241454900183150, 0.5000000000000013323 ) ) ;
#8295=CARTESIAN_POINT ( 'NONE',  ( -61.49999999999998579, 16.01041666598386826, 0.6339745962155628467 ) ) ;
#8299=CARTESIAN_POINT ( 'NONE',  ( -61.99999999999999289, 14.14062499965860198, 0.5015494609379544944 ) ) ;
#8300=CARTESIAN_POINT ( 'NONE',  ( -61.99999999999998579, 9.640624999658600203, 0.5015494609379544944 ) ) ;
#8302=CARTESIAN_POINT ( 'NONE',  ( -61.13531646874998415, 16.14062499965860198, 1.500000000000002220 ) ) ;
#8304=ORIENTED_EDGE ( 'NONE', *, *, #10418, .T. ) ;
#8305=CARTESIAN_POINT ( 'NONE',  ( -61.49999999999998579, 13.70833333333333215, 2.366025403784441927 ) ) ;
#8308=CARTESIAN_POINT ( 'NONE',  ( -62.99999999999998579, 11.57291666598387003, 0.9226497308103756012 ) ) ;
#8310=VECTOR ( 'NONE', #5599, 1000.000000000000000 ) ;
#8311=CARTESIAN_POINT ( 'NONE',  ( -62.86468353124998032, 13.68229166632526983, 1.000774730468978246 ) ) ;
#8312=EDGE_CURVE ( 'NONE', #3615, #10295, #4429, .T. ) ;
#8314=AXIS2_PLACEMENT_3D ( 'NONE', #6509, #9162, #9996 ) ;
#8315=CARTESIAN_POINT ( 'NONE',  ( -61.13531646874998415, 11.91145833299193413, 1.000774730468978468 ) ) ;
#8316=DIRECTION ( 'NONE',  ( 0.000000000000000000, 0.000000000000000000, -1.000000000000000000 ) ) ;
#8317=VECTOR ( 'NONE', #2534, 1000.000000000000000 ) ;
#8319=ORIENTED_EDGE ( 'NONE', *, *, #8995, .T. ) ;
#8324=CARTESIAN_POINT ( 'NONE',  ( -61.49999999999998579, 9.510416665983870033, 0.6339745962155628467 ) ) ;
#8325=CARTESIAN_POINT ( 'NONE',  ( -62.49999999999998579, 11.08333333333333393, 0.6339745962155627357 ) ) ;
#8327=CARTESIAN_POINT ( 'NONE',  ( -60.99999999999998579, 14.96874999931720218, 1.500000000000002220 ) ) ;
#8328=CARTESIAN_POINT ( 'NONE',  ( -60.99999999999998579, 8.229166666666667851, 2.077350269189628840 ) ) ;
#8330=CARTESIAN_POINT ( 'NONE',  ( -61.49999999999998579, 9.177083332650536107, 2.366025403784441927 ) ) ;
#8332=CARTESIAN_POINT ( 'NONE',  ( -61.13531646874998415, 11.91145833299193413, 1.000774730468978468 ) ) ;
#8334=CARTESIAN_POINT ( 'NONE',  ( -62.99999999999998579, 14.59374999931720218, 1.500000000000001998 ) ) ;
#8336=( BOUNDED_CURVE ( )  B_SPLINE_CURVE ( 2, ( #8875, #194, #1263, #434, #3818, #3579, #10297 ),
 .UNSPECIFIED., .F., .T. ) 
 B_SPLINE_CURVE_WITH_KNOTS ( ( 3, 2, 2, 3 ),
 ( 0.9609375000000000000, 0.9635416666666666297, 0.9687500000000000000, 0.9725886266600324292 ),
 .UNSPECIFIED. ) 
 CURVE ( )  GEOMETRIC_REPRESENTATION_ITEM ( )  RATIONAL_B_SPLINE_CURVE ( ( 0.9330127018922194093, 0.9330127018922194093, 1.000000000000000000, 0.8660254037844387076, 1.000000000000000000, 0.9012585362943751344, 0.9480652127606670199 ) ) 
 REPRESENTATION_ITEM ( '' )  );
#8337=CARTESIAN_POINT ( 'NONE',  ( -62.49999999999998579, 15.41666666666666607, 2.366025403784441483 ) ) ;
#8340=ORIENTED_EDGE ( 'NONE', *, *, #10973, .F. ) ;
#8341=CARTESIAN_POINT ( 'NONE',  ( -61.99999999999998579, 13.65624999931720218, 2.500000000000002665 ) ) ;
#8342=EDGE_CURVE ( 'NONE', #8888, #2070, #2524, .T. ) ;
#8343=CARTESIAN_POINT ( 'NONE',  ( -62.43234176562499016, 13.99479166632526805, 2.248837904296538071 ) ) ;
#8345=CARTESIAN_POINT ( 'NONE',  ( -61.13531646874998415, 13.66145833299193590, 1.000774730468978468 ) ) ;
#8349=CARTESIAN_POINT ( 'NONE',  ( -61.13531646874997705, 12.61979166632526805, 1.999225269531026417 ) ) ;
#8350=CARTESIAN_POINT ( 'NONE',  ( -61.56765823437498142, 15.68229166632526628, 0.7511620957034663704 ) ) ;
#8352=FACE_OUTER_BOUND ( 'NONE', #612, .T. ) ;
#8353=CARTESIAN_POINT ( 'NONE',  ( -62.99999999999998579, 16.09374999931720396, 1.500000000000001998 ) ) ;
#8354=CARTESIAN_POINT ( 'NONE',  ( -62.26794919243111082, 10.42633545031537246, 2.500000000000003109 ) ) ;
#8355=ORIENTED_EDGE ( 'NONE', *, *, #5371, .T. ) ;
#8357=CARTESIAN_POINT ( 'NONE',  ( -61.99999999999998579, 12.56249999999999822, 0.5000000000000013323 ) ) ;
#8358=CARTESIAN_POINT ( 'NONE',  ( -62.86468353124998032, 14.43229166632526983, 1.000774730468978024 ) ) ;
#8360=CARTESIAN_POINT ( 'NONE',  ( -61.13531646874998415, 9.598958332991934128, 1.000774730468978468 ) ) ;
#8361=CARTESIAN_POINT ( 'NONE',  ( -61.13531646874997705, 15.66145833299193590, 1.000774730468978468 ) ) ;
#8363=ORIENTED_EDGE ( 'NONE', *, *, #9314, .F. ) ;
#8364=CARTESIAN_POINT ( 'NONE',  ( -60.99999999999998579, 13.52083333333333215, 0.9226497308103762673 ) ) ;
#8365=CARTESIAN_POINT ( 'NONE',  ( -61.13531646874998415, 9.390624999658600203, 1.500000000000002220 ) ) ;
#8367=CARTESIAN_POINT ( 'NONE',  ( -61.49999999999998579, 12.17708333265053611, 2.366025403784441927 ) ) ;
#8369=CARTESIAN_POINT ( 'NONE',  ( -62.86468353124998742, 13.72395833299193413, 1.999225269531025972 ) ) ;
#8371=ADVANCED_FACE ( 'NONE', ( #9768 ), #10592, .T. ) ;
#8372=VERTEX_POINT ( 'NONE', #10757 ) ;
#8373=CARTESIAN_POINT ( 'NONE',  ( -61.99999999999998579, 13.07812499965860198, 2.498450539062049724 ) ) ;
#8375=EDGE_CURVE ( 'NONE', #3158, #7302, #6876, .T. ) ;
#8376=CARTESIAN_POINT ( 'NONE',  ( -61.99999999999998579, 13.78124999931720218, 0.5000000000000013323 ) ) ;
#8377=EDGE_LOOP ( 'NONE', ( #10416, #5914, #10916, #3424 ) ) ;
#8382=CARTESIAN_POINT ( 'NONE',  ( -62.49999999999998579, 11.58333333333333393, 0.6339745962155627357 ) ) ;
#8383=EDGE_LOOP ( 'NONE', ( #4688, #4219, #5773, #10176 ) ) ;
#8385=CARTESIAN_POINT ( 'NONE',  ( -62.49999999999998579, 13.88541666598387003, 2.366025403784441483 ) ) ;
#8388=CARTESIAN_POINT ( 'NONE',  ( -62.86468353124998742, 13.28645833299193413, 1.999225269531025972 ) ) ;
#8393=CARTESIAN_POINT ( 'NONE',  ( -61.73205080756886076, 13.27008544963257286, 0.5000000000000014433 ) ) ;
#8395=CARTESIAN_POINT ( 'NONE',  ( -61.56765823437498852, 15.78645833299193590, 2.248837904296538515 ) ) ;
#8396=CARTESIAN_POINT ( 'NONE',  ( -62.99999999999998579, 11.87500000000000000, 1.500000000000001998 ) ) ;
#8399=CARTESIAN_POINT ( 'NONE',  ( -61.13531646874998415, 12.39062499965860198, 1.500000000000002220 ) ) ;
#8400=CARTESIAN_POINT ( 'NONE',  ( -62.86468353124998742, 16.03645833299193768, 1.999225269531025972 ) ) ;
#8402=CARTESIAN_POINT ( 'NONE',  ( -61.99999999999998579, 12.56249999999999822, 0.5000000000000013323 ) ) ;
#8403=( BOUNDED_CURVE ( )  B_SPLINE_CURVE ( 2, ( #1199, #2756, #7928, #7815, #5293, #1143, #8705, #8816, #2933 ),
 .UNSPECIFIED., .F., .T. ) 
 B_SPLINE_CURVE_WITH_KNOTS ( ( 3, 2, 2, 2, 3 ),
 ( 0.2578125000000000000, 0.2604166666666666852, 0.2656250000000000000, 0.2708333333333333148, 0.2734375000000000000 ),
 .UNSPECIFIED. ) 
 CURVE ( )  GEOMETRIC_REPRESENTATION_ITEM ( )  RATIONAL_B_SPLINE_CURVE ( ( 0.9330127018922194093, 0.9330127018922194093, 1.000000000000000000, 0.8660254037844387076, 1.000000000000000000, 0.8660254037844387076, 1.000000000000000000, 0.9330127018922194093, 0.9330127018922194093 ) ) 
 REPRESENTATION_ITEM ( '' )  );
#8405=CARTESIAN_POINT ( 'NONE',  ( -61.56765823437498852, 8.598958332991934128, 2.248837904296538515 ) ) ;
#8409=LINE ( 'NONE', #10539, #4231 ) ;
#8411=CARTESIAN_POINT ( 'NONE',  ( -62.86468353124999453, 14.70312499965860020, 1.500000000000002220 ) ) ;
#8412=CARTESIAN_POINT ( 'NONE',  ( -62.43234176562499016, 11.74479166632526805, 2.248837904296538071 ) ) ;
#8413=CARTESIAN_POINT ( 'NONE',  ( -61.99999999999999289, 15.07812499965860376, 2.498450539062049724 ) ) ;
#8415=EDGE_LOOP ( 'NONE', ( #5029, #9792, #3207, #10512 ) ) ;
#8416=CARTESIAN_POINT ( 'NONE',  ( -60.99999999999998579, 14.00000000000000000, 1.500000000000002220 ) ) ;
#8417=CARTESIAN_POINT ( 'NONE',  ( -61.56765823437498142, 8.932291666325268054, 0.7511620957034663704 ) ) ;
#8418=CARTESIAN_POINT ( 'NONE',  ( -61.99999999999998579, 11.90624999931720396, 2.654700538379254571 ) ) ;
#8419=ORIENTED_EDGE ( 'NONE', *, *, #9500, .F. ) ;
#8421=CARTESIAN_POINT ( 'NONE',  ( -61.73205080756886076, 9.448664549684629321, 2.500000000000003109 ) ) ;
#8422=CARTESIAN_POINT ( 'NONE',  ( -62.43234176562499016, 13.99479166632526805, 2.248837904296538071 ) ) ;
#8426=CARTESIAN_POINT ( 'NONE',  ( -62.86468353124998742, 13.53645833299193413, 1.999225269531025972 ) ) ;
#8427=FACE_OUTER_BOUND ( 'NONE', #8173, .T. ) ;
#8429=ORIENTED_EDGE ( 'NONE', *, *, #811, .F. ) ;
#8431=ORIENTED_EDGE ( 'NONE', *, *, #1448, .T. ) ;
#8432=CARTESIAN_POINT ( 'NONE',  ( -61.49999999999998579, 10.79166666666666607, 0.6339745962155628467 ) ) ;
#8433=ORIENTED_EDGE ( 'NONE', *, *, #2745, .T. ) ;
#8434=CARTESIAN_POINT ( 'NONE',  ( -62.86468353124998742, 9.536458332991935904, 1.999225269531025972 ) ) ;
#8436=CARTESIAN_POINT ( 'NONE',  ( -61.99999999999998579, 13.07812499965860198, 2.498450539062049724 ) ) ;
#8444=CARTESIAN_POINT ( 'NONE',  ( -62.86468353124998742, 15.22395833299193590, 1.999225269531025972 ) ) ;
#8447=DIRECTION ( 'NONE',  ( -0.000000000000000000, -1.000000000000000000, -0.000000000000000000 ) ) ;
#8448=CARTESIAN_POINT ( 'NONE',  ( -62.86468353124999453, 13.01562499965860198, 1.500000000000002220 ) ) ;
#8449=CARTESIAN_POINT ( 'NONE',  ( -61.99999999999998579, 15.82812499965860020, 2.498450539062049724 ) ) ;
#8450=CARTESIAN_POINT ( 'NONE',  ( -61.99999999999998579, 14.78124999931720218, 0.5000000000000013323 ) ) ;
#8451=CARTESIAN_POINT ( 'NONE',  ( -61.49999999999998579, 13.51041666598387003, 0.6339745962155628467 ) ) ;
#8452=CARTESIAN_POINT ( 'NONE',  ( -62.43234176562499016, 9.057291666325268054, 2.248837904296538071 ) ) ;
#8453=CARTESIAN_POINT ( 'NONE',  ( -61.99999999999998579, 26.00000000000000355, 1.500000000000002220 ) ) ;
#8456=CARTESIAN_POINT ( 'NONE',  ( -62.99999999999998579, 12.60416666666666607, 0.9226497308103756012 ) ) ;
#8457=EDGE_CURVE ( 'NONE', #3127, #2471, #9396, .T. ) ;
#8458=CARTESIAN_POINT ( 'NONE',  ( -62.43234176562498305, 14.91145833299193590, 0.7511620957034662593 ) ) ;
#8459=CARTESIAN_POINT ( 'NONE',  ( -61.56765823437498852, 10.53645833299193413, 2.248837904296538515 ) ) ;
#8460=CARTESIAN_POINT ( 'NONE',  ( -61.56765823437498852, 15.59895833299193590, 2.248837904296538515 ) ) ;
#8463=CARTESIAN_POINT ( 'NONE',  ( -62.99999999999998579, 14.64583333333333393, 2.077350269189627952 ) ) ;
#8464=CARTESIAN_POINT ( 'NONE',  ( -62.86468353124999453, 8.765624999658601979, 1.500000000000002220 ) ) ;
#8467=CARTESIAN_POINT ( 'NONE',  ( -62.99999999999998579, 12.82291666598386826, 0.9226497308103756012 ) ) ;
#8469=CARTESIAN_POINT ( 'NONE',  ( -61.99999999999998579, 16.00000000000000000, 1.500000000000002220 ) ) ;
#8471=CARTESIAN_POINT ( 'NONE',  ( -62.43234176562498305, 12.16145833299193413, 0.7511620957034662593 ) ) ;
#8475=CARTESIAN_POINT ( 'NONE',  ( -62.43234176562499016, 12.80729166632526805, 2.248837904296538071 ) ) ;
#8476=CARTESIAN_POINT ( 'NONE',  ( -61.73205080756886076, 11.41741454900183328, 2.500000000000003109 ) ) ;
#8477=STYLED_ITEM('',(#11027),#8688);
#8486=CIRCLE ( 'NONE', #3162, 2.500000000000002220 ) ;
#8487=CARTESIAN_POINT ( 'NONE',  ( -62.86468353124998032, 9.244791666325268054, 1.000774730468978246 ) ) ;
#8488=CARTESIAN_POINT ( 'NONE',  ( -61.49999999999998579, 14.20833333333333393, 2.366025403784441927 ) ) ;
#8490=CARTESIAN_POINT ( 'NONE',  ( -62.86468353124999453, 13.26562499965860198, 1.500000000000002220 ) ) ;
#8495=VERTEX_POINT ( 'NONE', #8990 ) ;
#8496=CARTESIAN_POINT ( 'NONE',  ( -61.73205080756886076, 12.69866454968462754, 2.500000000000003109 ) ) ;
#8497=CARTESIAN_POINT ( 'NONE',  ( -62.43234176562498305, 14.66145833299193413, 0.7511620957034662593 ) ) ;
#8500=CARTESIAN_POINT ( 'NONE',  ( -61.99999999999998579, 16.00000000000000000, 2.500000000000000444 ) ) ;
#8502=CARTESIAN_POINT ( 'NONE',  ( -60.99999999999998579, 10.75000000000000000, 1.500000000000002220 ) ) ;
#8503=CARTESIAN_POINT ( 'NONE',  ( -62.86468353124999453, 13.03645833299193413, 1.999225269531025750 ) ) ;
#8504=CARTESIAN_POINT ( 'NONE',  ( -62.43234176562498305, 8.911458332991934128, 0.7511620957034662593 ) ) ;
#8505=DIRECTION ( 'NONE',  ( -0.000000000000000000, -1.000000000000000000, -0.000000000000000000 ) ) ;
#8507=CARTESIAN_POINT ( 'NONE',  ( -61.56765823437498142, 9.182291666325268054, 0.7511620957034663704 ) ) ;
#8508=DIRECTION ( 'NONE',  ( 0.000000000000000000, 0.000000000000000000, -1.000000000000000000 ) ) ;
#8514=CARTESIAN_POINT ( 'NONE',  ( -61.99999999999999289, 15.26562499965860020, 2.498450539062049724 ) ) ;
#8515=CARTESIAN_POINT ( 'NONE',  ( -61.99999999999998579, 11.64062499965860198, 0.5015494609379544944 ) ) ;
#8516=CARTESIAN_POINT ( 'NONE',  ( -62.43234176562499016, 15.55729166632526628, 2.248837904296538071 ) ) ;
#8518=VERTEX_POINT ( 'NONE', #7271 ) ;
#8519=CARTESIAN_POINT ( 'NONE',  ( -60.99999999999998579, 14.49999999999999822, 1.500000000000002220 ) ) ;
#8520=CARTESIAN_POINT ( 'NONE',  ( -62.43234176562499016, 9.057291666325268054, 2.248837904296538071 ) ) ;
#8523=CARTESIAN_POINT ( 'NONE',  ( -62.49999999999998579, 13.55208333265053433, 0.6339745962155627357 ) ) ;
#8524=CARTESIAN_POINT ( 'NONE',  ( -62.26794919243111082, 14.57366454968463110, 0.5000000000000013323 ) ) ;
#8527=CARTESIAN_POINT ( 'NONE',  ( -61.99999999999999289, 11.51562499965860020, 2.498450539062049724 ) ) ;
#8529=CARTESIAN_POINT ( 'NONE',  ( -61.99999999999998579, 12.93750000000000000, 2.500000000000002665 ) ) ;
#8530=ORIENTED_EDGE ( 'NONE', *, *, #4281, .T. ) ;
#8532=CARTESIAN_POINT ( 'NONE',  ( -61.99999999999998579, 10.31250000000000000, 0.5000000000000013323 ) ) ;
#8533=CARTESIAN_POINT ( 'NONE',  ( -62.43234176562499016, 12.55729166632526805, 2.248837904296538071 ) ) ;
#8534=DIRECTION ( 'NONE',  ( 0.000000000000000000, 0.000000000000000000, -1.000000000000000000 ) ) ;
#8535=CARTESIAN_POINT ( 'NONE',  ( -62.99999999999998579, 9.822916665983871809, 0.9226497308103756012 ) ) ;
#8539=EDGE_LOOP ( 'NONE', ( #6252, #6762, #2976, #6153 ) ) ;
#8540=CARTESIAN_POINT ( 'NONE',  ( -61.99999999999998579, 16.00000000000000000, 1.500000000000002220 ) ) ;
#8541=CARTESIAN_POINT ( 'NONE',  ( -62.86468353124999453, 11.70312499965860198, 1.500000000000002220 ) ) ;
#8543=CLOSED_SHELL ( 'NONE', ( #3333, #9518, #5594, #10780, #1308, #263, #2416, #8810, #5559, #868, #10818, #8766, #8709, #9541, #10507, #9146, #1973, #2262, #9379, #8614, #7945, #7556, #113, #1137, #10191, #1483, #1653, #10030, #6127, #7833, #10422, #5548, #5862, #316, #10129, #8371, #3829, #10527, #5634, #10125, #10717, #9725, #10759, #1272, #2622, #8666, #8013, #287, #10714, #5444, #3600, #1073, #2592, #10153, #180, #3724, #1830, #2567, #6148, #9547, #6644, #5775, #10081, #6374, #8046, #3213, #1708, #4137, #4796, #4615, #297, #3953, #538, #10229, #8796, #5584, #6202, #8951 ) ) ;
#8544=CARTESIAN_POINT ( 'NONE',  ( -61.56765823437498142, 9.432291666325268054, 0.7511620957034663704 ) ) ;
#8545=CARTESIAN_POINT ( 'NONE',  ( -61.13531646874998415, 13.41145833299193235, 1.000774730468978468 ) ) ;
#8550=EDGE_CURVE ( 'NONE', #8575, #2384, #606, .T. ) ;
#8552=CARTESIAN_POINT ( 'NONE',  ( -62.26794919243111082, 10.82366454968462932, 0.5000000000000013323 ) ) ;
#8553=CARTESIAN_POINT ( 'NONE',  ( -61.13531646874998415, 15.32812499965860020, 1.500000000000002220 ) ) ;
#8556=( BOUNDED_CURVE ( )  B_SPLINE_CURVE ( 2, ( #8068, #3603, #10379, #6337, #8661, #4432, #7832, #2775, #6162 ),
 .UNSPECIFIED., .F., .T. ) 
 B_SPLINE_CURVE_WITH_KNOTS ( ( 3, 2, 2, 2, 3 ),
 ( 0.5546875000000000000, 0.5572916666666666297, 0.5625000000000000000, 0.5677083333333333703, 0.5703125000000000000 ),
 .UNSPECIFIED. ) 
 CURVE ( )  GEOMETRIC_REPRESENTATION_ITEM ( )  RATIONAL_B_SPLINE_CURVE ( ( 0.9330127018922194093, 0.9330127018922194093, 1.000000000000000000, 0.8660254037844387076, 1.000000000000000000, 0.8660254037844387076, 1.000000000000000000, 0.9330127018922194093, 0.9330127018922194093 ) ) 
 REPRESENTATION_ITEM ( '' )  );
#8557=CARTESIAN_POINT ( 'NONE',  ( -61.99999999999998579, 16.00000000000000000, 0.5000000000000041078 ) ) ;
#8559=CARTESIAN_POINT ( 'NONE',  ( -61.56765823437498852, 13.59895833299193413, 2.248837904296538515 ) ) ;
#8560=AXIS2_PLACEMENT_3D ( 'NONE', #4405, #1920, #8763 ) ;
#8561=CARTESIAN_POINT ( 'NONE',  ( -62.43234176562499016, 8.244791666325268054, 2.248837904296538071 ) ) ;
#8562=FACE_OUTER_BOUND ( 'NONE', #9801, .T. ) ;
#8563=DIRECTION ( 'NONE',  ( -0.000000000000000000, -1.000000000000000000, -0.000000000000000000 ) ) ;
#8564=CARTESIAN_POINT ( 'NONE',  ( -61.13531646874998415, 9.119791666325268054, 1.999225269531026417 ) ) ;
#8570=AXIS2_PLACEMENT_3D ( 'NONE', #7364, #8201, #9029 ) ;
#8571=CARTESIAN_POINT ( 'NONE',  ( -62.43234176562499016, 15.74479166632526628, 2.248837904296538071 ) ) ;
#8572=CARTESIAN_POINT ( 'NONE',  ( -61.13531646874998415, 10.84895833299193590, 1.000774730468978468 ) ) ;
#8573=CARTESIAN_POINT ( 'NONE',  ( -61.56765823437498852, 9.286458332991935904, 2.248837904296538515 ) ) ;
#8574=CARTESIAN_POINT ( 'NONE',  ( -62.49999999999998579, 13.13541666598387003, 2.366025403784441483 ) ) ;
#8575=VERTEX_POINT ( 'NONE', #5024 ) ;
#8576=CARTESIAN_POINT ( 'NONE',  ( -62.99999999999998579, 15.10416666666666785, 0.9226497308103756012 ) ) ;
#8577=EDGE_CURVE ( 'NONE', #9081, #10876, #7433, .T. ) ;
#8578=CARTESIAN_POINT ( 'NONE',  ( -61.56765823437498142, 8.432291666325268054, 0.7511620957034663704 ) ) ;
#8581=CARTESIAN_POINT ( 'NONE',  ( -61.99999999999998579, 12.78124999931720218, 0.3452994616207497591 ) ) ;
#8582=CARTESIAN_POINT ( 'NONE',  ( -62.99999999999998579, 14.60416666666666430, 0.9226497308103756012 ) ) ;
#8585=CARTESIAN_POINT ( 'NONE',  ( -61.99999999999999289, 11.14062499965860020, 0.5015494609379544944 ) ) ;
#8587=CARTESIAN_POINT ( 'NONE',  ( -61.99999999999998579, 11.03124999931720218, 0.5000000000000013323 ) ) ;
#8588=ORIENTED_EDGE ( 'NONE', *, *, #4109, .F. ) ;
#8590=CARTESIAN_POINT ( 'NONE',  ( -61.13531646874998415, 12.64062499965860198, 1.500000000000002220 ) ) ;
#8591=CARTESIAN_POINT ( 'NONE',  ( -61.99999999999998579, 13.81249999999999822, 0.5000000000000013323 ) ) ;
#8592=CARTESIAN_POINT ( 'NONE',  ( -62.99999999999998579, 9.572916665983870033, 0.9226497308103756012 ) ) ;
#8593=ORIENTED_EDGE ( 'NONE', *, *, #4725, .F. ) ;
#8594=CARTESIAN_POINT ( 'NONE',  ( -61.99999999999998579, 9.687500000000000000, 2.500000000000002665 ) ) ;
#8596=CARTESIAN_POINT ( 'NONE',  ( -60.99999999999998579, 14.75000000000000000, 1.500000000000002220 ) ) ;
#8597=CARTESIAN_POINT ( 'NONE',  ( -61.99999999999998579, 11.14062499965860020, 0.5015494609379544944 ) ) ;
#8599=ORIENTED_EDGE ( 'NONE', *, *, #5434, .T. ) ;
#8600=CARTESIAN_POINT ( 'NONE',  ( -62.86468353124998742, 9.286458332991934128, 1.999225269531025972 ) ) ;
#8601=CARTESIAN_POINT ( 'NONE',  ( -62.99999999999998579, 13.86458333265053611, 2.077350269189627952 ) ) ;
#8602=CARTESIAN_POINT ( 'NONE',  ( -61.56765823437498852, 13.59895833299193413, 2.248837904296538515 ) ) ;
#8603=CARTESIAN_POINT ( 'NONE',  ( -61.99999999999998579, 9.281249999317203958, 0.5000000000000013323 ) ) ;
#8604=ORIENTED_EDGE ( 'NONE', *, *, #4867, .T. ) ;
#8608=CARTESIAN_POINT ( 'NONE',  ( -61.99999999999998579, 16.00000000000000000, 1.500000000000002220 ) ) ;
#8609=CARTESIAN_POINT ( 'NONE',  ( -61.13531646874998415, 15.07812499965860020, 1.500000000000002220 ) ) ;
#8610=CARTESIAN_POINT ( 'NONE',  ( -62.99999999999998579, 8.843749999317203958, 1.500000000000001998 ) ) ;
#8611=CARTESIAN_POINT ( 'NONE',  ( -61.99999999999998579, 12.43749999999999822, 2.500000000000002665 ) ) ;
#8612=CARTESIAN_POINT ( 'NONE',  ( -61.99999999999998579, 16.00000000000000000, 2.500000000000000444 ) ) ;
#8613=CARTESIAN_POINT ( 'NONE',  ( -62.86468353124999453, 13.53645833299193413, 1.999225269531025750 ) ) ;
#8614=ADVANCED_FACE ( 'NONE', ( #10811 ), #7432, .T. ) ;
#8615=CARTESIAN_POINT ( 'NONE',  ( -61.56765823437498142, 8.369791666325268054, 0.7511620957034663704 ) ) ;
#8618=CARTESIAN_POINT ( 'NONE',  ( -61.13531646874998415, 9.640624999658601979, 1.500000000000002220 ) ) ;
#8619=CARTESIAN_POINT ( 'NONE',  ( -61.99999999999998579, 16.00000000000000000, 0.5000000000000041078 ) ) ;
#8622=CARTESIAN_POINT ( 'NONE',  ( -60.99999999999998579, 11.23958333265053611, 0.9226497308103762673 ) ) ;
#8623=( BOUNDED_CURVE ( )  B_SPLINE_CURVE ( 2, ( #884, #1721, #1047, #10323, #6892, #4263, #54, #3438, #2607 ),
 .UNSPECIFIED., .F., .T. ) 
 B_SPLINE_CURVE_WITH_KNOTS ( ( 3, 2, 2, 2, 3 ),
 ( 0.5234375000000000000, 0.5260416666666666297, 0.5312500000000000000, 0.5364583333333333703, 0.5390625000000000000 ),
 .UNSPECIFIED. ) 
 CURVE ( )  GEOMETRIC_REPRESENTATION_ITEM ( )  RATIONAL_B_SPLINE_CURVE ( ( 0.9330127018922194093, 0.9330127018922194093, 1.000000000000000000, 0.8660254037844387076, 1.000000000000000000, 0.8660254037844387076, 1.000000000000000000, 0.9330127018922194093, 0.9330127018922194093 ) ) 
 REPRESENTATION_ITEM ( '' )  );
#8624=CARTESIAN_POINT ( 'NONE',  ( -62.86468353124999453, 15.97395833299193590, 1.999225269531025750 ) ) ;
#8625=CARTESIAN_POINT ( 'NONE',  ( -61.56765823437498142, 10.61979166632526805, 0.7511620957034663704 ) ) ;
#8626=CARTESIAN_POINT ( 'NONE',  ( -61.56765823437498142, 8.869791666325268054, 0.7511620957034663704 ) ) ;
#8628=ORIENTED_EDGE ( 'NONE', *, *, #4352, .T. ) ;
#8629=CARTESIAN_POINT ( 'NONE',  ( -62.49999999999998579, 14.66666666666666607, 2.366025403784441483 ) ) ;
#8630=CARTESIAN_POINT ( 'NONE',  ( -61.99999999999999289, 10.45312499965860198, 0.5015494609379544944 ) ) ;
#8632=CARTESIAN_POINT ( 'NONE',  ( -62.49999999999998579, 12.80208333265053611, 0.6339745962155627357 ) ) ;
#8633=CARTESIAN_POINT ( 'NONE',  ( -62.26794919243111082, 13.07366454968462932, 0.5000000000000013323 ) ) ;
#8634=ORIENTED_EDGE ( 'NONE', *, *, #1204, .T. ) ;
#8635=DIRECTION ( 'NONE',  ( 0.000000000000000000, 0.000000000000000000, -1.000000000000000000 ) ) ;
#8636=CARTESIAN_POINT ( 'NONE',  ( -61.13531646874997705, 12.05729166632526628, 1.999225269531026417 ) ) ;
#8637=CARTESIAN_POINT ( 'NONE',  ( -62.99999999999998579, 15.60416666666666607, 0.9226497308103756012 ) ) ;
#8638=CARTESIAN_POINT ( 'NONE',  ( -61.99999999999998579, 15.43749999999999822, 2.500000000000002665 ) ) ;
#8640=CARTESIAN_POINT ( 'NONE',  ( -62.99999999999998579, 11.12500000000000000, 1.500000000000001998 ) ) ;
#8642=CARTESIAN_POINT ( 'NONE',  ( -62.86468353124999453, 13.76562499965860198, 1.500000000000002220 ) ) ;
#8643=CARTESIAN_POINT ( 'NONE',  ( -60.99999999999998579, 10.25000000000000000, 1.500000000000002220 ) ) ;
#8644=CARTESIAN_POINT ( 'NONE',  ( -60.99999999999998579, 9.718749999317202182, 1.500000000000002220 ) ) ;
#8649=EDGE_CURVE ( 'NONE', #10734, #9779, #9704, .T. ) ;
#8650=CARTESIAN_POINT ( 'NONE',  ( -61.56765823437498852, 10.78645833299193413, 2.248837904296538515 ) ) ;
#8652=CARTESIAN_POINT ( 'NONE',  ( -62.43234176562498305, 9.223958332991935904, 0.7511620957034662593 ) ) ;
#8653=DIRECTION ( 'NONE',  ( -0.000000000000000000, -1.000000000000000000, -0.000000000000000000 ) ) ;
#8654=CARTESIAN_POINT ( 'NONE',  ( -62.43234176562498305, 14.22395833299193413, 0.7511620957034662593 ) ) ;
#8655=CARTESIAN_POINT ( 'NONE',  ( -61.99999999999998579, 13.18750000000000000, 2.500000000000002665 ) ) ;
#8657=CARTESIAN_POINT ( 'NONE',  ( -62.26794919243111082, 9.426335450315370679, 2.500000000000003109 ) ) ;
#8659=CIRCLE ( 'NONE', #7963, 0.9999999999999983347 ) ;
#8661=CARTESIAN_POINT ( 'NONE',  ( -60.99999999999998579, 12.71874999931720396, 1.500000000000002220 ) ) ;
#8662=CARTESIAN_POINT ( 'NONE',  ( -62.99999999999998579, 8.375000000000000000, 1.500000000000001998 ) ) ;
#8666=ADVANCED_FACE ( 'NONE', ( #5918 ), #1750, .T. ) ;
#8667=CARTESIAN_POINT ( 'NONE',  ( -61.13531646874997705, 14.36979166632527161, 1.999225269531026417 ) ) ;
#8669=CARTESIAN_POINT ( 'NONE',  ( -62.43234176562499016, 8.994791666325268054, 2.248837904296538071 ) ) ;
#8670=CARTESIAN_POINT ( 'NONE',  ( -61.99999999999998579, 9.312500000000000000, 0.5000000000000013323 ) ) ;
#8672=CARTESIAN_POINT ( 'NONE',  ( -62.86468353124998742, 10.28645833299193590, 1.999225269531025972 ) ) ;
#8678=CYLINDRICAL_SURFACE ( 'NONE', #758, 0.9999999999999981126 ) ;
#8681=CARTESIAN_POINT ( 'NONE',  ( -62.86468353124998032, 14.93229166632526983, 1.000774730468978024 ) ) ;
#8682=CARTESIAN_POINT ( 'NONE',  ( -61.56765823437498852, 12.28645833299193413, 2.248837904296538515 ) ) ;
#8683=CARTESIAN_POINT ( 'NONE',  ( -61.56765823437498142, 8.369791666325268054, 0.7511620957034663704 ) ) ;
#8686=CARTESIAN_POINT ( 'NONE',  ( -62.99999999999998579, 15.62500000000000000, 1.500000000000001998 ) ) ;
#8687=CARTESIAN_POINT ( 'NONE',  ( -62.43234176562498305, 10.47395833299193413, 0.7511620957034662593 ) ) ;
#8688=MANIFOLD_SOLID_BREP ( 'Thread1', #8543 ) ;
#8690=CARTESIAN_POINT ( 'NONE',  ( -61.13531646874998415, 15.80729166632526628, 1.999225269531026417 ) ) ;
#8692=CARTESIAN_POINT ( 'NONE',  ( -61.99999999999998579, 14.03124999931720218, 0.3452994616207497591 ) ) ;
#8697=( BOUNDED_CURVE ( )  B_SPLINE_CURVE ( 2, ( #2303, #5687, #636, #9240, #1681, #4953, #6738, #8354, #684 ),
 .UNSPECIFIED., .F., .F. ) 
 B_SPLINE_CURVE_WITH_KNOTS ( ( 3, 2, 2, 2, 3 ),
 ( 0.2890624999999999445, 0.2916666666666666852, 0.2968750000000000000, 0.3020833333333333148, 0.3046875000000000000 ),
 .UNSPECIFIED. ) 
 CURVE ( )  GEOMETRIC_REPRESENTATION_ITEM ( )  RATIONAL_B_SPLINE_CURVE ( ( 0.9330127018922192983, 0.9330127018922178550, 1.000000000000000000, 0.8660254037844387076, 1.000000000000000000, 0.8660254037844387076, 1.000000000000000000, 0.9330127018922194093, 0.9330127018922194093 ) ) 
 REPRESENTATION_ITEM ( '' )  );
#8699=CARTESIAN_POINT ( 'NONE',  ( -61.13531646874997705, 11.30729166632526805, 1.999225269531026417 ) ) ;
#8700=CARTESIAN_POINT ( 'NONE',  ( -61.99999999999998579, 8.890624999658601979, 0.5015494609379544944 ) ) ;
#8702=CARTESIAN_POINT ( 'NONE',  ( -61.49999999999998579, 12.95833333333333215, 2.366025403784441927 ) ) ;
#8704=CARTESIAN_POINT ( 'NONE',  ( -62.99999999999998579, 10.62499999999999822, 1.500000000000001998 ) ) ;
#8705=CARTESIAN_POINT ( 'NONE',  ( -62.49999999999998579, 10.16666666666666785, 2.366025403784441483 ) ) ;
#8706=CARTESIAN_POINT ( 'NONE',  ( -62.86468353124998032, 14.24479166632526983, 1.000774730468978246 ) ) ;
#8707=CARTESIAN_POINT ( 'NONE',  ( -61.49999999999998579, 11.04166666666666607, 0.6339745962155628467 ) ) ;
#8708=CARTESIAN_POINT ( 'NONE',  ( -62.99999999999998579, 9.864583332650536107, 2.077350269189627952 ) ) ;
#8709=ADVANCED_FACE ( 'NONE', ( #4341 ), #6976, .T. ) ;
#8710=ORIENTED_EDGE ( 'NONE', *, *, #8550, .F. ) ;
#8714=CARTESIAN_POINT ( 'NONE',  ( -61.13531646874998415, 10.80729166632526628, 1.999225269531026417 ) ) ;
#8716=CARTESIAN_POINT ( 'NONE',  ( -62.86468353124998742, 10.53645833299193413, 1.999225269531025972 ) ) ;
#8717=CARTESIAN_POINT ( 'NONE',  ( -61.99999999999998579, 16.00000000000000000, 1.500000000000002220 ) ) ;
#8719=CARTESIAN_POINT ( 'NONE',  ( -62.86468353124999453, 14.01562499965860198, 1.500000000000002220 ) ) ;
#8721=ORIENTED_EDGE ( 'NONE', *, *, #7522, .T. ) ;
#8723=VECTOR ( 'NONE', #9298, 999.9999999999998863 ) ;
#8725=CARTESIAN_POINT ( 'NONE',  ( -61.99999999999998579, 15.15624999931720218, 2.500000000000002665 ) ) ;
#8726=CARTESIAN_POINT ( 'NONE',  ( -62.99999999999998579, 8.354166666666666075, 0.9226497308103756012 ) ) ;
#8727=CARTESIAN_POINT ( 'NONE',  ( -62.49999999999998579, 8.802083332650536107, 0.6339745962155627357 ) ) ;
#8729=CARTESIAN_POINT ( 'NONE',  ( -61.13531646874998415, 13.89062499965860198, 1.500000000000002220 ) ) ;
#8730=CARTESIAN_POINT ( 'NONE',  ( -62.86468353124998032, 8.682291666325268054, 1.000774730468978246 ) ) ;
#8731=CARTESIAN_POINT ( 'NONE',  ( -61.99999999999998579, 11.90624999931720041, 2.500000000000002665 ) ) ;
#8734=CARTESIAN_POINT ( 'NONE',  ( -62.43234176562498305, 10.72395833299193413, 0.7511620957034662593 ) ) ;
#8736=ORIENTED_EDGE ( 'NONE', *, *, #901, .T. ) ;
#8737=CARTESIAN_POINT ( 'NONE',  ( -61.49999999999998579, 13.92708333265053611, 2.366025403784441927 ) ) ;
#8741=CARTESIAN_POINT ( 'NONE',  ( -61.99999999999998579, 10.03124999931720218, 0.5000000000000013323 ) ) ;
#8742=CARTESIAN_POINT ( 'NONE',  ( -61.99999999999998579, 12.64062499965860198, 0.5015494609379544944 ) ) ;
#8745=CARTESIAN_POINT ( 'NONE',  ( -61.13531646874997705, 8.307291666325268054, 1.999225269531026417 ) ) ;
#8746=VERTEX_POINT ( 'NONE', #9644 ) ;
#8747=CARTESIAN_POINT ( 'NONE',  ( -62.49999999999998579, 15.83333333333333037, 0.6339745962155627357 ) ) ;
#8748=CARTESIAN_POINT ( 'NONE',  ( -61.99999999999999289, 9.703124999658601979, 0.5015494609379544944 ) ) ;
#8750=CARTESIAN_POINT ( 'NONE',  ( -62.43234176562498305, 15.16145833299193590, 0.7511620957034662593 ) ) ;
#8751=CARTESIAN_POINT ( 'NONE',  ( -60.99999999999998579, 13.96874999931720218, 1.500000000000002220 ) ) ;
#8756=FACE_OUTER_BOUND ( 'NONE', #9537, .T. ) ;
#8757=CARTESIAN_POINT ( 'NONE',  ( -61.13531646874997705, 12.59895833299193590, 1.000774730468978468 ) ) ;
#8758=CARTESIAN_POINT ( 'NONE',  ( -61.13531646874998415, 8.848958332991935904, 1.000774730468978468 ) ) ;
#8759=CARTESIAN_POINT ( 'NONE',  ( -61.99999999999998579, 13.06250000000000178, 0.5000000000000013323 ) ) ;
#8761=CARTESIAN_POINT ( 'NONE',  ( -61.99999999999998579, 12.43750000000000000, 2.654700538379254571 ) ) ;
#8763=DIRECTION ( 'NONE',  ( 0.000000000000000000, 0.000000000000000000, -1.000000000000000000 ) ) ;
#8764=CARTESIAN_POINT ( 'NONE',  ( -61.13531646874998415, 14.66145833299193590, 1.000774730468978468 ) ) ;
#8766=ADVANCED_FACE ( 'NONE', ( #482 ), #249, .T. ) ;
#8767=CARTESIAN_POINT ( 'NONE',  ( -60.99999999999998579, 10.46874999931720218, 1.500000000000002220 ) ) ;
#8769=( BOUNDED_CURVE ( )  B_SPLINE_CURVE ( 2, ( #6730, #7509, #1720, #4111, #9124, #2554, #7403, #10981, #2389 ),
 .UNSPECIFIED., .F., .T. ) 
 B_SPLINE_CURVE_WITH_KNOTS ( ( 3, 2, 2, 2, 3 ),
 ( 0.7109375000000000000, 0.7135416666666666297, 0.7187500000000000000, 0.7239583333333333703, 0.7265625000000000000 ),
 .UNSPECIFIED. ) 
 CURVE ( )  GEOMETRIC_REPRESENTATION_ITEM ( )  RATIONAL_B_SPLINE_CURVE ( ( 0.9330127018922194093, 0.9330127018922194093, 1.000000000000000000, 0.8660254037844387076, 1.000000000000000000, 0.8660254037844387076, 1.000000000000000000, 0.9330127018922194093, 0.9330127018922194093 ) ) 
 REPRESENTATION_ITEM ( '' )  );
#8772=CARTESIAN_POINT ( 'NONE',  ( -61.99999999999998579, 11.39062499965859843, 0.5015494609379544944 ) ) ;
#8775=CARTESIAN_POINT ( 'NONE',  ( -61.99999999999998579, 10.70312499965860198, 0.5015494609379544944 ) ) ;
#8776=CARTESIAN_POINT ( 'NONE',  ( -61.99999999999998579, 16.00000000000000000, -1.000000000000000000 ) ) ;
#8777=CARTESIAN_POINT ( 'NONE',  ( -62.43234176562498305, 14.72395833299193413, 0.7511620957034662593 ) ) ;
#8778=CARTESIAN_POINT ( 'NONE',  ( -61.73205080756886076, 8.917414549001833279, 2.500000000000003109 ) ) ;
#8780=CARTESIAN_POINT ( 'NONE',  ( -60.99999999999998579, 10.52083333333333393, 0.9226497308103762673 ) ) ;
#8781=VERTEX_POINT ( 'NONE', #8812 ) ;
#8782=DIRECTION ( 'NONE',  ( 0.000000000000000000, -0.000000000000000000, 1.000000000000000000 ) ) ;
#8783=CARTESIAN_POINT ( 'NONE',  ( -62.49999999999998579, 8.583333333333333925, 0.6339745962155627357 ) ) ;
#8786=CARTESIAN_POINT ( 'NONE',  ( -61.13531646874998415, 16.07812499965860198, 1.500000000000002220 ) ) ;
#8787=CARTESIAN_POINT ( 'NONE',  ( -62.43234176562499016, 14.55729166632526983, 2.248837904296538071 ) ) ;
#8788=CARTESIAN_POINT ( 'NONE',  ( -62.86468353124998032, 10.18229166632526805, 1.000774730468978246 ) ) ;
#8791=CARTESIAN_POINT ( 'NONE',  ( -61.56765823437498142, 10.93229166632526805, 0.7511620957034663704 ) ) ;
#8792=CARTESIAN_POINT ( 'NONE',  ( -61.13531646874998415, 16.14062499965860198, 1.500000000000002220 ) ) ;
#8795=DIRECTION ( 'NONE',  ( -0.000000000000000000, -1.000000000000000000, -0.000000000000000000 ) ) ;
#8796=ADVANCED_FACE ( 'NONE', ( #2929 ), #10829, .T. ) ;
#8798=LINE ( 'NONE', #7131, #4997 ) ;
#8799=CARTESIAN_POINT ( 'NONE',  ( -62.43234176562499016, 12.49479166632526805, 2.248837904296538071 ) ) ;
#8800=CARTESIAN_POINT ( 'NONE',  ( -61.13531646874997705, 9.307291666325268054, 1.999225269531026417 ) ) ;
#8803=CARTESIAN_POINT ( 'NONE',  ( -62.26794919243112503, 10.89508544963257464, 2.500000000000000000 ) ) ;
#8804=CARTESIAN_POINT ( 'NONE',  ( -62.86468353124999453, 10.03645833299193413, 1.999225269531025750 ) ) ;
#8805=CARTESIAN_POINT ( 'NONE',  ( -62.86468353124998742, 14.72395833299193413, 1.999225269531025972 ) ) ;
#8806=CARTESIAN_POINT ( 'NONE',  ( -62.99999999999998579, 14.32291666598387003, 0.9226497308103756012 ) ) ;
#8807=LINE ( 'NONE', #3033, #10712 ) ;
#8809=ORIENTED_EDGE ( 'NONE', *, *, #1848, .F. ) ;
#8810=ADVANCED_FACE ( 'NONE', ( #3803 ), #6184, .T. ) ;
#8811=CARTESIAN_POINT ( 'NONE',  ( -61.56765823437498852, 12.28645833299193413, 2.248837904296538515 ) ) ;
#8812=CARTESIAN_POINT ( 'NONE',  ( -61.99999999999998579, 14.65624999931720041, 2.500000000000002665 ) ) ;
#8813=CARTESIAN_POINT ( 'NONE',  ( -61.99999999999998579, 16.00000000000000000, 2.500000000000000444 ) ) ;
#8815=CARTESIAN_POINT ( 'NONE',  ( -62.49999999999998579, 12.41666666666666607, 2.366025403784441483 ) ) ;
#8816=CARTESIAN_POINT ( 'NONE',  ( -62.26794919243111082, 10.17633545031537068, 2.500000000000003109 ) ) ;
#8817=CARTESIAN_POINT ( 'NONE',  ( -61.13531646874998415, 14.61979166632526805, 1.999225269531026417 ) ) ;
#8818=LINE ( 'NONE', #1202, #10629 ) ;
#8819=CARTESIAN_POINT ( 'NONE',  ( -60.99999999999998579, 11.19791666598387003, 2.077350269189628840 ) ) ;
#8820=EDGE_LOOP ( 'NONE', ( #521, #6863, #10545, #6883 ) ) ;
#8821=CARTESIAN_POINT ( 'NONE',  ( -61.99999999999998579, 16.00000000000000000, 1.500000000000002220 ) ) ;
#8822=EDGE_CURVE ( 'NONE', #2668, #3478, #5334, .T. ) ;
#8823=CARTESIAN_POINT ( 'NONE',  ( -61.99999999999998579, 14.31250000000000000, 0.5000000000000013323 ) ) ;
#8824=CARTESIAN_POINT ( 'NONE',  ( -61.13531646874998415, 12.59895833299193590, 1.000774730468978468 ) ) ;
#8827=ORIENTED_EDGE ( 'NONE', *, *, #3433, .F. ) ;
#8828=CARTESIAN_POINT ( 'NONE',  ( -62.43234176562498305, 10.47395833299193413, 0.7511620957034662593 ) ) ;
#8829=( BOUNDED_CURVE ( )  B_SPLINE_CURVE ( 2, ( #4569, #533, #8033, #10523, #3917, #7307, #9026, #3682, #9327 ),
 .UNSPECIFIED., .F., .T. ) 
 B_SPLINE_CURVE_WITH_KNOTS ( ( 3, 2, 2, 2, 3 ),
 ( 0.9765625000000000000, 0.9791666666666666297, 0.9843750000000000000, 0.9895833333333333703, 0.9921875000000000000 ),
 .UNSPECIFIED. ) 
 CURVE ( )  GEOMETRIC_REPRESENTATION_ITEM ( )  RATIONAL_B_SPLINE_CURVE ( ( 0.9330127018922194093, 0.9330127018922194093, 1.000000000000000000, 0.8660254037844387076, 1.000000000000000000, 0.8660254037844387076, 1.000000000000000000, 0.9330127018922194093, 0.9330127018922194093 ) ) 
 REPRESENTATION_ITEM ( '' )  );
#8830=DIRECTION ( 'NONE',  ( 0.000000000000000000, 0.000000000000000000, -1.000000000000000000 ) ) ;
#8831=CARTESIAN_POINT ( 'NONE',  ( -62.86468353124998032, 14.24479166632526983, 1.000774730468978246 ) ) ;
#8833=VERTEX_POINT ( 'NONE', #8971 ) ;
#8836=CARTESIAN_POINT ( 'NONE',  ( -62.26794919243111082, 15.04241454900182973, 0.5000000000000013323 ) ) ;
#8837=CARTESIAN_POINT ( 'NONE',  ( -62.86468353124998742, 15.97395833299193590, 1.999225269531025972 ) ) ;
#8838=DIRECTION ( 'NONE',  ( -0.000000000000000000, -1.000000000000000000, -0.000000000000000000 ) ) ;
#8839=CARTESIAN_POINT ( 'NONE',  ( -61.99999999999998579, 15.53124999931720041, 0.5000000000000013323 ) ) ;
#8840=CARTESIAN_POINT ( 'NONE',  ( -61.99999999999998579, 10.78124999931720218, 0.5000000000000013323 ) ) ;
#8841=CARTESIAN_POINT ( 'NONE',  ( -61.99999999999999289, 14.95312499965860198, 0.5015494609379544944 ) ) ;
#8842=CARTESIAN_POINT ( 'NONE',  ( -61.56765823437498142, 10.11979166632526805, 0.7511620957034663704 ) ) ;
#8843=CARTESIAN_POINT ( 'NONE',  ( -61.99999999999998579, 9.437499999999998224, 2.500000000000002665 ) ) ;
#8845=CARTESIAN_POINT ( 'NONE',  ( -62.86468353124999453, 11.01562499965860020, 1.500000000000002220 ) ) ;
#8846=LINE ( 'NONE', #9620, #2180 ) ;
#8854=CARTESIAN_POINT ( 'NONE',  ( -60.99999999999998579, 10.02083333333333215, 0.9226497308103762673 ) ) ;
#8855=CARTESIAN_POINT ( 'NONE',  ( -62.86468353124998742, 12.72395833299193413, 1.999225269531025972 ) ) ;
#8857=CARTESIAN_POINT ( 'NONE',  ( -61.13531646874997705, 9.807291666325268054, 1.999225269531026417 ) ) ;
#8858=CARTESIAN_POINT ( 'NONE',  ( -61.99999999999998579, 16.00000000000000000, 2.500000000000000444 ) ) ;
#8860=CARTESIAN_POINT ( 'NONE',  ( -62.86468353124999453, 12.03645833299193413, 1.999225269531025750 ) ) ;
#8862=CARTESIAN_POINT ( 'NONE',  ( -62.43234176562498305, 15.66145833299193590, 0.7511620957034662593 ) ) ;
#8863=EDGE_CURVE ( 'NONE', #3037, #6239, #3728, .T. ) ;
#8864=CARTESIAN_POINT ( 'NONE',  ( -61.49999999999998579, 14.76041666598386826, 0.6339745962155628467 ) ) ;
#8866=ORIENTED_EDGE ( 'NONE', *, *, #6873, .T. ) ;
#8870=CARTESIAN_POINT ( 'NONE',  ( -62.86468353124999453, 12.97395833299193413, 1.999225269531025750 ) ) ;
#8871=CARTESIAN_POINT ( 'NONE',  ( -61.13531646874998415, 9.078124999658601979, 1.500000000000002220 ) ) ;
#8873=VERTEX_POINT ( 'NONE', #5574 ) ;
#8874=CARTESIAN_POINT ( 'NONE',  ( -61.49999999999998579, 12.29166666666666607, 0.6339745962155628467 ) ) ;
#8875=CARTESIAN_POINT ( 'NONE',  ( -61.99999999999998579, 15.90624999931719863, 2.500000000000002665 ) ) ;
#8877=CARTESIAN_POINT ( 'NONE',  ( -62.43234176562498305, 14.47395833299193413, 0.7511620957034662593 ) ) ;
#8879=CYLINDRICAL_SURFACE ( 'NONE', #10802, 0.9999999999999981126 ) ;
#8880=CARTESIAN_POINT ( 'NONE',  ( -60.99999999999998579, 10.96874999931720218, 1.500000000000002220 ) ) ;
#8883=VECTOR ( 'NONE', #5828, 1000.000000000000000 ) ;
#8884=CARTESIAN_POINT ( 'NONE',  ( -62.43234176562498305, 12.91145833299193590, 0.7511620957034662593 ) ) ;
#8885=EDGE_CURVE ( 'NONE', #1879, #4030, #1463, .T. ) ;
#8888=VERTEX_POINT ( 'NONE', #3027 ) ;
#8890=CARTESIAN_POINT ( 'NONE',  ( -61.99999999999998579, 10.32812499965860020, 2.498450539062049724 ) ) ;
#8892=CARTESIAN_POINT ( 'NONE',  ( -62.43234176562498305, 15.22395833299193590, 0.7511620957034662593 ) ) ;
#8894=EDGE_LOOP ( 'NONE', ( #8827, #3185, #6207, #3351 ) ) ;
#8895=CARTESIAN_POINT ( 'NONE',  ( -62.99999999999998579, 9.395833333333333925, 2.077350269189627952 ) ) ;
#8896=ORIENTED_EDGE ( 'NONE', *, *, #9592, .F. ) ;
#8897=CARTESIAN_POINT ( 'NONE',  ( -61.49999999999998579, 8.708333333333333925, 2.366025403784441927 ) ) ;
#8898=CARTESIAN_POINT ( 'NONE',  ( -61.49999999999998579, 10.04166666666666785, 0.6339745962155628467 ) ) ;
#8900=CARTESIAN_POINT ( 'NONE',  ( -61.99999999999998579, 9.812500000000000000, 0.5000000000000013323 ) ) ;
#8902=CARTESIAN_POINT ( 'NONE',  ( -61.13531646874998415, 9.848958332991934128, 1.000774730468978468 ) ) ;
#8903=LINE ( 'NONE', #9558, #7099 ) ;
#8904=CARTESIAN_POINT ( 'NONE',  ( -61.99999999999998579, 16.00000000000000000, 1.500000000000002220 ) ) ;
#8905=EDGE_CURVE ( 'NONE', #7083, #312, #7491, .T. ) ;
#8906=CARTESIAN_POINT ( 'NONE',  ( -61.13531646874998415, 10.16145833299193413, 1.000774730468978468 ) ) ;
#8907=CARTESIAN_POINT ( 'NONE',  ( -61.99999999999998579, 13.68749999999999822, 2.500000000000002665 ) ) ;
#8909=CARTESIAN_POINT ( 'NONE',  ( -61.99999999999998579, 13.40624999931720041, 2.500000000000002665 ) ) ;
#8910=DIRECTION ( 'NONE',  ( -0.000000000000000000, -1.000000000000000000, -0.000000000000000000 ) ) ;
#8913=CARTESIAN_POINT ( 'NONE',  ( -60.99999999999998579, 10.19791666598387181, 2.077350269189628840 ) ) ;
#8914=CARTESIAN_POINT ( 'NONE',  ( -62.43234176562498305, 12.91145833299193590, 0.7511620957034662593 ) ) ;
#8915=CARTESIAN_POINT ( 'NONE',  ( -61.99999999999999289, 9.765624999658600203, 2.498450539062049724 ) ) ;
#8919=CARTESIAN_POINT ( 'NONE',  ( -61.13531646874997705, 11.61979166632526805, 1.999225269531026417 ) ) ;
#8921=CARTESIAN_POINT ( 'NONE',  ( -61.99999999999998579, 14.64062499965860020, 0.5015494609379544944 ) ) ;
#8922=CARTESIAN_POINT ( 'NONE',  ( -60.99999999999998579, 14.46874999931720218, 1.500000000000002220 ) ) ;
#8923=CARTESIAN_POINT ( 'NONE',  ( -61.73205080756886076, 14.77008544963257108, 0.5000000000000014433 ) ) ;
#8927=CARTESIAN_POINT ( 'NONE',  ( -61.99999999999999289, 13.14062499965860198, 0.5015494609379544944 ) ) ;
#8928=CARTESIAN_POINT ( 'NONE',  ( -61.13531646874998415, 8.578124999658601979, 1.500000000000002220 ) ) ;
#8929=CARTESIAN_POINT ( 'NONE',  ( -62.26794919243112503, 10.64508544963257464, 2.500000000000000000 ) ) ;
#8931=CARTESIAN_POINT ( 'NONE',  ( -60.99999999999998579, 11.97916666666666785, 2.077350269189628840 ) ) ;
#8932=CARTESIAN_POINT ( 'NONE',  ( -62.99999999999998579, 13.34374999931720396, 1.500000000000001998 ) ) ;
#8933=( BOUNDED_CURVE ( )  B_SPLINE_CURVE ( 2, ( #9529, #1811, #4409, #138, #8643, #5414, #1922, #2701, #2875 ),
 .UNSPECIFIED., .F., .F. ) 
 B_SPLINE_CURVE_WITH_KNOTS ( ( 3, 2, 2, 2, 3 ),
 ( 0.2734375000000000000, 0.2760416666666666852, 0.2812500000000000000, 0.2864583333333333148, 0.2890624999999999445 ),
 .UNSPECIFIED. ) 
 CURVE ( )  GEOMETRIC_REPRESENTATION_ITEM ( )  RATIONAL_B_SPLINE_CURVE ( ( 0.9330127018922194093, 0.9330127018922194093, 1.000000000000000000, 0.8660254037844387076, 1.000000000000000000, 0.8660254037844387076, 1.000000000000000000, 0.9330127018922207416, 0.9330127018922192983 ) ) 
 REPRESENTATION_ITEM ( '' )  );
#8937=CARTESIAN_POINT ( 'NONE',  ( -60.99999999999998579, 10.71874999931720396, 1.500000000000002220 ) ) ;
#8940=VECTOR ( 'NONE', #3222, 1000.000000000000000 ) ;
#8941=CARTESIAN_POINT ( 'NONE',  ( -62.43234176562499016, 12.49479166632526805, 2.248837904296538071 ) ) ;
#8943=VERTEX_POINT ( 'NONE', #4888 ) ;
#8944=CARTESIAN_POINT ( 'NONE',  ( -62.43234176562499016, 11.30729166632526805, 2.248837904296538071 ) ) ;
#8945=FACE_OUTER_BOUND ( 'NONE', #6515, .T. ) ;
#8947=CARTESIAN_POINT ( 'NONE',  ( -61.56765823437498852, 15.34895833299193590, 2.248837904296538515 ) ) ;
#8948=CARTESIAN_POINT ( 'NONE',  ( -60.99999999999998579, 8.968749999317203958, 1.500000000000002220 ) ) ;
#8949=ORIENTED_EDGE ( 'NONE', *, *, #8005, .F. ) ;
#8950=CARTESIAN_POINT ( 'NONE',  ( -61.99999999999998579, 16.00000000000000000, 1.500000000000002220 ) ) ;
#8951=ADVANCED_FACE ( 'NONE', ( #7303 ), #10840, .F. ) ;
#8953=LINE ( 'NONE', #3892, #5172 ) ;
#8954=CARTESIAN_POINT ( 'NONE',  ( -60.99999999999998579, 10.25000000000000000, 1.500000000000002220 ) ) ;
#8956=CARTESIAN_POINT ( 'NONE',  ( -61.73205080756886076, 11.94866454968463110, 2.500000000000003109 ) ) ;
#8957=FACE_OUTER_BOUND ( 'NONE', #7926, .T. ) ;
#8958=CARTESIAN_POINT ( 'NONE',  ( -62.43234176562499016, 9.744791666325268054, 2.248837904296538071 ) ) ;
#8959=CARTESIAN_POINT ( 'NONE',  ( -62.26794919243111082, 15.89508544963257108, 2.500000000000003109 ) ) ;
#8960=CARTESIAN_POINT ( 'NONE',  ( -61.13531646874998415, 12.14062499965860198, 1.500000000000002220 ) ) ;
#8966=CARTESIAN_POINT ( 'NONE',  ( -62.49999999999998579, 10.38541666598387003, 2.366025403784441483 ) ) ;
#8968=CARTESIAN_POINT ( 'NONE',  ( -62.86468353124999453, 13.95312499965860198, 1.500000000000002220 ) ) ;
#8969=CARTESIAN_POINT ( 'NONE',  ( -61.99999999999999289, 10.01562499965860198, 2.498450539062049724 ) ) ;
#8970=ORIENTED_EDGE ( 'NONE', *, *, #4046, .T. ) ;
#8971=CARTESIAN_POINT ( 'NONE',  ( -61.99999999999998579, 15.28124999931720218, 0.5000000000000013323 ) ) ;
#8972=CARTESIAN_POINT ( 'NONE',  ( -61.13531646874998415, 11.39062499965860020, 1.500000000000002220 ) ) ;
#8974=DIRECTION ( 'NONE',  ( -0.000000000000000000, -1.000000000000000000, -0.000000000000000000 ) ) ;
#8975=CARTESIAN_POINT ( 'NONE',  ( -61.99999999999998579, 15.90624999931720396, 2.654700538379254571 ) ) ;
#8980=CARTESIAN_POINT ( 'NONE',  ( -62.43234176562498305, 12.91145833299193590, 0.7511620957034662593 ) ) ;
#8981=CARTESIAN_POINT ( 'NONE',  ( -61.99999999999998579, 9.515624999658601979, 2.498450539062049724 ) ) ;
#8982=CARTESIAN_POINT ( 'NONE',  ( -62.99999999999998579, 8.395833333333333925, 2.077350269189627952 ) ) ;
#8984=CARTESIAN_POINT ( 'NONE',  ( -60.99999999999998579, 12.97916666666666785, 2.077350269189628840 ) ) ;
#8985=CARTESIAN_POINT ( 'NONE',  ( -62.99999999999998579, 13.32291666598387003, 0.9226497308103756012 ) ) ;
#8987=CARTESIAN_POINT ( 'NONE',  ( -61.49999999999998579, 10.01041666598387003, 0.6339745962155628467 ) ) ;
#8989=CARTESIAN_POINT ( 'NONE',  ( -61.56765823437498852, 13.28645833299193413, 2.248837904296538515 ) ) ;
#8990=CARTESIAN_POINT ( 'NONE',  ( -61.99999999999998579, 8.312499999999998224, 0.5000000000000013323 ) ) ;
#8991=( BOUNDED_CURVE ( )  B_SPLINE_CURVE ( 2, ( #6731, #7404, #7461, #10104, #8192, #10786, #5622, #2390, #3963 ),
 .UNSPECIFIED., .F., .T. ) 
 B_SPLINE_CURVE_WITH_KNOTS ( ( 3, 2, 2, 2, 3 ),
 ( 0.007812499999999973112, 0.01041666666666666609, 0.01562500000000000000, 0.02083333333333333218, 0.02343749999999996531 ),
 .UNSPECIFIED. ) 
 CURVE ( )  GEOMETRIC_REPRESENTATION_ITEM ( )  RATIONAL_B_SPLINE_CURVE ( ( 0.9330127018922194093, 0.9330127018922187432, 1.000000000000000000, 0.8660254037844387076, 1.000000000000000000, 0.8660254037844387076, 1.000000000000000000, 0.9330127018922202975, 0.9330127018922194093 ) ) 
 REPRESENTATION_ITEM ( '' )  );
#8993=CARTESIAN_POINT ( 'NONE',  ( -61.99999999999998579, 11.32812499965860020, 2.498450539062049724 ) ) ;
#8994=CARTESIAN_POINT ( 'NONE',  ( -60.99999999999998579, 12.19791666598386826, 2.077350269189628840 ) ) ;
#8995=EDGE_CURVE ( 'NONE', #1159, #6239, #5624, .T. ) ;
#8996=CARTESIAN_POINT ( 'NONE',  ( -62.86468353124999453, 15.51562499965860198, 1.500000000000002220 ) ) ;
#9000=CARTESIAN_POINT ( 'NONE',  ( -61.99999999999998579, 8.656249999317202182, 2.500000000000002665 ) ) ;
#9001=CARTESIAN_POINT ( 'NONE',  ( -62.49999999999998579, 9.583333333333332149, 0.6339745962155627357 ) ) ;
#9004=CARTESIAN_POINT ( 'NONE',  ( -61.99999999999998579, 8.187500000000001776, 2.500000000000003109 ) ) ;
#9006=CARTESIAN_POINT ( 'NONE',  ( -62.86468353124998032, 12.49479166632526628, 1.000774730468978246 ) ) ;
#9008=CARTESIAN_POINT ( 'NONE',  ( -60.99999999999998579, 9.239583332650536107, 0.9226497308103762673 ) ) ;
#9009=FACE_OUTER_BOUND ( 'NONE', #8377, .T. ) ;
#9013=CARTESIAN_POINT ( 'NONE',  ( -61.99999999999998579, 14.15624999931720218, 2.500000000000002665 ) ) ;
#9014=EDGE_CURVE ( 'NONE', #6754, #1879, #4862, .T. ) ;
#9015=CARTESIAN_POINT ( 'NONE',  ( -62.43234176562499016, 14.24479166632526983, 2.248837904296538071 ) ) ;
#9016=CARTESIAN_POINT ( 'NONE',  ( -61.99999999999999289, 9.890624999658601979, 0.5015494609379544944 ) ) ;
#9018=EDGE_LOOP ( 'NONE', ( #3870, #9585 ) ) ;
#9020=CARTESIAN_POINT ( 'NONE',  ( -61.56765823437498142, 11.43229166632526805, 0.7511620957034663704 ) ) ;
#9025=CARTESIAN_POINT ( 'NONE',  ( -60.99999999999998579, 15.48958333265053788, 0.9226497308103762673 ) ) ;
#9026=CARTESIAN_POINT ( 'NONE',  ( -62.49999999999998579, 16.13541666598386826, 2.366025403784441483 ) ) ;
#9029=DIRECTION ( 'NONE',  ( 0.000000000000000000, 0.000000000000000000, 1.000000000000000000 ) ) ;
#9030=CARTESIAN_POINT ( 'NONE',  ( -61.13531646874998415, 14.57812499965860020, 1.500000000000002220 ) ) ;
#9031=CARTESIAN_POINT ( 'NONE',  ( -61.56765823437498852, 10.28645833299193413, 2.248837904296538515 ) ) ;
#9033=CARTESIAN_POINT ( 'NONE',  ( -61.99999999999998579, 16.00000000000000000, 2.500000000000000444 ) ) ;
#9034=ORIENTED_EDGE ( 'NONE', *, *, #10288, .T. ) ;
#9035=CARTESIAN_POINT ( 'NONE',  ( -60.99999999999998579, 14.27083333333333393, 0.9226497308103762673 ) ) ;
#9039=CARTESIAN_POINT ( 'NONE',  ( -62.99999999999998579, 11.36458333265053611, 2.077350269189627952 ) ) ;
#9042=CARTESIAN_POINT ( 'NONE',  ( -62.99999999999998579, 14.87500000000000000, 1.500000000000001998 ) ) ;
#9043=CARTESIAN_POINT ( 'NONE',  ( -61.13531646874998415, 12.07812499965860198, 1.500000000000002220 ) ) ;
#9046=CARTESIAN_POINT ( 'NONE',  ( -61.13531646874998415, 11.36979166632526628, 1.999225269531026417 ) ) ;
#9050=CARTESIAN_POINT ( 'NONE',  ( -62.43234176562499016, 15.80729166632526628, 2.248837904296538071 ) ) ;
#9055=( BOUNDED_CURVE ( )  B_SPLINE_CURVE ( 2, ( #3993, #9941, #6613, #561, #10723, #8118, #7282, #9992, #5762 ),
 .UNSPECIFIED., .F., .F. ) 
 B_SPLINE_CURVE_WITH_KNOTS ( ( 3, 2, 2, 2, 3 ),
 ( 0.3828125000000000000, 0.3854166666666666852, 0.3906250000000000000, 0.3958333333333333148, 0.3984375000000000000 ),
 .UNSPECIFIED. ) 
 CURVE ( )  GEOMETRIC_REPRESENTATION_ITEM ( )  RATIONAL_B_SPLINE_CURVE ( ( 0.9330127018922194093, 0.9330127018922194093, 1.000000000000000000, 0.8660254037844387076, 1.000000000000000000, 0.8660254037844387076, 1.000000000000000000, 0.9330127018922194093, 0.9330127018922194093 ) ) 
 REPRESENTATION_ITEM ( '' )  );
#9058=EDGE_CURVE ( 'NONE', #7667, #8833, #2443, .T. ) ;
#9059=CARTESIAN_POINT ( 'NONE',  ( -62.49999999999998579, 10.41666666666666785, 2.366025403784441483 ) ) ;
#9060=VECTOR ( 'NONE', #3208, 1000.000000000000000 ) ;
#9062=DIRECTION ( 'NONE',  ( -0.000000000000000000, -1.000000000000000000, -0.000000000000000000 ) ) ;
#9063=CARTESIAN_POINT ( 'NONE',  ( -62.49999999999998579, 14.88541666598386826, 2.366025403784441483 ) ) ;
#9064=CARTESIAN_POINT ( 'NONE',  ( -60.99999999999998579, 8.489583332650536107, 0.9226497308103762673 ) ) ;
#9065=CARTESIAN_POINT ( 'NONE',  ( -61.13531646874998415, 11.61979166632526983, 1.999225269531026417 ) ) ;
#9066=CARTESIAN_POINT ( 'NONE',  ( -61.99999999999998579, 10.56249999999999822, 0.5000000000000013323 ) ) ;
#9068=FACE_OUTER_BOUND ( 'NONE', #967, .T. ) ;
#9071=CARTESIAN_POINT ( 'NONE',  ( -62.86468353124999453, 14.45312499965860020, 1.500000000000002220 ) ) ;
#9072=CARTESIAN_POINT ( 'NONE',  ( -61.56765823437498142, 9.869791666325268054, 0.7511620957034663704 ) ) ;
#9074=CARTESIAN_POINT ( 'NONE',  ( -62.99999999999998579, 14.12499999999999822, 1.500000000000001998 ) ) ;
#9075=CARTESIAN_POINT ( 'NONE',  ( -61.99999999999999289, 11.20312499965859843, 0.5015494609379544944 ) ) ;
#9076=CARTESIAN_POINT ( 'NONE',  ( -62.43234176562499016, 16.05729166632526628, 2.248837904296538071 ) ) ;
#9078=CARTESIAN_POINT ( 'NONE',  ( -61.13531646874998415, 16.05729166632526983, 1.999225269531026417 ) ) ;
#9079=CARTESIAN_POINT ( 'NONE',  ( -61.56765823437498142, 8.432291666325268054, 0.7511620957034663704 ) ) ;
#9080=FACE_OUTER_BOUND ( 'NONE', #4830, .T. ) ;
#9081=VERTEX_POINT ( 'NONE', #1363 ) ;
#9082=CARTESIAN_POINT ( 'NONE',  ( -61.99999999999998579, 16.00000000000000000, 2.500000000000000444 ) ) ;
#9084=EDGE_CURVE ( 'NONE', #3958, #7755, #8140, .T. ) ;
#9086=CARTESIAN_POINT ( 'NONE',  ( -61.13531646874998415, 13.82812499965860198, 1.500000000000002220 ) ) ;
#9087=CARTESIAN_POINT ( 'NONE',  ( -61.56765823437498852, 10.03645833299193413, 2.248837904296538515 ) ) ;
#9088=LINE ( 'NONE', #2406, #2878 ) ;
#9090=CARTESIAN_POINT ( 'NONE',  ( -60.99999999999998579, 14.24999999999999822, 1.500000000000002220 ) ) ;
#9091=CARTESIAN_POINT ( 'NONE',  ( -61.99999999999998579, 9.062500000000000000, 0.5000000000000013323 ) ) ;
#9092=CARTESIAN_POINT ( 'NONE',  ( -62.49999999999998579, 12.38541666598386826, 2.366025403784441483 ) ) ;
#9093=AXIS2_PLACEMENT_3D ( 'NONE', #10112, #10946, #1471 ) ;
#9094=CARTESIAN_POINT ( 'NONE',  ( -62.43234176562498305, 14.41145833299193413, 0.7511620957034662593 ) ) ;
#9096=EDGE_LOOP ( 'NONE', ( #9646, #5776, #8267, #5984 ) ) ;
#9100=CARTESIAN_POINT ( 'NONE',  ( -62.86468353124999453, 11.26562499965860020, 1.500000000000002220 ) ) ;
#9101=CARTESIAN_POINT ( 'NONE',  ( -61.99999999999998579, 15.03124999931720218, 0.5000000000000013323 ) ) ;
#9102=CARTESIAN_POINT ( 'NONE',  ( -61.13531646874998415, 15.66145833299193590, 1.000774730468978468 ) ) ;
#9103=ORIENTED_EDGE ( 'NONE', *, *, #1371, .T. ) ;
#9107=CARTESIAN_POINT ( 'NONE',  ( -62.26794919243111082, 9.895085449632572860, 2.500000000000003109 ) ) ;
#9108=CARTESIAN_POINT ( 'NONE',  ( -61.49999999999998579, 9.541666666666667851, 0.6339745962155628467 ) ) ;
#9110=CARTESIAN_POINT ( 'NONE',  ( -61.73205080756886076, 15.02008544963257108, 0.5000000000000014433 ) ) ;
#9113=CYLINDRICAL_SURFACE ( 'NONE', #4406, 0.9999999999999981126 ) ;
#9114=CARTESIAN_POINT ( 'NONE',  ( -61.99999999999998579, 11.70312499965860020, 0.5015494609379544944 ) ) ;
#9115=CARTESIAN_POINT ( 'NONE',  ( -62.26794919243111082, 9.042414549001833279, 0.4999999999999998890 ) ) ;
#9116=ORIENTED_EDGE ( 'NONE', *, *, #6084, .F. ) ;
#9117=( BOUNDED_CURVE ( )  B_SPLINE_CURVE ( 2, ( #9066, #7453, #4103, #6622, #6671, #4829, #7502, #8236, #10885 ),
 .UNSPECIFIED., .F., .F. ) 
 B_SPLINE_CURVE_WITH_KNOTS ( ( 3, 2, 2, 2, 3 ),
 ( 0.3203125000000000000, 0.3229166666666666852, 0.3281250000000000000, 0.3333333333333333148, 0.3359374999999999445 ),
 .UNSPECIFIED. ) 
 CURVE ( )  GEOMETRIC_REPRESENTATION_ITEM ( )  RATIONAL_B_SPLINE_CURVE ( ( 0.9330127018922194093, 0.9330127018922194093, 1.000000000000000000, 0.8660254037844387076, 1.000000000000000000, 0.8660254037844387076, 1.000000000000000000, 0.9330127018922207416, 0.9330127018922192983 ) ) 
 REPRESENTATION_ITEM ( '' )  );
#9119=EDGE_CURVE ( 'NONE', #8372, #5268, #10544, .T. ) ;
#9122=CARTESIAN_POINT ( 'NONE',  ( -61.99999999999998579, 16.00000000000000000, 1.500000000000002220 ) ) ;
#9123=CARTESIAN_POINT ( 'NONE',  ( -61.99999999999998579, 13.26562499965860198, 2.498450539062049724 ) ) ;
#9124=CARTESIAN_POINT ( 'NONE',  ( -60.99999999999998579, 13.75000000000000000, 1.500000000000002220 ) ) ;
#9125=CARTESIAN_POINT ( 'NONE',  ( -60.99999999999998579, 14.47916666666666607, 2.077350269189628840 ) ) ;
#9127=CARTESIAN_POINT ( 'NONE',  ( -61.13531646874998415, 12.89062499965860198, 1.500000000000002220 ) ) ;
#9128=CARTESIAN_POINT ( 'NONE',  ( -61.13531646874998415, 15.89062499965860198, 1.500000000000002220 ) ) ;
#9131=CARTESIAN_POINT ( 'NONE',  ( -60.99999999999998579, 15.44791666598386826, 2.077350269189628840 ) ) ;
#9135=EDGE_CURVE ( 'NONE', #10734, #5253, #10265, .T. ) ;
#9137=CARTESIAN_POINT ( 'NONE',  ( -61.56765823437498852, 14.78645833299193413, 2.248837904296538515 ) ) ;
#9138=CARTESIAN_POINT ( 'NONE',  ( -62.43234176562499016, 9.494791666325268054, 2.248837904296538071 ) ) ;
#9139=CARTESIAN_POINT ( 'NONE',  ( -62.86468353124998032, 15.74479166632526628, 1.000774730468978024 ) ) ;
#9141=ORIENTED_EDGE ( 'NONE', *, *, #5613, .F. ) ;
#9142=CARTESIAN_POINT ( 'NONE',  ( -62.49999999999998579, 13.83333333333333215, 0.6339745962155627357 ) ) ;
#9145=CARTESIAN_POINT ( 'NONE',  ( -60.99999999999998579, 11.94791666598387181, 2.077350269189628840 ) ) ;
#9146=ADVANCED_FACE ( 'NONE', ( #10325 ), #9233, .T. ) ;
#9147=CARTESIAN_POINT ( 'NONE',  ( -61.99999999999998579, 9.562500000000000000, 0.5000000000000013323 ) ) ;
#9148=CARTESIAN_POINT ( 'NONE',  ( -61.13531646874998415, 14.57812499965860020, 1.500000000000002220 ) ) ;
#9150=ORIENTED_EDGE ( 'NONE', *, *, #3313, .F. ) ;
#9152=CARTESIAN_POINT ( 'NONE',  ( -62.43234176562498305, 11.47395833299193590, 0.7511620957034662593 ) ) ;
#9153=CARTESIAN_POINT ( 'NONE',  ( -61.99999999999998579, 12.28124999931720041, 0.5000000000000013323 ) ) ;
#9160=CARTESIAN_POINT ( 'NONE',  ( -61.99999999999998579, 8.531249999317203958, 0.5000000000000013323 ) ) ;
#9161=CARTESIAN_POINT ( 'NONE',  ( -61.49999999999998579, 10.54166666666666607, 0.6339745962155628467 ) ) ;
#9162=DIRECTION ( 'NONE',  ( -0.000000000000000000, -1.000000000000000000, -0.000000000000000000 ) ) ;
#9163=DIRECTION ( 'NONE',  ( -0.000000000000000000, -1.000000000000000000, -0.000000000000000000 ) ) ;
#9165=CARTESIAN_POINT ( 'NONE',  ( -60.99999999999998579, 9.447916665983868256, 2.077350269189628840 ) ) ;
#9166=CARTESIAN_POINT ( 'NONE',  ( -62.86468353124999453, 11.51562499965860020, 1.500000000000002220 ) ) ;
#9169=CARTESIAN_POINT ( 'NONE',  ( -62.99999999999998579, 15.37500000000000000, 1.500000000000001998 ) ) ;
#9171=CYLINDRICAL_SURFACE ( 'NONE', #10868, 0.9999999999999981126 ) ;
#9172=CARTESIAN_POINT ( 'NONE',  ( -62.43234176562499016, 13.74479166632526805, 2.248837904296538071 ) ) ;
#9175=CARTESIAN_POINT ( 'NONE',  ( -62.99999999999998579, 8.343749999317202182, 1.500000000000001998 ) ) ;
#9176=CARTESIAN_POINT ( 'NONE',  ( -61.56765823437498852, 13.34895833299193413, 2.248837904296538515 ) ) ;
#9177=CARTESIAN_POINT ( 'NONE',  ( -61.99999999999998579, 15.07812499965860198, 2.498450539062049724 ) ) ;
#9179=( BOUNDED_CURVE ( )  B_SPLINE_CURVE ( 2, ( #546, #5590, #6543, #3196, #7263, #9760, #5696, #2156, #9091 ),
 .UNSPECIFIED., .F., .T. ) 
 B_SPLINE_CURVE_WITH_KNOTS ( ( 3, 2, 2, 2, 3 ),
 ( 0.1171875000000000278, 0.1197916666666666713, 0.1250000000000000000, 0.1302083333333333426, 0.1328125000000000000 ),
 .UNSPECIFIED. ) 
 CURVE ( )  GEOMETRIC_REPRESENTATION_ITEM ( )  RATIONAL_B_SPLINE_CURVE ( ( 0.9330127018922194093, 0.9330127018922200755, 1.000000000000000000, 0.8660254037844387076, 1.000000000000000000, 0.8660254037844387076, 1.000000000000000000, 0.9330127018922194093, 0.9330127018922194093 ) ) 
 REPRESENTATION_ITEM ( '' )  );
#9181=FACE_OUTER_BOUND ( 'NONE', #10404, .T. ) ;
#9183=CARTESIAN_POINT ( 'NONE',  ( -62.99999999999998579, 16.07291666598386826, 0.9226497308103756012 ) ) ;
#9184=CYLINDRICAL_SURFACE ( 'NONE', #7664, 0.9999999999999981126 ) ;
#9189=CARTESIAN_POINT ( 'NONE',  ( -61.56765823437498142, 14.11979166632526805, 0.7511620957034663704 ) ) ;
#9190=CARTESIAN_POINT ( 'NONE',  ( -61.56765823437498142, 9.869791666325268054, 0.7511620957034663704 ) ) ;
#9191=AXIS2_PLACEMENT_3D ( 'NONE', #7322, #9984, #4810 ) ;
#9192=CARTESIAN_POINT ( 'NONE',  ( -61.99999999999999289, 15.45312499965860020, 0.5015494609379544944 ) ) ;
#9193=CARTESIAN_POINT ( 'NONE',  ( -61.99999999999998579, 14.40624999931720218, 2.500000000000002665 ) ) ;
#9194=ORIENTED_EDGE ( 'NONE', *, *, #2423, .T. ) ;
#9195=CARTESIAN_POINT ( 'NONE',  ( -62.99999999999998579, 13.39583333333333393, 2.077350269189627952 ) ) ;
#9198=CARTESIAN_POINT ( 'NONE',  ( -61.56765823437498852, 9.098958332991935904, 2.248837904296538515 ) ) ;
#9199=CARTESIAN_POINT ( 'NONE',  ( -61.99999999999998579, 11.78124999931720218, 0.3452994616207497591 ) ) ;
#9202=CARTESIAN_POINT ( 'NONE',  ( -62.86468353124999453, 13.95312499965860198, 1.500000000000002220 ) ) ;
#9206=CARTESIAN_POINT ( 'NONE',  ( -61.99999999999998579, 12.45312499965860020, 0.5015494609379544944 ) ) ;
#9207=CYLINDRICAL_SURFACE ( 'NONE', #10084, 0.9999999999999981126 ) ;
#9209=VERTEX_POINT ( 'NONE', #5047 ) ;
#9211=EDGE_CURVE ( 'NONE', #312, #5388, #1838, .T. ) ;
#9216=CARTESIAN_POINT ( 'NONE',  ( -60.99999999999998579, 15.47916666666666607, 2.077350269189628840 ) ) ;
#9217=CARTESIAN_POINT ( 'NONE',  ( -61.99999999999998579, 11.31250000000000000, 0.3452994616207497591 ) ) ;
#9219=CARTESIAN_POINT ( 'NONE',  ( -61.49999999999998579, 14.92708333265053611, 2.366025403784441927 ) ) ;
#9220=CARTESIAN_POINT ( 'NONE',  ( -62.99999999999998579, 13.84374999931720218, 1.500000000000001998 ) ) ;
#9222=CARTESIAN_POINT ( 'NONE',  ( -61.13531646874998415, 12.61979166632526805, 1.999225269531026417 ) ) ;
#9224=CARTESIAN_POINT ( 'NONE',  ( -61.99999999999998579, 9.031249999317202182, 0.5000000000000013323 ) ) ;
#9225=ORIENTED_EDGE ( 'NONE', *, *, #8822, .F. ) ;
#9230=CARTESIAN_POINT ( 'NONE',  ( -61.56765823437498142, 15.61979166632526628, 0.7511620957034663704 ) ) ;
#9232=CARTESIAN_POINT ( 'NONE',  ( -60.99999999999998579, 10.44791666598387003, 2.077350269189628840 ) ) ;
#9233=CYLINDRICAL_SURFACE ( 'NONE', #5461, 0.9999999999999981126 ) ;
#9234=CARTESIAN_POINT ( 'NONE',  ( -62.43234176562498305, 12.22395833299193413, 0.7511620957034662593 ) ) ;
#9235=EDGE_CURVE ( 'NONE', #5087, #10857, #2958, .T. ) ;
#9236=CARTESIAN_POINT ( 'NONE',  ( -62.86468353124999453, 15.51562499965860198, 1.500000000000002220 ) ) ;
#9237=CARTESIAN_POINT ( 'NONE',  ( -61.73205080756886076, 14.94866454968462932, 2.500000000000003109 ) ) ;
#9239=CARTESIAN_POINT ( 'NONE',  ( -61.99999999999998579, 8.828124999658601979, 2.498450539062049724 ) ) ;
#9240=CARTESIAN_POINT ( 'NONE',  ( -62.99999999999998579, 10.35416666666666785, 0.9226497308103756012 ) ) ;
#9244=CARTESIAN_POINT ( 'NONE',  ( -62.86468353124999453, 13.95312499965860198, 1.500000000000002220 ) ) ;
#9245=CARTESIAN_POINT ( 'NONE',  ( -61.99999999999998579, 10.76562499965860020, 2.498450539062049724 ) ) ;
#9246=CARTESIAN_POINT ( 'NONE',  ( -62.86468353124998032, 8.182291666325268054, 1.000774730468978024 ) ) ;
#9248=EDGE_LOOP ( 'NONE', ( #10796, #9753, #3591, #4024, #8628, #5568, #2304, #9833, #765, #329, #6505, #2877, #6954, #7695, #5416, #8634, #10722, #1716, #183, #3466, #2787, #2590, #5082, #3902, #2883, #4675, #172, #9303, #4420, #3918, #3652, #9549, #5025, #8355, #6484, #7503, #8119, #188, #3811, #1667, #807, #7970, #3311, #7106, #2425, #6611, #1704, #7369, #8304, #6715, #10737, #3543, #6931, #7587, #9886, #6191, #5064, #2760, #1543, #2133, #1541, #3907, #1832, #10616, #659, #3307, #3169, #1496 ) ) ;
#9249=CARTESIAN_POINT ( 'NONE',  ( -61.99999999999998579, 13.31250000000000000, 0.3452994616207497591 ) ) ;
#9250=CARTESIAN_POINT ( 'NONE',  ( -61.13531646874998415, 8.390624999658601979, 1.500000000000002220 ) ) ;
#9251=CARTESIAN_POINT ( 'NONE',  ( -62.99999999999998579, 12.09374999931720218, 1.500000000000001998 ) ) ;
#9252=CARTESIAN_POINT ( 'NONE',  ( -60.99999999999998579, 9.479166666666669627, 2.077350269189628840 ) ) ;
#9254=EDGE_CURVE ( 'NONE', #5880, #7919, #10893, .T. ) ;
#9255=CARTESIAN_POINT ( 'NONE',  ( -61.56765823437498852, 13.53645833299193413, 2.248837904296538515 ) ) ;
#9258=CARTESIAN_POINT ( 'NONE',  ( -61.56765823437498142, 13.43229166632526805, 0.7511620957034663704 ) ) ;
#9259=CARTESIAN_POINT ( 'NONE',  ( -62.26794919243111082, 12.64508544963257286, 2.500000000000003109 ) ) ;
#9262=FACE_OUTER_BOUND ( 'NONE', #7308, .T. ) ;
#9264=CARTESIAN_POINT ( 'NONE',  ( -61.99999999999998579, 16.00000000000000000, 2.500000000000000444 ) ) ;
#9265=VERTEX_POINT ( 'NONE', #8786 ) ;
#9266=CARTESIAN_POINT ( 'NONE',  ( -61.99999999999998579, 11.06250000000000000, 0.3452994616207497591 ) ) ;
#9269=CARTESIAN_POINT ( 'NONE',  ( -61.99999999999998579, 9.203124999658601979, 0.5015494609379544944 ) ) ;
#9270=CARTESIAN_POINT ( 'NONE',  ( -61.49999999999998579, 10.51041666598387003, 0.6339745962155628467 ) ) ;
#9273=CARTESIAN_POINT ( 'NONE',  ( -62.86468353124998032, 12.74479166632526805, 1.000774730468978246 ) ) ;
#9275=CARTESIAN_POINT ( 'NONE',  ( -62.26794919243111082, 12.89508544963257108, 2.500000000000003109 ) ) ;
#9278=ORIENTED_EDGE ( 'NONE', *, *, #801, .F. ) ;
#9280=CARTESIAN_POINT ( 'NONE',  ( -62.86468353124998032, 14.93229166632526983, 1.000774730468978246 ) ) ;
#9281=CARTESIAN_POINT ( 'NONE',  ( -61.99999999999998579, 14.40624999931720218, 2.500000000000002665 ) ) ;
#9283=CARTESIAN_POINT ( 'NONE',  ( -61.99999999999998579, 16.00000000000000000, 1.500000000000002220 ) ) ;
#9284=CARTESIAN_POINT ( 'NONE',  ( -62.86468353124999453, 13.28645833299193413, 1.999225269531025750 ) ) ;
#9285=CARTESIAN_POINT ( 'NONE',  ( -62.43234176562498305, 8.161458332991934128, 0.7511620957034662593 ) ) ;
#9286=CYLINDRICAL_SURFACE ( 'NONE', #4766, 0.9999999999999981126 ) ;
#9287=DIRECTION ( 'NONE',  ( -0.000000000000000000, -1.000000000000000000, -0.000000000000000000 ) ) ;
#9288=CARTESIAN_POINT ( 'NONE',  ( -61.13531646874998415, 9.140624999658601979, 1.500000000000002220 ) ) ;
#9289=CARTESIAN_POINT ( 'NONE',  ( -61.99999999999998579, 10.65624999931720218, 2.500000000000002665 ) ) ;
#9290=ORIENTED_EDGE ( 'NONE', *, *, #3250, .F. ) ;
#9291=AXIS2_PLACEMENT_3D ( 'NONE', #9552, #1109, #7780 ) ;
#9292=DIRECTION ( 'NONE',  ( -0.000000000000000000, 1.000000000000000000, -0.000000000000000000 ) ) ;
#9294=EDGE_CURVE ( 'NONE', #9906, #8873, #8486, .T. ) ;
#9296=CARTESIAN_POINT ( 'NONE',  ( -61.13531646874998415, 11.30729166632526805, 1.999225269531026417 ) ) ;
#9297=CARTESIAN_POINT ( 'NONE',  ( -62.86468353124999453, 15.01562499965860020, 1.500000000000002220 ) ) ;
#9298=DIRECTION ( 'NONE',  ( -0.8660254037844418162, -0.4999999999999947264, 0.000000000000000000 ) ) ;
#9300=CARTESIAN_POINT ( 'NONE',  ( -61.49999999999998579, 14.95833333333333393, 2.366025403784441927 ) ) ;
#9301=CARTESIAN_POINT ( 'NONE',  ( -62.86468353124999453, 9.036458332991935904, 1.999225269531025750 ) ) ;
#9302=CARTESIAN_POINT ( 'NONE',  ( -62.99999999999998579, 12.86458333265053788, 2.077350269189627952 ) ) ;
#9303=ORIENTED_EDGE ( 'NONE', *, *, #2766, .T. ) ;
#9304=CARTESIAN_POINT ( 'NONE',  ( -62.43234176562499016, 14.24479166632526983, 2.248837904296538071 ) ) ;
#9305=CARTESIAN_POINT ( 'NONE',  ( -61.99999999999998579, 16.00000000000000000, 1.500000000000002220 ) ) ;
#9308=CARTESIAN_POINT ( 'NONE',  ( -61.99999999999998579, 13.20312499965860198, 0.5015494609379544944 ) ) ;
#9309=CARTESIAN_POINT ( 'NONE',  ( -61.99999999999998579, 12.65624999931720396, 2.500000000000002665 ) ) ;
#9313=CARTESIAN_POINT ( 'NONE',  ( -62.26794919243111082, 12.32366454968463110, 0.5000000000000013323 ) ) ;
#9314=EDGE_CURVE ( 'NONE', #35, #3037, #1023, .T. ) ;
#9316=ORIENTED_EDGE ( 'NONE', *, *, #10276, .F. ) ;
#9317=CARTESIAN_POINT ( 'NONE',  ( -61.13531646874998415, 8.890624999658601979, 1.500000000000002220 ) ) ;
#9318=CARTESIAN_POINT ( 'NONE',  ( -62.49999999999998579, 15.91666666666666607, 2.366025403784441483 ) ) ;
#9320=CARTESIAN_POINT ( 'NONE',  ( -62.86468353124998032, 13.74479166632526805, 1.000774730468978246 ) ) ;
#9321=CARTESIAN_POINT ( 'NONE',  ( -60.99999999999998579, 8.218749999317202182, 1.500000000000002220 ) ) ;
#9325=FACE_OUTER_BOUND ( 'NONE', #8066, .T. ) ;
#9326=CARTESIAN_POINT ( 'NONE',  ( -62.43234176562499016, 15.74479166632526628, 2.248837904296538071 ) ) ;
#9327=CARTESIAN_POINT ( 'NONE',  ( -61.99999999999998579, 16.15624999931720041, 2.500000000000002665 ) ) ;
#9329=( BOUNDED_CURVE ( )  B_SPLINE_CURVE ( 2, ( #5213, #4375, #3164, #6569, #2282, #6512, #10830, #8959, #6404 ),
 .UNSPECIFIED., .F., .T. ) 
 B_SPLINE_CURVE_WITH_KNOTS ( ( 3, 2, 2, 2, 3 ),
 ( 0.9453125000000000000, 0.9479166666666666297, 0.9531250000000000000, 0.9583333333333333703, 0.9609375000000000000 ),
 .UNSPECIFIED. ) 
 CURVE ( )  GEOMETRIC_REPRESENTATION_ITEM ( )  RATIONAL_B_SPLINE_CURVE ( ( 0.9330127018922194093, 0.9330127018922194093, 1.000000000000000000, 0.8660254037844387076, 1.000000000000000000, 0.8660254037844387076, 1.000000000000000000, 0.9330127018922194093, 0.9330127018922194093 ) ) 
 REPRESENTATION_ITEM ( '' )  );
#9330=DIRECTION ( 'NONE',  ( 0.000000000000000000, 0.000000000000000000, -1.000000000000000000 ) ) ;
#9331=CARTESIAN_POINT ( 'NONE',  ( -61.99999999999999289, 13.20312499965860198, 0.5015494609379544944 ) ) ;
#9332=CARTESIAN_POINT ( 'NONE',  ( -61.13531646874998415, 8.348958332991935904, 1.000774730468978468 ) ) ;
#9333=CYLINDRICAL_SURFACE ( 'NONE', #7790, 0.9999999999999981126 ) ;
#9335=CARTESIAN_POINT ( 'NONE',  ( -62.43234176562499016, 9.307291666325268054, 2.248837904296538071 ) ) ;
#9336=CARTESIAN_POINT ( 'NONE',  ( -61.99999999999998579, 14.18750000000000000, 2.500000000000002665 ) ) ;
#9337=VERTEX_POINT ( 'NONE', #9726 ) ;
#9341=CARTESIAN_POINT ( 'NONE',  ( -61.99999999999999289, 15.64062499965860198, 0.5015494609379544944 ) ) ;
#9342=CARTESIAN_POINT ( 'NONE',  ( -61.99999999999998579, 11.51562499965860020, 2.498450539062049724 ) ) ;
#9344=CARTESIAN_POINT ( 'NONE',  ( -62.86468353124999453, 15.28645833299193413, 1.999225269531025750 ) ) ;
#9346=ORIENTED_EDGE ( 'NONE', *, *, #2419, .F. ) ;
#9347=CARTESIAN_POINT ( 'NONE',  ( -62.99999999999998579, 15.64583333333333393, 2.077350269189627952 ) ) ;
#9348=CARTESIAN_POINT ( 'NONE',  ( -62.86468353124998032, 8.494791666325268054, 1.000774730468978024 ) ) ;
#9349=CARTESIAN_POINT ( 'NONE',  ( -60.99999999999998579, 12.71874999931720396, 1.500000000000002220 ) ) ;
#9353=CARTESIAN_POINT ( 'NONE',  ( -62.86468353124999453, 12.20312499965860198, 1.500000000000002220 ) ) ;
#9354=CARTESIAN_POINT ( 'NONE',  ( -61.99999999999998579, 15.68749999999999645, 2.500000000000002665 ) ) ;
#9357=CARTESIAN_POINT ( 'NONE',  ( -61.99999999999998579, 12.82812499965860198, 2.498450539062049724 ) ) ;
#9358=CARTESIAN_POINT ( 'NONE',  ( -61.99999999999998579, 11.40624999931720218, 2.500000000000002665 ) ) ;
#9360=MECHANICAL_DESIGN_GEOMETRIC_PRESENTATION_REPRESENTATION('',(#8477),#3686);
#9361=CARTESIAN_POINT ( 'NONE',  ( -61.49999999999998579, 9.677083332650534331, 2.366025403784441927 ) ) ;
#9364=VECTOR ( 'NONE', #10817, 1000.000000000000000 ) ;
#9365=ORIENTED_EDGE ( 'NONE', *, *, #3790, .F. ) ;
#9366=CARTESIAN_POINT ( 'NONE',  ( -61.99999999999998579, 14.03124999931720218, 0.5000000000000013323 ) ) ;
#9367=CARTESIAN_POINT ( 'NONE',  ( -61.13531646874998415, 11.57812499965860198, 1.500000000000002220 ) ) ;
#9369=ORIENTED_EDGE ( 'NONE', *, *, #6789, .F. ) ;
#9370=VECTOR ( 'NONE', #4144, 1000.000000000000000 ) ;
#9371=CARTESIAN_POINT ( 'NONE',  ( -61.99999999999998579, 9.328124999658600203, 2.498450539062049724 ) ) ;
#9375=CARTESIAN_POINT ( 'NONE',  ( -62.86468353124998742, 12.53645833299193590, 1.999225269531025972 ) ) ;
#9376=CARTESIAN_POINT ( 'NONE',  ( -61.49999999999998579, 13.29166666666666607, 0.6339745962155628467 ) ) ;
#9379=ADVANCED_FACE ( 'NONE', ( #1167 ), #4546, .T. ) ;
#9381=CARTESIAN_POINT ( 'NONE',  ( -62.86468353124998032, 15.43229166632526805, 1.000774730468978246 ) ) ;
#9386=CARTESIAN_POINT ( 'NONE',  ( -62.86468353124999453, 13.51562499965860020, 1.500000000000002220 ) ) ;
#9387=CARTESIAN_POINT ( 'NONE',  ( -61.13531646874998415, 9.098958332991934128, 1.000774730468978468 ) ) ;
#9390=CARTESIAN_POINT ( 'NONE',  ( -61.13531646874998415, 8.661458332991935904, 1.000774730468978468 ) ) ;
#9391=CARTESIAN_POINT ( 'NONE',  ( -60.99999999999998579, 15.69791666598386648, 2.077350269189628840 ) ) ;
#9394=CARTESIAN_POINT ( 'NONE',  ( -61.73205080756886076, 11.27008544963257286, 0.5000000000000044409 ) ) ;
#9395=VECTOR ( 'NONE', #6941, 1000.000000000000000 ) ;
#9396=( BOUNDED_CURVE ( )  B_SPLINE_CURVE ( 2, ( #7214, #2163, #317, #5596, #10421 ),
 .UNSPECIFIED., .F., .F. ) 
 B_SPLINE_CURVE_WITH_KNOTS ( ( 3, 2, 3 ),
 ( 0.9921875000000000000, 0.9947916666666666297, 1.000000000000000000 ),
 .UNSPECIFIED. ) 
 CURVE ( )  GEOMETRIC_REPRESENTATION_ITEM ( )  RATIONAL_B_SPLINE_CURVE ( ( 0.9330127018922194093, 0.9330127018922194093, 1.000000000000000000, 0.8660254037844387076, 1.000000000000000000 ) ) 
 REPRESENTATION_ITEM ( '' )  );
#9397=CARTESIAN_POINT ( 'NONE',  ( -61.13531646874997705, 15.30729166632526983, 1.999225269531026417 ) ) ;
#9398=CARTESIAN_POINT ( 'NONE',  ( -61.99999999999998579, 10.64062499965860376, 0.5015494609379544944 ) ) ;
#9399=CARTESIAN_POINT ( 'NONE',  ( -61.13531646874997705, 8.807291666325268054, 1.999225269531026417 ) ) ;
#9400=CARTESIAN_POINT ( 'NONE',  ( -61.73205080756886076, 9.770085449632574637, 0.5000000000000044409 ) ) ;
#9402=CARTESIAN_POINT ( 'NONE',  ( -61.49999999999998579, 15.70833333333333037, 2.366025403784441927 ) ) ;
#9403=CARTESIAN_POINT ( 'NONE',  ( -62.43234176562498305, 8.473958332991934128, 0.7511620957034662593 ) ) ;
#9405=CARTESIAN_POINT ( 'NONE',  ( -61.49999999999998579, 13.42708333265053433, 2.366025403784441927 ) ) ;
#9406=CARTESIAN_POINT ( 'NONE',  ( -61.99999999999998579, 14.93749999999999822, 2.500000000000002665 ) ) ;
#9407=ORIENTED_EDGE ( 'NONE', *, *, #4221, .F. ) ;
#9408=CARTESIAN_POINT ( 'NONE',  ( -61.49999999999998579, 9.791666666666667851, 0.6339745962155628467 ) ) ;
#9410=CARTESIAN_POINT ( 'NONE',  ( -62.43234176562499016, 11.49479166632526805, 2.248837904296538071 ) ) ;
#9414=CARTESIAN_POINT ( 'NONE',  ( -61.99999999999998579, 15.43749999999999822, 2.500000000000002665 ) ) ;
#9415=CARTESIAN_POINT ( 'NONE',  ( -61.13531646874998415, 12.61979166632526805, 1.999225269531026417 ) ) ;
#9416=CARTESIAN_POINT ( 'NONE',  ( -61.99999999999998579, 12.06250000000000000, 0.5000000000000013323 ) ) ;
#9417=CARTESIAN_POINT ( 'NONE',  ( -61.99999999999998579, 9.281249999317200405, 0.3452994616207497591 ) ) ;
#9419=CARTESIAN_POINT ( 'NONE',  ( -61.73205080756886076, 13.94866454968462932, 2.500000000000003109 ) ) ;
#9421=CYLINDRICAL_SURFACE ( 'NONE', #1959, 0.9999999999999981126 ) ;
#9422=CARTESIAN_POINT ( 'NONE',  ( -62.86468353124998032, 11.93229166632526628, 1.000774730468978246 ) ) ;
#9425=ORIENTED_EDGE ( 'NONE', *, *, #3705, .T. ) ;
#9427=CARTESIAN_POINT ( 'NONE',  ( -62.43234176562499016, 8.807291666325268054, 2.248837904296538071 ) ) ;
#9428=CARTESIAN_POINT ( 'NONE',  ( -62.49999999999998579, 15.83333333333333037, 0.6339745962155627357 ) ) ;
#9429=CARTESIAN_POINT ( 'NONE',  ( -61.56765823437498852, 12.84895833299193413, 2.248837904296538515 ) ) ;
#9430=CARTESIAN_POINT ( 'NONE',  ( -60.99999999999998579, 13.22916666666666607, 2.077350269189628840 ) ) ;
#9433=LINE ( 'NONE', #100, #3197 ) ;
#9434=ORIENTED_EDGE ( 'NONE', *, *, #3149, .T. ) ;
#9435=CARTESIAN_POINT ( 'NONE',  ( -60.99999999999998579, 13.19791666598387003, 2.077350269189628840 ) ) ;
#9436=CARTESIAN_POINT ( 'NONE',  ( -62.86468353124998032, 15.18229166632526805, 1.000774730468978246 ) ) ;
#9437=CYLINDRICAL_SURFACE ( 'NONE', #2545, 0.9999999999999981126 ) ;
#9438=DIRECTION ( 'NONE',  ( 0.000000000000000000, 0.000000000000000000, 1.000000000000000000 ) ) ;
#9440=CIRCLE ( 'NONE', #8570, 2.500000000000002220 ) ;
#9441=CARTESIAN_POINT ( 'NONE',  ( -61.13531646874998415, 14.14062499965860198, 1.500000000000002220 ) ) ;
#9443=CARTESIAN_POINT ( 'NONE',  ( -61.13531646874998415, 9.307291666325268054, 1.999225269531026417 ) ) ;
#9446=CARTESIAN_POINT ( 'NONE',  ( -61.99999999999998579, 8.953124999658601979, 0.5015494609379544944 ) ) ;
#9447=FACE_OUTER_BOUND ( 'NONE', #3279, .T. ) ;
#9448=ORIENTED_EDGE ( 'NONE', *, *, #5434, .F. ) ;
#9450=CARTESIAN_POINT ( 'NONE',  ( -61.99999999999998579, 11.31250000000000000, 0.5000000000000013323 ) ) ;
#9451=AXIS2_PLACEMENT_3D ( 'NONE', #8239, #1455, #2288 ) ;
#9452=CARTESIAN_POINT ( 'NONE',  ( -62.43234176562498305, 15.91145833299193590, 0.7511620957034662593 ) ) ;
#9453=CARTESIAN_POINT ( 'NONE',  ( -62.43234176562499016, 10.99479166632526805, 2.248837904296538071 ) ) ;
#9454=CARTESIAN_POINT ( 'NONE',  ( -61.13531646874998415, 8.328124999658601979, 1.500000000000002220 ) ) ;
#9456=CARTESIAN_POINT ( 'NONE',  ( -61.49999999999998579, 14.79166666666666607, 0.6339745962155628467 ) ) ;
#9457=CARTESIAN_POINT ( 'NONE',  ( -62.43234176562499016, 10.30729166632526983, 2.248837904296538071 ) ) ;
#9462=CARTESIAN_POINT ( 'NONE',  ( -62.49999999999998579, 13.80208333265053611, 0.6339745962155627357 ) ) ;
#9463=CARTESIAN_POINT ( 'NONE',  ( -62.49999999999998579, 14.58333333333333393, 0.6339745962155627357 ) ) ;
#9464=VERTEX_POINT ( 'NONE', #663 ) ;
#9466=( BOUNDED_CURVE ( )  B_SPLINE_CURVE ( 2, ( #6859, #10289, #7028, #10406, #2635, #2866, #7750, #5173, #6079 ),
 .UNSPECIFIED., .F., .T. ) 
 B_SPLINE_CURVE_WITH_KNOTS ( ( 3, 2, 2, 2, 3 ),
 ( 0.4453125000000000000, 0.4479166666666666852, 0.4531250000000000000, 0.4583333333333333148, 0.4609375000000000000 ),
 .UNSPECIFIED. ) 
 CURVE ( )  GEOMETRIC_REPRESENTATION_ITEM ( )  RATIONAL_B_SPLINE_CURVE ( ( 0.9330127018922194093, 0.9330127018922194093, 1.000000000000000000, 0.8660254037844387076, 1.000000000000000000, 0.8660254037844387076, 1.000000000000000000, 0.9330127018922194093, 0.9330127018922194093 ) ) 
 REPRESENTATION_ITEM ( '' )  );
#9467=CARTESIAN_POINT ( 'NONE',  ( -62.86468353124998032, 11.18229166632526983, 1.000774730468978024 ) ) ;
#9471=CARTESIAN_POINT ( 'NONE',  ( -60.99999999999998579, 10.52083333333333393, 0.9226497308103762673 ) ) ;
#9473=CARTESIAN_POINT ( 'NONE',  ( -61.99999999999998579, 14.20312499965860198, 0.5015494609379544944 ) ) ;
#9474=CARTESIAN_POINT ( 'NONE',  ( -61.73205080756886076, 11.05133545031537068, 0.5000000000000014433 ) ) ;
#9475=CARTESIAN_POINT ( 'NONE',  ( -60.99999999999998579, 9.218749999317203958, 1.500000000000002220 ) ) ;
#9477=CARTESIAN_POINT ( 'NONE',  ( -61.99999999999998579, 14.06250000000000000, 0.5000000000000013323 ) ) ;
#9478=CARTESIAN_POINT ( 'NONE',  ( -61.49999999999998579, 9.927083332650536107, 2.366025403784441927 ) ) ;
#9479=CARTESIAN_POINT ( 'NONE',  ( -62.86468353124998032, 10.68229166632526628, 1.000774730468978246 ) ) ;
#9481=ORIENTED_EDGE ( 'NONE', *, *, #10968, .T. ) ;
#9483=CARTESIAN_POINT ( 'NONE',  ( -62.43234176562498305, 8.973958332991934128, 0.7511620957034662593 ) ) ;
#9485=CARTESIAN_POINT ( 'NONE',  ( -61.99999999999998579, 14.32812499965860020, 2.498450539062049724 ) ) ;
#9486=CARTESIAN_POINT ( 'NONE',  ( -61.73205080756886076, 13.19866454968462932, 2.500000000000003109 ) ) ;
#9488=LINE ( 'NONE', #2773, #10461 ) ;
#9491=CARTESIAN_POINT ( 'NONE',  ( -61.49999999999998579, 12.79166666666666607, 0.6339745962155628467 ) ) ;
#9492=CARTESIAN_POINT ( 'NONE',  ( -62.99999999999998579, 8.875000000000001776, 1.500000000000001998 ) ) ;
#9494=LINE ( 'NONE', #8500, #4385 ) ;
#9496=CARTESIAN_POINT ( 'NONE',  ( -61.56765823437498142, 13.43229166632526805, 0.7511620957034663704 ) ) ;
#9497=CARTESIAN_POINT ( 'NONE',  ( -61.13531646874998415, 8.307291666325269830, 1.999225269531026417 ) ) ;
#9500=EDGE_CURVE ( 'NONE', #6298, #7493, #2178, .T. ) ;
#9501=CARTESIAN_POINT ( 'NONE',  ( -61.13531646874998415, 11.16145833299193413, 1.000774730468978468 ) ) ;
#9503=ORIENTED_EDGE ( 'NONE', *, *, #9667, .T. ) ;
#9506=CARTESIAN_POINT ( 'NONE',  ( -61.99999999999998579, 16.00000000000000000, 2.500000000000000444 ) ) ;
#9507=CARTESIAN_POINT ( 'NONE',  ( -62.86468353124998032, 12.93229166632526805, 1.000774730468978246 ) ) ;
#9508=CARTESIAN_POINT ( 'NONE',  ( -61.13531646874997705, 8.348958332991934128, 1.000774730468978468 ) ) ;
#9511=ORIENTED_EDGE ( 'NONE', *, *, #1348, .F. ) ;
#9512=CARTESIAN_POINT ( 'NONE',  ( -62.49999999999998579, 15.16666666666666607, 2.366025403784441483 ) ) ;
#9513=CARTESIAN_POINT ( 'NONE',  ( -61.56765823437498852, 10.34895833299193413, 2.248837904296538515 ) ) ;
#9514=CARTESIAN_POINT ( 'NONE',  ( -61.13531646874998415, 15.55729166632526628, 1.999225269531026417 ) ) ;
#9515=CARTESIAN_POINT ( 'NONE',  ( -62.99999999999998579, 13.07291666598387003, 0.9226497308103756012 ) ) ;
#9518=ADVANCED_FACE ( 'NONE', ( #8957 ), #9949, .F. ) ;
#9519=CARTESIAN_POINT ( 'NONE',  ( -60.99999999999998579, 9.729166666666667851, 2.077350269189628840 ) ) ;
#9520=CARTESIAN_POINT ( 'NONE',  ( -61.13531646874997705, 11.05729166632526805, 1.999225269531026417 ) ) ;
#9521=EDGE_CURVE ( 'NONE', #2251, #8495, #5583, .T. ) ;
#9524=CARTESIAN_POINT ( 'NONE',  ( -61.06765823437498852, 16.17968749948790119, 1.500000000000002220 ) ) ;
#9526=CARTESIAN_POINT ( 'NONE',  ( -62.99999999999998579, 10.89583333333333393, 2.077350269189627952 ) ) ;
#9527=DIRECTION ( 'NONE',  ( -0.000000000000000000, -1.000000000000000000, -0.000000000000000000 ) ) ;
#9528=CARTESIAN_POINT ( 'NONE',  ( -61.13531646874998415, 13.64062499965860198, 1.500000000000002220 ) ) ;
#9529=CARTESIAN_POINT ( 'NONE',  ( -61.99999999999998579, 10.18750000000000000, 2.500000000000002665 ) ) ;
#9530=CARTESIAN_POINT ( 'NONE',  ( -62.49999999999998579, 9.635416665983870033, 2.366025403784441483 ) ) ;
#9532=( BOUNDED_CURVE ( )  B_SPLINE_CURVE ( 2, ( #8741, #288, #6299, #7069, #1358, #2134, #4724, #6240, #1240 ),
 .UNSPECIFIED., .F., .T. ) 
 B_SPLINE_CURVE_WITH_KNOTS ( ( 3, 2, 2, 2, 3 ),
 ( 0.2265625000000000000, 0.2291666666666666574, 0.2343750000000000000, 0.2395833333333333426, 0.2421874999999999722 ),
 .UNSPECIFIED. ) 
 CURVE ( )  GEOMETRIC_REPRESENTATION_ITEM ( )  RATIONAL_B_SPLINE_CURVE ( ( 0.9330127018922194093, 0.9330127018922194093, 1.000000000000000000, 0.8660254037844387076, 1.000000000000000000, 0.8660254037844387076, 1.000000000000000000, 0.9330127018922200755, 0.9330127018922194093 ) ) 
 REPRESENTATION_ITEM ( '' )  );
#9533=CARTESIAN_POINT ( 'NONE',  ( -61.73205080756886076, 13.44866454968462932, 2.500000000000003109 ) ) ;
#9535=CARTESIAN_POINT ( 'NONE',  ( -62.86468353124998742, 11.72395833299193413, 1.999225269531025972 ) ) ;
#9537=EDGE_LOOP ( 'NONE', ( #2894, #2438, #1787, #9503 ) ) ;
#9539=CARTESIAN_POINT ( 'NONE',  ( -61.99999999999998579, 10.57812499965860198, 2.498450539062049724 ) ) ;
#9541=ADVANCED_FACE ( 'NONE', ( #4930 ), #3212, .T. ) ;
#9542=CARTESIAN_POINT ( 'NONE',  ( -61.13531646874998415, 15.16145833299193590, 1.000774730468978468 ) ) ;
#9543=CARTESIAN_POINT ( 'NONE',  ( -61.49999999999998579, 8.927083332650536107, 2.366025403784441927 ) ) ;
#9547=ADVANCED_FACE ( 'NONE', ( #4716 ), #6619, .T. ) ;
#9549=ORIENTED_EDGE ( 'NONE', *, *, #4412, .T. ) ;
#9550=CARTESIAN_POINT ( 'NONE',  ( -61.99999999999998579, 16.00000000000000000, 0.5000000000000041078 ) ) ;
#9551=CARTESIAN_POINT ( 'NONE',  ( -60.99999999999998579, 9.000000000000001776, 1.500000000000002220 ) ) ;
#9552=CARTESIAN_POINT ( 'NONE',  ( -61.99999999999998579, 16.00000000000000000, 1.500000000000002220 ) ) ;
#9553=CARTESIAN_POINT ( 'NONE',  ( -60.99999999999998579, 12.00000000000000000, 1.500000000000002220 ) ) ;
#9555=CARTESIAN_POINT ( 'NONE',  ( -61.56765823437498852, 13.84895833299193413, 2.248837904296538515 ) ) ;
#9557=CARTESIAN_POINT ( 'NONE',  ( -61.56765823437498142, 9.119791666325268054, 0.7511620957034663704 ) ) ;
#9558=CARTESIAN_POINT ( 'NONE',  ( -61.99999999999998579, 16.00000000000000000, 0.5000000000000041078 ) ) ;
#9560=CARTESIAN_POINT ( 'NONE',  ( -61.13531646874998415, 10.39062499965860198, 1.500000000000002220 ) ) ;
#9562=CARTESIAN_POINT ( 'NONE',  ( -61.99999999999998579, 16.00000000000000000, 1.500000000000002220 ) ) ;
#9564=CARTESIAN_POINT ( 'NONE',  ( -62.49999999999998579, 14.33333333333333393, 0.6339745962155627357 ) ) ;
#9565=CARTESIAN_POINT ( 'NONE',  ( -60.99999999999998579, 11.21874999931720218, 1.500000000000002220 ) ) ;
#9568=EDGE_CURVE ( 'NONE', #10687, #1239, #5864, .T. ) ;
#9569=CARTESIAN_POINT ( 'NONE',  ( -62.86468353124999453, 12.45312499965860198, 1.500000000000002220 ) ) ;
#9570=CARTESIAN_POINT ( 'NONE',  ( -61.56765823437498142, 9.369791666325268054, 0.7511620957034663704 ) ) ;
#9572=CARTESIAN_POINT ( 'NONE',  ( -61.99999999999998579, 15.81250000000000000, 0.3452994616207497591 ) ) ;
#9573=CARTESIAN_POINT ( 'NONE',  ( -61.56765823437498852, 10.59895833299193413, 2.248837904296538515 ) ) ;
#9574=CARTESIAN_POINT ( 'NONE',  ( -62.86468353124998742, 15.22395833299193590, 1.999225269531025972 ) ) ;
#9576=CARTESIAN_POINT ( 'NONE',  ( -62.49999999999998579, 14.55208333265053611, 0.6339745962155627357 ) ) ;
#9578=ORIENTED_EDGE ( 'NONE', *, *, #5180, .T. ) ;
#9581=CARTESIAN_POINT ( 'NONE',  ( -62.86468353124999453, 11.70312499965860198, 1.500000000000002220 ) ) ;
#9582=CARTESIAN_POINT ( 'NONE',  ( -62.86468353124999453, 8.703124999658601979, 1.500000000000002220 ) ) ;
#9585=ORIENTED_EDGE ( 'NONE', *, *, #4800, .T. ) ;
#9586=CARTESIAN_POINT ( 'NONE',  ( -61.49999999999998579, 11.79166666666666785, 0.6339745962155628467 ) ) ;
#9587=FACE_OUTER_BOUND ( 'NONE', #71, .T. ) ;
#9588=CARTESIAN_POINT ( 'NONE',  ( -61.56765823437498142, 14.43229166632526983, 0.7511620957034663704 ) ) ;
#9589=FACE_OUTER_BOUND ( 'NONE', #2244, .T. ) ;
#9590=CARTESIAN_POINT ( 'NONE',  ( -60.99999999999998579, 10.44791666598387003, 2.077350269189628840 ) ) ;
#9592=EDGE_CURVE ( 'NONE', #869, #3127, #492, .T. ) ;
#9595=CARTESIAN_POINT ( 'NONE',  ( -61.13531646874998415, 10.82812499965860020, 1.500000000000002220 ) ) ;
#9598=CARTESIAN_POINT ( 'NONE',  ( -62.86468353124999453, 10.26562499965860198, 1.500000000000002220 ) ) ;
#9600=EDGE_CURVE ( 'NONE', #947, #8873, #95, .T. ) ;
#9601=CARTESIAN_POINT ( 'NONE',  ( -61.13531646874998415, 14.61979166632526805, 1.999225269531026417 ) ) ;
#9604=CARTESIAN_POINT ( 'NONE',  ( -62.49999999999998579, 9.416666666666666075, 2.366025403784441483 ) ) ;
#9607=CARTESIAN_POINT ( 'NONE',  ( -61.99999999999998579, 8.812500000000000000, 0.5000000000000013323 ) ) ;
#9608=CARTESIAN_POINT ( 'NONE',  ( -62.99999999999998579, 8.625000000000000000, 1.500000000000001998 ) ) ;
#9609=DIRECTION ( 'NONE',  ( -0.000000000000000000, -1.000000000000000000, -0.000000000000000000 ) ) ;
#9610=CARTESIAN_POINT ( 'NONE',  ( -61.06765823437498852, 16.03906249982930277, 1.500000000000002220 ) ) ;
#9611=CARTESIAN_POINT ( 'NONE',  ( -60.99999999999998579, 10.73958333265053611, 0.9226497308103762673 ) ) ;
#9612=CARTESIAN_POINT ( 'NONE',  ( -62.86468353124998032, 13.49479166632526805, 1.000774730468978024 ) ) ;
#9613=CARTESIAN_POINT ( 'NONE',  ( -61.13531646874998415, 10.09895833299193413, 1.000774730468978468 ) ) ;
#9614=UNCERTAINTY_MEASURE_WITH_UNIT (LENGTH_MEASURE( 1.000000000000000082E-05 ), #1804, 'distance_accuracy_value', 'NONE');
#9615=EDGE_CURVE ( 'NONE', #6298, #3002, #3270, .T. ) ;
#9617=CARTESIAN_POINT ( 'NONE',  ( -62.99999999999998579, 9.604166666666667851, 0.9226497308103756012 ) ) ;
#9619=CARTESIAN_POINT ( 'NONE',  ( -61.99999999999998579, 10.07812499965860198, 2.498450539062049724 ) ) ;
#9620=CARTESIAN_POINT ( 'NONE',  ( -61.99999999999998579, 16.00000000000000000, 0.5000000000000041078 ) ) ;
#9625=VECTOR ( 'NONE', #3117, 999.9999999999998863 ) ;
#9626=DIRECTION ( 'NONE',  ( -0.000000000000000000, -1.000000000000000000, -0.000000000000000000 ) ) ;
#9627=CARTESIAN_POINT ( 'NONE',  ( -61.13531646874998415, 13.07812499965860198, 1.500000000000002220 ) ) ;
#9628=CARTESIAN_POINT ( 'NONE',  ( -62.43234176562498305, 9.411458332991935904, 0.7511620957034662593 ) ) ;
#9631=CARTESIAN_POINT ( 'NONE',  ( -61.99999999999998579, 8.406249999317203958, 2.500000000000003109 ) ) ;
#9632=CARTESIAN_POINT ( 'NONE',  ( -62.86468353124999453, 10.28645833299193413, 1.999225269531025750 ) ) ;
#9634=CARTESIAN_POINT ( 'NONE',  ( -62.43234176562498305, 15.91145833299193590, 0.7511620957034662593 ) ) ;
#9635=CARTESIAN_POINT ( 'NONE',  ( -62.49999999999998579, 14.13541666598387003, 2.366025403784441483 ) ) ;
#9638=AXIS2_PLACEMENT_3D ( 'NONE', #4395, #9640, #1014 ) ;
#9640=DIRECTION ( 'NONE',  ( -0.000000000000000000, -1.000000000000000000, -0.000000000000000000 ) ) ;
#9641=ORIENTED_EDGE ( 'NONE', *, *, #6084, .T. ) ;
#9643=CARTESIAN_POINT ( 'NONE',  ( -61.99999999999999289, 12.26562499965860198, 2.498450539062049724 ) ) ;
#9644=CARTESIAN_POINT ( 'NONE',  ( -61.99999999999998579, 11.90624999931720041, 2.500000000000002665 ) ) ;
#9645=LINE ( 'NONE', #8813, #7310 ) ;
#9646=ORIENTED_EDGE ( 'NONE', *, *, #4359, .F. ) ;
#9647=CARTESIAN_POINT ( 'NONE',  ( -62.99999999999998579, 12.64583333333333393, 2.077350269189627952 ) ) ;
#9650=CARTESIAN_POINT ( 'NONE',  ( -61.13531646874998415, 13.91145833299193413, 1.000774730468978468 ) ) ;
#9651=CARTESIAN_POINT ( 'NONE',  ( -61.99999999999998579, 14.93749999999999822, 2.500000000000002665 ) ) ;
#9652=CARTESIAN_POINT ( 'NONE',  ( -61.49999999999998579, 10.92708333265053611, 2.366025403784441927 ) ) ;
#9654=CARTESIAN_POINT ( 'NONE',  ( -60.99999999999998579, 14.00000000000000000, 1.500000000000002220 ) ) ;
#9655=CARTESIAN_POINT ( 'NONE',  ( -62.99999999999998579, 15.36458333265053611, 2.077350269189627952 ) ) ;
#9656=CARTESIAN_POINT ( 'NONE',  ( -62.43234176562498305, 12.16145833299193413, 0.7511620957034662593 ) ) ;
#9659=CARTESIAN_POINT ( 'NONE',  ( -62.86468353124998742, 9.786458332991934128, 1.999225269531025972 ) ) ;
#9660=CARTESIAN_POINT ( 'NONE',  ( -61.99999999999998579, 15.65624999931720218, 2.500000000000002665 ) ) ;
#9661=CARTESIAN_POINT ( 'NONE',  ( -62.43234176562499016, 14.55729166632526983, 2.248837904296538071 ) ) ;
#9663=EDGE_CURVE ( 'NONE', #8255, #9464, #3113, .T. ) ;
#9664=CARTESIAN_POINT ( 'NONE',  ( -61.99999999999998579, 16.00000000000000000, 1.500000000000002220 ) ) ;
#9665=EDGE_LOOP ( 'NONE', ( #5132, #5633 ) ) ;
#9666=CARTESIAN_POINT ( 'NONE',  ( -60.99999999999998579, 8.770833333333333925, 0.9226497308103762673 ) ) ;
#9667=EDGE_CURVE ( 'NONE', #6433, #10637, #2456, .T. ) ;
#9668=CARTESIAN_POINT ( 'NONE',  ( -62.99999999999998579, 8.645833333333333925, 2.077350269189627952 ) ) ;
#9672=CARTESIAN_POINT ( 'NONE',  ( -61.56765823437498852, 14.84895833299193413, 2.248837904296538515 ) ) ;
#9673=CARTESIAN_POINT ( 'NONE',  ( -62.43234176562498305, 9.661458332991934128, 0.7511620957034662593 ) ) ;
#9676=CARTESIAN_POINT ( 'NONE',  ( -61.99999999999998579, 10.82812499965860198, 2.498450539062049724 ) ) ;
#9677=CARTESIAN_POINT ( 'NONE',  ( -62.26794919243111082, 13.67633545031537068, 2.500000000000003109 ) ) ;
#9678=ORIENTED_EDGE ( 'NONE', *, *, #175, .F. ) ;
#9680=CARTESIAN_POINT ( 'NONE',  ( -62.99999999999998579, 9.125000000000000000, 1.500000000000001998 ) ) ;
#9682=CARTESIAN_POINT ( 'NONE',  ( -62.86468353124998032, 12.43229166632526628, 1.000774730468978246 ) ) ;
#9683=CARTESIAN_POINT ( 'NONE',  ( -61.99999999999999289, 10.64062499965860198, 0.5015494609379544944 ) ) ;
#9687=CARTESIAN_POINT ( 'NONE',  ( -61.13531646874997705, 10.66145833299193413, 1.000774730468978468 ) ) ;
#9688=PRODUCT_CONTEXT ( 'NONE', #4401, 'mechanical' ) ;
#9689=CARTESIAN_POINT ( 'NONE',  ( -62.86468353124998032, 15.68229166632526628, 1.000774730468978246 ) ) ;
#9690=CARTESIAN_POINT ( 'NONE',  ( -61.49999999999998579, 14.26041666598387003, 0.6339745962155628467 ) ) ;
#9691=DIRECTION ( 'NONE',  ( -0.000000000000000000, -1.000000000000000000, -0.000000000000000000 ) ) ;
#9697=CARTESIAN_POINT ( 'NONE',  ( -61.99999999999999289, 12.89062499965860198, 0.5015494609379544944 ) ) ;
#9698=CARTESIAN_POINT ( 'NONE',  ( -61.99999999999998579, 8.140624999658601979, 0.5015494609379544944 ) ) ;
#9701=CARTESIAN_POINT ( 'NONE',  ( -61.49999999999998579, 12.79166666666666607, 0.6339745962155628467 ) ) ;
#9703=CARTESIAN_POINT ( 'NONE',  ( -62.86468353124998032, 14.74479166632526628, 1.000774730468978246 ) ) ;
#9704=( BOUNDED_CURVE ( )  B_SPLINE_CURVE ( 2, ( #5756, #6655, #3521, #8637, #4183, #4400, #3575, #5966, #9354 ),
 .UNSPECIFIED., .F., .F. ) 
 B_SPLINE_CURVE_WITH_KNOTS ( ( 3, 2, 2, 2, 3 ),
 ( 0.9453125000000000000, 0.9479166666666666297, 0.9531250000000000000, 0.9583333333333333703, 0.9609375000000000000 ),
 .UNSPECIFIED. ) 
 CURVE ( )  GEOMETRIC_REPRESENTATION_ITEM ( )  RATIONAL_B_SPLINE_CURVE ( ( 0.9330127018922194093, 0.9330127018922194093, 1.000000000000000000, 0.8660254037844387076, 1.000000000000000000, 0.8660254037844387076, 1.000000000000000000, 0.9330127018922194093, 0.9330127018922194093 ) ) 
 REPRESENTATION_ITEM ( '' )  );
#9706=CARTESIAN_POINT ( 'NONE',  ( -60.99999999999998579, 10.23958333265053788, 0.9226497308103762673 ) ) ;
#9710=CARTESIAN_POINT ( 'NONE',  ( -62.43234176562498305, 12.66145833299193413, 0.7511620957034662593 ) ) ;
#9711=ORIENTED_EDGE ( 'NONE', *, *, #4633, .T. ) ;
#9712=EDGE_CURVE ( 'NONE', #312, #8261, #5366, .T. ) ;
#9713=CARTESIAN_POINT ( 'NONE',  ( -61.13531646874998415, 9.890624999658601979, 1.500000000000002220 ) ) ;
#9715=CARTESIAN_POINT ( 'NONE',  ( -61.99999999999998579, 14.95312499965860198, 0.5015494609379544944 ) ) ;
#9716=CARTESIAN_POINT ( 'NONE',  ( -61.99999999999998579, 14.68750000000000000, 2.500000000000002665 ) ) ;
#9718=DIRECTION ( 'NONE',  ( -0.000000000000000000, -1.000000000000000000, -0.000000000000000000 ) ) ;
#9719=VECTOR ( 'NONE', #6548, 1000.000000000000000 ) ;
#9720=ORIENTED_EDGE ( 'NONE', *, *, #4423, .F. ) ;
#9721=CARTESIAN_POINT ( 'NONE',  ( -60.99999999999998579, 8.750000000000000000, 1.500000000000002220 ) ) ;
#9722=CARTESIAN_POINT ( 'NONE',  ( -62.99999999999998579, 8.895833333333333925, 2.077350269189627952 ) ) ;
#9723=DIRECTION ( 'NONE',  ( -0.000000000000000000, -1.000000000000000000, -0.000000000000000000 ) ) ;
#9724=CARTESIAN_POINT ( 'NONE',  ( -61.49999999999998579, 12.04166666666666607, 0.6339745962155628467 ) ) ;
#9725=ADVANCED_FACE ( 'NONE', ( #2886 ), #383, .T. ) ;
#9726=CARTESIAN_POINT ( 'NONE',  ( -61.99999999999998579, 9.187500000000000000, 2.500000000000002665 ) ) ;
#9727=CARTESIAN_POINT ( 'NONE',  ( -61.99999999999998579, 10.51562499965860198, 2.498450539062049724 ) ) ;
#9728=CARTESIAN_POINT ( 'NONE',  ( -62.43234176562498305, 10.47395833299193413, 0.7511620957034662593 ) ) ;
#9729=CARTESIAN_POINT ( 'NONE',  ( -62.26794919243111082, 12.07366454968463110, 0.5000000000000013323 ) ) ;
#9734=CARTESIAN_POINT ( 'NONE',  ( -62.99999999999998579, 9.145833333333333925, 2.077350269189627952 ) ) ;
#9737=CARTESIAN_POINT ( 'NONE',  ( -62.26794919243111082, 10.29241454900183328, 0.5000000000000013323 ) ) ;
#9738=CARTESIAN_POINT ( 'NONE',  ( -62.43234176562499016, 12.24479166632526805, 2.248837904296538071 ) ) ;
#9740=CARTESIAN_POINT ( 'NONE',  ( -61.99999999999999289, 10.51562499965860198, 2.498450539062049724 ) ) ;
#9741=CARTESIAN_POINT ( 'NONE',  ( -61.99999999999998579, 8.687500000000000000, 2.500000000000002665 ) ) ;
#9744=CARTESIAN_POINT ( 'NONE',  ( -61.99999999999999289, 11.57812499965860198, 2.498450539062049724 ) ) ;
#9747=CARTESIAN_POINT ( 'NONE',  ( -61.13531646874998415, 14.84895833299193413, 1.000774730468978468 ) ) ;
#9748=CARTESIAN_POINT ( 'NONE',  ( -61.49999999999998579, 15.26041666598387003, 0.6339745962155628467 ) ) ;
#9749=CARTESIAN_POINT ( 'NONE',  ( -60.99999999999998579, 14.71874999931720218, 1.500000000000002220 ) ) ;
#9751=CARTESIAN_POINT ( 'NONE',  ( -61.73205080756886076, 16.02008544963257464, 0.5000000000000014433 ) ) ;
#9753=ORIENTED_EDGE ( 'NONE', *, *, #1614, .T. ) ;
#9755=CARTESIAN_POINT ( 'NONE',  ( -62.43234176562499016, 12.24479166632526805, 2.248837904296538071 ) ) ;
#9756=CARTESIAN_POINT ( 'NONE',  ( -61.56765823437498142, 8.119791666325268054, 0.7511620957034663704 ) ) ;
#9757=CARTESIAN_POINT ( 'NONE',  ( -61.99999999999997868, 10.53124999931720573, 0.5000000000000013323 ) ) ;
#9758=EDGE_LOOP ( 'NONE', ( #6267, #9346, #6312, #3753 ) ) ;
#9759=CARTESIAN_POINT ( 'NONE',  ( -61.99999999999998579, 12.93750000000000178, 2.654700538379254571 ) ) ;
#9760=CARTESIAN_POINT ( 'NONE',  ( -60.99999999999998579, 9.020833333333333925, 0.9226497308103762673 ) ) ;
#9763=CARTESIAN_POINT ( 'NONE',  ( -61.99999999999998579, 16.00000000000000000, 1.500000000000002220 ) ) ;
#9764=CARTESIAN_POINT ( 'NONE',  ( -60.99999999999998579, 10.48958333265053611, 0.9226497308103762673 ) ) ;
#9766=( GEOMETRIC_REPRESENTATION_CONTEXT ( 3 ) GLOBAL_UNCERTAINTY_ASSIGNED_CONTEXT ( ( #10707 ) ) GLOBAL_UNIT_ASSIGNED_CONTEXT ( ( #8264, #5017, #7425 ) ) REPRESENTATION_CONTEXT ( 'NONE', 'WORKASPACE' ) );
#9768=FACE_OUTER_BOUND ( 'NONE', #2185, .T. ) ;
#9770=CARTESIAN_POINT ( 'NONE',  ( -62.86468353124999453, 13.20312499965860198, 1.500000000000002220 ) ) ;
#9772=CARTESIAN_POINT ( 'NONE',  ( -61.56765823437498852, 8.598958332991934128, 2.248837904296538515 ) ) ;
#9773=( BOUNDED_CURVE ( )  B_SPLINE_CURVE ( 2, ( #1986, #3763, #9478, #10306, #4415, #314, #5358, #202, #3701 ),
 .UNSPECIFIED., .F., .T. ) 
 B_SPLINE_CURVE_WITH_KNOTS ( ( 3, 2, 2, 2, 3 ),
 ( 0.2109375000000000000, 0.2135416666666666574, 0.2187500000000000000, 0.2239583333333333426, 0.2265625000000000000 ),
 .UNSPECIFIED. ) 
 CURVE ( )  GEOMETRIC_REPRESENTATION_ITEM ( )  RATIONAL_B_SPLINE_CURVE ( ( 0.9330127018922194093, 0.9330127018922194093, 1.000000000000000000, 0.8660254037844387076, 1.000000000000000000, 0.8660254037844387076, 1.000000000000000000, 0.9330127018922194093, 0.9330127018922194093 ) ) 
 REPRESENTATION_ITEM ( '' )  );
#9775=CARTESIAN_POINT ( 'NONE',  ( -62.86468353124998032, 10.49479166632526983, 1.000774730468978246 ) ) ;
#9777=CARTESIAN_POINT ( 'NONE',  ( -62.86468353124998032, 15.74479166632526805, 1.000774730468978246 ) ) ;
#9779=VERTEX_POINT ( 'NONE', #3537 ) ;
#9780=CYLINDRICAL_SURFACE ( 'NONE', #10469, 0.9999999999999981126 ) ;
#9781=EDGE_CURVE ( 'NONE', #5253, #4602, #9931, .T. ) ;
#9784=CARTESIAN_POINT ( 'NONE',  ( -62.99999999999998579, 9.145833333333333925, 2.077350269189627952 ) ) ;
#9786=CARTESIAN_POINT ( 'NONE',  ( -61.73205080756886076, 12.05133545031537068, 0.5000000000000014433 ) ) ;
#9787=CARTESIAN_POINT ( 'NONE',  ( -61.49999999999998579, 8.291666666666666075, 0.6339745962155628467 ) ) ;
#9788=CARTESIAN_POINT ( 'NONE',  ( -61.99999999999998579, 10.14062499965860198, 0.5015494609379544944 ) ) ;
#9789=CARTESIAN_POINT ( 'NONE',  ( -61.49999999999998579, 15.42708333265053611, 2.366025403784441927 ) ) ;
#9790=CARTESIAN_POINT ( 'NONE',  ( -62.43234176562499016, 12.05729166632526628, 2.248837904296538071 ) ) ;
#9792=ORIENTED_EDGE ( 'NONE', *, *, #10358, .T. ) ;
#9793=VECTOR ( 'NONE', #5587, 1000.000000000000000 ) ;
#9797=CARTESIAN_POINT ( 'NONE',  ( -62.99999999999998579, 10.32291666598387003, 0.9226497308103756012 ) ) ;
#9798=CARTESIAN_POINT ( 'NONE',  ( -61.56765823437498142, 14.11979166632526805, 0.7511620957034663704 ) ) ;
#9799=CARTESIAN_POINT ( 'NONE',  ( -61.13531646874998415, 10.07812499965860198, 1.500000000000002220 ) ) ;
#9801=EDGE_LOOP ( 'NONE', ( #3862, #9880, #3041, #1493 ) ) ;
#9803=CARTESIAN_POINT ( 'NONE',  ( -62.86468353124998032, 11.24479166632526805, 1.000774730468978024 ) ) ;
#9805=CARTESIAN_POINT ( 'NONE',  ( -60.99999999999998579, 13.98958333265053788, 0.9226497308103762673 ) ) ;
#9811=CARTESIAN_POINT ( 'NONE',  ( -61.13531646874997705, 13.09895833299193413, 1.000774730468978468 ) ) ;
#9812=CARTESIAN_POINT ( 'NONE',  ( -62.86468353124998742, 8.473958332991934128, 1.999225269531025972 ) ) ;
#9813=CARTESIAN_POINT ( 'NONE',  ( -62.49999999999998579, 8.416666666666666075, 2.366025403784441483 ) ) ;
#9814=VERTEX_POINT ( 'NONE', #7888 ) ;
#9815=CARTESIAN_POINT ( 'NONE',  ( -62.99999999999998579, 11.85416666666666607, 0.9226497308103756012 ) ) ;
#9820=AXIS2_PLACEMENT_3D ( 'NONE', #8469, #6755, #4909 ) ;
#9821=CARTESIAN_POINT ( 'NONE',  ( -62.99999999999998579, 10.07291666598387003, 0.9226497308103756012 ) ) ;
#9823=CARTESIAN_POINT ( 'NONE',  ( -62.26794919243111082, 13.42633545031536890, 2.500000000000003109 ) ) ;
#9825=CARTESIAN_POINT ( 'NONE',  ( -61.56765823437498142, 12.86979166632526805, 0.7511620957034663704 ) ) ;
#9827=VERTEX_POINT ( 'NONE', #10488 ) ;
#9828=CARTESIAN_POINT ( 'NONE',  ( -61.56765823437498142, 11.93229166632526805, 0.7511620957034663704 ) ) ;
#9829=CYLINDRICAL_SURFACE ( 'NONE', #7610, 0.9999999999999981126 ) ;
#9831=CARTESIAN_POINT ( 'NONE',  ( -61.99999999999998579, 15.32812499965860198, 2.498450539062049724 ) ) ;
#9833=ORIENTED_EDGE ( 'NONE', *, *, #3927, .T. ) ;
#9836=( BOUNDED_CURVE ( )  B_SPLINE_CURVE ( 2, ( #4328, #4273, #7683, #2618, #4445, #286, #7847, #5327, #232 ),
 .UNSPECIFIED., .F., .T. ) 
 B_SPLINE_CURVE_WITH_KNOTS ( ( 3, 2, 2, 2, 3 ),
 ( 0.5859375000000000000, 0.5885416666666666297, 0.5937500000000000000, 0.5989583333333333703, 0.6015625000000000000 ),
 .UNSPECIFIED. ) 
 CURVE ( )  GEOMETRIC_REPRESENTATION_ITEM ( )  RATIONAL_B_SPLINE_CURVE ( ( 0.9330127018922194093, 0.9330127018922194093, 1.000000000000000000, 0.8660254037844387076, 1.000000000000000000, 0.8660254037844387076, 1.000000000000000000, 0.9330127018922194093, 0.9330127018922194093 ) ) 
 REPRESENTATION_ITEM ( '' )  );
#9839=CARTESIAN_POINT ( 'NONE',  ( -61.99999999999998579, 9.531249999317202182, 0.5000000000000013323 ) ) ;
#9840=CARTESIAN_POINT ( 'NONE',  ( -60.99999999999998579, 9.520833333333333925, 0.9226497308103762673 ) ) ;
#9842=CYLINDRICAL_SURFACE ( 'NONE', #10963, 0.9999999999999981126 ) ;
#9845=CARTESIAN_POINT ( 'NONE',  ( -61.99999999999998579, 16.00000000000000000, 1.500000000000002220 ) ) ;
#9846=CARTESIAN_POINT ( 'NONE',  ( -62.43234176562498305, 12.47395833299193413, 0.7511620957034662593 ) ) ;
#9847=CARTESIAN_POINT ( 'NONE',  ( -62.26794919243111082, 12.04241454900183328, 0.5000000000000013323 ) ) ;
#9850=CARTESIAN_POINT ( 'NONE',  ( -60.99999999999998579, 15.22916666666666607, 2.077350269189628840 ) ) ;
#9852=CARTESIAN_POINT ( 'NONE',  ( -60.99999999999998579, 13.73958333265053611, 0.9226497308103762673 ) ) ;
#9853=CARTESIAN_POINT ( 'NONE',  ( -61.13531646874998415, 14.09895833299193413, 1.000774730468978468 ) ) ;
#9854=CARTESIAN_POINT ( 'NONE',  ( -61.99999999999999289, 10.39062499965860198, 0.5015494609379544944 ) ) ;
#9856=EDGE_LOOP ( 'NONE', ( #2214, #9034, #6781, #2803 ) ) ;
#9858=CARTESIAN_POINT ( 'NONE',  ( -61.13531646874997705, 11.91145833299193413, 1.000774730468978468 ) ) ;
#9861=CARTESIAN_POINT ( 'NONE',  ( -61.99999999999998579, 16.00000000000000000, 1.500000000000002220 ) ) ;
#9862=CARTESIAN_POINT ( 'NONE',  ( -62.99999999999998579, 15.57291666598387003, 0.9226497308103756012 ) ) ;
#9866=EDGE_CURVE ( 'NONE', #2471, #2202, #8659, .T. ) ;
#9867=CARTESIAN_POINT ( 'NONE',  ( -62.86468353124999453, 13.97395833299193413, 1.999225269531025750 ) ) ;
#9868=CARTESIAN_POINT ( 'NONE',  ( -61.56765823437498852, 9.786458332991934128, 2.248837904296538515 ) ) ;
#9869=CARTESIAN_POINT ( 'NONE',  ( -62.26794919243111082, 8.426335450315370679, 2.500000000000001776 ) ) ;
#9871=CARTESIAN_POINT ( 'NONE',  ( -62.99999999999998579, 13.89583333333333393, 2.077350269189627952 ) ) ;
#9872=DIRECTION ( 'NONE',  ( -0.000000000000000000, -1.000000000000000000, -0.000000000000000000 ) ) ;
#9875=CARTESIAN_POINT ( 'NONE',  ( -62.49999999999998579, 11.88541666598387003, 2.366025403784441483 ) ) ;
#9878=CARTESIAN_POINT ( 'NONE',  ( -61.56765823437498142, 13.11979166632526805, 0.7511620957034663704 ) ) ;
#9880=ORIENTED_EDGE ( 'NONE', *, *, #7451, .T. ) ;
#9881=CARTESIAN_POINT ( 'NONE',  ( -61.13531646874998415, 11.39062499965860020, 1.500000000000002220 ) ) ;
#9883=CARTESIAN_POINT ( 'NONE',  ( -61.99999999999998579, 15.45312499965860020, 0.5015494609379544944 ) ) ;
#9886=ORIENTED_EDGE ( 'NONE', *, *, #2096, .T. ) ;
#9888=CARTESIAN_POINT ( 'NONE',  ( -60.99999999999998579, 10.02083333333333215, 0.9226497308103762673 ) ) ;
#9889=CARTESIAN_POINT ( 'NONE',  ( -61.99999999999998579, 16.00000000000000000, 0.5000000000000041078 ) ) ;
#9890=CARTESIAN_POINT ( 'NONE',  ( -61.73205080756886787, 8.448664549684631098, 2.500000000000004885 ) ) ;
#9891=DIRECTION ( 'NONE',  ( 0.000000000000000000, 0.000000000000000000, -1.000000000000000000 ) ) ;
#9892=CARTESIAN_POINT ( 'NONE',  ( -62.99999999999998579, 8.572916665983868256, 0.9226497308103756012 ) ) ;
#9893=CARTESIAN_POINT ( 'NONE',  ( -61.99999999999998579, 11.57812499965860198, 2.498450539062049724 ) ) ;
#9896=ORIENTED_EDGE ( 'NONE', *, *, #8228, .F. ) ;
#9897=CARTESIAN_POINT ( 'NONE',  ( -61.99999999999998579, 15.43749999999999822, 2.500000000000002665 ) ) ;
#9903=CARTESIAN_POINT ( 'NONE',  ( -62.43234176562498305, 14.41145833299193413, 0.7511620957034662593 ) ) ;
#9904=CARTESIAN_POINT ( 'NONE',  ( -62.86468353124999453, 9.953124999658601979, 1.500000000000002220 ) ) ;
#9905=CARTESIAN_POINT ( 'NONE',  ( -61.99999999999998579, 14.43749999999999822, 2.500000000000002665 ) ) ;
#9906=VERTEX_POINT ( 'NONE', #8776 ) ;
#9907=CARTESIAN_POINT ( 'NONE',  ( -61.99999999999998579, 8.406249999317203958, 2.500000000000003109 ) ) ;
#9908=CARTESIAN_POINT ( 'NONE',  ( -61.99999999999999289, 11.70312499965860198, 0.5015494609379544944 ) ) ;
#9910=CARTESIAN_POINT ( 'NONE',  ( -61.13531646874998415, 15.61979166632526628, 1.999225269531026417 ) ) ;
#9912=CARTESIAN_POINT ( 'NONE',  ( -61.99999999999998579, 15.18750000000000000, 2.500000000000002665 ) ) ;
#9913=CARTESIAN_POINT ( 'NONE',  ( -62.49999999999998579, 16.13541666598386826, 2.366025403784441483 ) ) ;
#9915=EDGE_LOOP ( 'NONE', ( #4107, #8599, #7144, #2890 ) ) ;
#9916=CARTESIAN_POINT ( 'NONE',  ( -62.49999999999998579, 11.88541666598387003, 2.366025403784441483 ) ) ;
#9918=EDGE_CURVE ( 'NONE', #1268, #1104, #2269, .T. ) ;
#9919=AXIS2_PLACEMENT_3D ( 'NONE', #6051, #3382, #9438 ) ;
#9920=CARTESIAN_POINT ( 'NONE',  ( -61.13531646874998415, 14.82812499965860020, 1.500000000000002220 ) ) ;
#9921=CARTESIAN_POINT ( 'NONE',  ( -62.86468353124999453, 9.453124999658600203, 1.500000000000002220 ) ) ;
#9922=AXIS2_PLACEMENT_3D ( 'NONE', #2779, #221, #6340 ) ;
#9923=DIRECTION ( 'NONE',  ( -0.000000000000000000, -1.000000000000000000, -0.000000000000000000 ) ) ;
#9925=CARTESIAN_POINT ( 'NONE',  ( -62.99999999999998579, 13.87500000000000000, 1.500000000000001998 ) ) ;
#9926=CARTESIAN_POINT ( 'NONE',  ( -62.49999999999998579, 8.635416665983868256, 2.366025403784441483 ) ) ;
#9929=CARTESIAN_POINT ( 'NONE',  ( -62.99999999999998579, 11.86458333265053611, 2.077350269189627952 ) ) ;
#9931=( BOUNDED_CURVE ( )  B_SPLINE_CURVE ( 2, ( #1095, #1035, #1213, #7046, #7825, #4482, #3770, #2106, #9660 ),
 .UNSPECIFIED., .F., .F. ) 
 B_SPLINE_CURVE_WITH_KNOTS ( ( 3, 2, 2, 2, 3 ),
 ( 0.9140625000000000000, 0.9166666666666666297, 0.9218750000000000000, 0.9270833333333333703, 0.9296875000000000000 ),
 .UNSPECIFIED. ) 
 CURVE ( )  GEOMETRIC_REPRESENTATION_ITEM ( )  RATIONAL_B_SPLINE_CURVE ( ( 0.9330127018922194093, 0.9330127018922194093, 1.000000000000000000, 0.8660254037844387076, 1.000000000000000000, 0.8660254037844387076, 1.000000000000000000, 0.9330127018922194093, 0.9330127018922194093 ) ) 
 REPRESENTATION_ITEM ( '' )  );
#9932=CARTESIAN_POINT ( 'NONE',  ( -61.56765823437498852, 13.78645833299193413, 2.248837904296538515 ) ) ;
#9934=VERTEX_POINT ( 'NONE', #1337 ) ;
#9936=CARTESIAN_POINT ( 'NONE',  ( -62.86468353124999453, 12.01562499965860198, 1.500000000000002220 ) ) ;
#9937=LINE ( 'NONE', #3990, #9364 ) ;
#9938=EDGE_CURVE ( 'NONE', #3002, #8372, #3457, .T. ) ;
#9940=ORIENTED_EDGE ( 'NONE', *, *, #8649, .F. ) ;
#9941=CARTESIAN_POINT ( 'NONE',  ( -62.26794919243111082, 11.07366454968462932, 0.5000000000000013323 ) ) ;
#9943=ORIENTED_EDGE ( 'NONE', *, *, #10676, .F. ) ;
#9946=CARTESIAN_POINT ( 'NONE',  ( -62.99999999999998579, 9.354166666666666075, 0.9226497308103756012 ) ) ;
#9948=CARTESIAN_POINT ( 'NONE',  ( -60.99999999999998579, 14.98958333265053611, 0.9226497308103762673 ) ) ;
#9949=CYLINDRICAL_SURFACE ( 'NONE', #2630, 0.9999999999999981126 ) ;
#9951=CYLINDRICAL_SURFACE ( 'NONE', #10624, 0.9999999999999981126 ) ;
#9952=CARTESIAN_POINT ( 'NONE',  ( -61.99999999999998579, 11.32812499965860020, 2.498450539062049724 ) ) ;
#9955=CARTESIAN_POINT ( 'NONE',  ( -61.49999999999998579, 9.260416665983870033, 0.6339745962155628467 ) ) ;
#9956=ORIENTED_EDGE ( 'NONE', *, *, #7256, .F. ) ;
#9957=CARTESIAN_POINT ( 'NONE',  ( -60.99999999999998579, 13.71874999931720218, 1.500000000000002220 ) ) ;
#9958=CARTESIAN_POINT ( 'NONE',  ( -61.56765823437498852, 14.28645833299193413, 2.248837904296538515 ) ) ;
#9962=CARTESIAN_POINT ( 'NONE',  ( -61.99999999999998579, 16.00000000000000000, 0.5000000000000041078 ) ) ;
#9963=CARTESIAN_POINT ( 'NONE',  ( -62.86468353124999453, 12.01562499965860198, 1.500000000000002220 ) ) ;
#9964=CARTESIAN_POINT ( 'NONE',  ( -61.99999999999998579, 15.20312499965860020, 0.5015494609379544944 ) ) ;
#9965=CARTESIAN_POINT ( 'NONE',  ( -61.56765823437498852, 16.03645833299193768, 2.248837904296538515 ) ) ;
#9966=CARTESIAN_POINT ( 'NONE',  ( -62.49999999999998579, 15.55208333265053611, 0.6339745962155627357 ) ) ;
#9972=CARTESIAN_POINT ( 'NONE',  ( -61.99999999999999289, 14.39062499965860198, 0.5015494609379544944 ) ) ;
#9973=CARTESIAN_POINT ( 'NONE',  ( -62.86468353124998742, 9.223958332991935904, 1.999225269531025972 ) ) ;
#9975=CARTESIAN_POINT ( 'NONE',  ( -61.13531646874997705, 15.86979166632526628, 1.999225269531026417 ) ) ;
#9977=ORIENTED_EDGE ( 'NONE', *, *, #4185, .F. ) ;
#9978=CARTESIAN_POINT ( 'NONE',  ( -62.49999999999998579, 13.66666666666666785, 2.366025403784441483 ) ) ;
#9979=CARTESIAN_POINT ( 'NONE',  ( -62.99999999999998579, 11.07291666598386826, 0.9226497308103756012 ) ) ;
#9981=CARTESIAN_POINT ( 'NONE',  ( -60.99999999999998579, 11.73958333265053788, 0.9226497308103762673 ) ) ;
#9982=DIRECTION ( 'NONE',  ( 0.000000000000000000, 0.000000000000000000, -1.000000000000000000 ) ) ;
#9983=CARTESIAN_POINT ( 'NONE',  ( -61.56765823437498852, 14.53645833299193413, 2.248837904296538515 ) ) ;
#9984=DIRECTION ( 'NONE',  ( -0.000000000000000000, -1.000000000000000000, -0.000000000000000000 ) ) ;
#9985=ORIENTED_EDGE ( 'NONE', *, *, #1448, .F. ) ;
#9988=CARTESIAN_POINT ( 'NONE',  ( -61.13531646874998415, 11.41145833299193590, 1.000774730468978468 ) ) ;
#9989=CARTESIAN_POINT ( 'NONE',  ( -60.99999999999998579, 12.23958333265053611, 0.9226497308103762673 ) ) ;
#9990=CARTESIAN_POINT ( 'NONE',  ( -61.56765823437498142, 15.18229166632526805, 0.7511620957034663704 ) ) ;
#9992=CARTESIAN_POINT ( 'NONE',  ( -62.26794919243111082, 11.17633545031536890, 2.500000000000003109 ) ) ;
#9993=ORIENTED_EDGE ( 'NONE', *, *, #5031, .F. ) ;
#9994=CARTESIAN_POINT ( 'NONE',  ( -61.49999999999998579, 9.427083332650536107, 2.366025403784441927 ) ) ;
#9995=CARTESIAN_POINT ( 'NONE',  ( -62.49999999999998579, 9.833333333333332149, 0.6339745962155627357 ) ) ;
#9996=DIRECTION ( 'NONE',  ( 0.000000000000000000, 0.000000000000000000, -1.000000000000000000 ) ) ;
#9997=CARTESIAN_POINT ( 'NONE',  ( -61.49999999999998579, 8.208333333333333925, 2.366025403784441927 ) ) ;
#10000=CARTESIAN_POINT ( 'NONE',  ( -62.49999999999998579, 9.135416665983868256, 2.366025403784441483 ) ) ;
#10001=CARTESIAN_POINT ( 'NONE',  ( -61.13531646874998415, 11.41145833299193590, 1.000774730468978468 ) ) ;
#10004=LINE ( 'NONE', #3277, #8883 ) ;
#10008=CARTESIAN_POINT ( 'NONE',  ( -61.13531646874998415, 14.05729166632526805, 1.999225269531026417 ) ) ;
#10010=CARTESIAN_POINT ( 'NONE',  ( -62.86468353124998032, 13.24479166632526983, 1.000774730468978024 ) ) ;
#10011=CARTESIAN_POINT ( 'NONE',  ( -62.43234176562498305, 15.97395833299193590, 0.7511620957034662593 ) ) ;
#10015=CARTESIAN_POINT ( 'NONE',  ( -61.13531646874998415, 8.411458332991934128, 1.000774730468978468 ) ) ;
#10020=CARTESIAN_POINT ( 'NONE',  ( -61.99999999999999289, 14.64062499965859843, 0.5015494609379544944 ) ) ;
#10021=CARTESIAN_POINT ( 'NONE',  ( -62.43234176562499016, 9.994791666325268054, 2.248837904296538071 ) ) ;
#10022=CARTESIAN_POINT ( 'NONE',  ( -61.99999999999999289, 8.140624999658601979, 0.5015494609379544944 ) ) ;
#10025=CARTESIAN_POINT ( 'NONE',  ( -62.99999999999998579, 13.60416666666666607, 0.9226497308103756012 ) ) ;
#10026=CARTESIAN_POINT ( 'NONE',  ( -61.13531646874997705, 8.161458332991934128, 1.000774730468978468 ) ) ;
#10028=CARTESIAN_POINT ( 'NONE',  ( -61.49999999999998579, 11.42708333265053611, 2.366025403784441927 ) ) ;
#10030=ADVANCED_FACE ( 'NONE', ( #8945 ), #5759, .T. ) ;
#10031=CARTESIAN_POINT ( 'NONE',  ( -61.13531646874998415, 13.32812499965860020, 1.500000000000002220 ) ) ;
#10034=CARTESIAN_POINT ( 'NONE',  ( -62.43234176562498305, 10.97395833299193590, 0.7511620957034662593 ) ) ;
#10035=PLANE ( 'NONE',  #3171 ) ;
#10039=EDGE_CURVE ( 'NONE', #8495, #6754, #9937, .T. ) ;
#10040=ORIENTED_EDGE ( 'NONE', *, *, #3970, .F. ) ;
#10041=CARTESIAN_POINT ( 'NONE',  ( -61.99999999999998579, 15.56249999999999822, 0.5000000000000013323 ) ) ;
#10042=CARTESIAN_POINT ( 'NONE',  ( -61.99999999999998579, 10.81249999999999822, 0.3452994616207497591 ) ) ;
#10044=DIRECTION ( 'NONE',  ( -0.000000000000000000, -1.000000000000000000, -0.000000000000000000 ) ) ;
#10046=CARTESIAN_POINT ( 'NONE',  ( -62.86468353124998742, 13.03645833299193235, 1.999225269531025972 ) ) ;
#10047=CARTESIAN_POINT ( 'NONE',  ( -61.99999999999998579, 12.03124999931720041, 0.5000000000000013323 ) ) ;
#10049=CARTESIAN_POINT ( 'NONE',  ( -62.49999999999998579, 15.33333333333333393, 0.6339745962155627357 ) ) ;
#10050=VERTEX_POINT ( 'NONE', #9101 ) ;
#10052=CARTESIAN_POINT ( 'NONE',  ( -62.86468353124998742, 15.72395833299193768, 1.999225269531025972 ) ) ;
#10053=CARTESIAN_POINT ( 'NONE',  ( -61.99999999999998579, 11.81249999999999822, 0.5000000000000013323 ) ) ;
#10056=CARTESIAN_POINT ( 'NONE',  ( -61.13531646874997705, 12.91145833299193590, 1.000774730468978468 ) ) ;
#10057=CARTESIAN_POINT ( 'NONE',  ( -61.13531646874998415, 15.39062499965860020, 1.500000000000002220 ) ) ;
#10058=CARTESIAN_POINT ( 'NONE',  ( -60.99999999999998579, 15.00000000000000000, 1.500000000000002220 ) ) ;
#10059=CARTESIAN_POINT ( 'NONE',  ( -61.73205080756886076, 13.41741454900182973, 2.500000000000003109 ) ) ;
#10061=CARTESIAN_POINT ( 'NONE',  ( -62.43234176562498305, 8.223958332991934128, 0.7511620957034662593 ) ) ;
#10064=CARTESIAN_POINT ( 'NONE',  ( -61.99999999999998579, 11.90624999931720041, 2.500000000000002665 ) ) ;
#10066=CARTESIAN_POINT ( 'NONE',  ( -61.13531646874997705, 13.84895833299193413, 1.000774730468978468 ) ) ;
#10067=CARTESIAN_POINT ( 'NONE',  ( -62.86468353124999453, 9.203124999658600203, 1.500000000000002220 ) ) ;
#10070=CARTESIAN_POINT ( 'NONE',  ( -61.49999999999998579, 13.79166666666666785, 0.6339745962155628467 ) ) ;
#10071=CARTESIAN_POINT ( 'NONE',  ( -62.86468353124998032, 8.994791666325268054, 1.000774730468978024 ) ) ;
#10072=SHAPE_REPRESENTATION_RELATIONSHIP ( 'NONE' , 'NONE' ,  #6156, #6440 ) ;
#10073=CARTESIAN_POINT ( 'NONE',  ( -62.99999999999998579, 12.32291666598386826, 0.9226497308103756012 ) ) ;
#10077=CARTESIAN_POINT ( 'NONE',  ( -62.43234176562498305, 13.41145833299193413, 0.7511620957034662593 ) ) ;
#10081=ADVANCED_FACE ( 'NONE', ( #7437 ), #9829, .T. ) ;
#10082=CARTESIAN_POINT ( 'NONE',  ( -62.86468353124998032, 13.49479166632526805, 1.000774730468978246 ) ) ;
#10083=CARTESIAN_POINT ( 'NONE',  ( -61.49999999999998579, 11.42708333265053611, 2.366025403784441927 ) ) ;
#10084=AXIS2_PLACEMENT_3D ( 'NONE', #4918, #10919, #8316 ) ;
#10087=ORIENTED_EDGE ( 'NONE', *, *, #7541, .T. ) ;
#10088=CARTESIAN_POINT ( 'NONE',  ( -61.99999999999998579, 12.43749999999999822, 2.500000000000002665 ) ) ;
#10089=AXIS2_PLACEMENT_3D ( 'NONE', #8821, #1207, #4586 ) ;
#10090=ORIENTED_EDGE ( 'NONE', *, *, #7319, .F. ) ;
#10091=CARTESIAN_POINT ( 'NONE',  ( -60.99999999999998579, 10.47916666666666607, 2.077350269189628840 ) ) ;
#10093=CARTESIAN_POINT ( 'NONE',  ( -61.13531646874998415, 8.369791666325268054, 1.999225269531026417 ) ) ;
#10096=EDGE_CURVE ( 'NONE', #4846, #562, #2822, .T. ) ;
#10097=CARTESIAN_POINT ( 'NONE',  ( -61.99999999999998579, 13.45312499965860376, 0.5015494609379544944 ) ) ;
#10100=VERTEX_POINT ( 'NONE', #2480 ) ;
#10101=ORIENTED_EDGE ( 'NONE', *, *, #10904, .F. ) ;
#10102=CARTESIAN_POINT ( 'NONE',  ( -62.43234176562499016, 14.99479166632526805, 2.248837904296538071 ) ) ;
#10104=CARTESIAN_POINT ( 'NONE',  ( -62.99999999999998579, 8.104166666666667851, 0.9226497308103756012 ) ) ;
#10105=( BOUNDED_CURVE ( )  B_SPLINE_CURVE ( 2, ( #5004, #3292, #638, #3137, #7520, #5741, #9916, #7414, #10064 ),
 .UNSPECIFIED., .F., .T. ) 
 B_SPLINE_CURVE_WITH_KNOTS ( ( 3, 2, 2, 2, 3 ),
 ( 0.4453125000000000000, 0.4479166666666666852, 0.4531250000000000000, 0.4583333333333333148, 0.4609375000000000000 ),
 .UNSPECIFIED. ) 
 CURVE ( )  GEOMETRIC_REPRESENTATION_ITEM ( )  RATIONAL_B_SPLINE_CURVE ( ( 0.9330127018922194093, 0.9330127018922194093, 1.000000000000000000, 0.8660254037844387076, 1.000000000000000000, 0.8660254037844387076, 1.000000000000000000, 0.9330127018922194093, 0.9330127018922194093 ) ) 
 REPRESENTATION_ITEM ( '' )  );
#10107=CARTESIAN_POINT ( 'NONE',  ( -61.56765823437498852, 13.09895833299193413, 2.248837904296538515 ) ) ;
#10108=CARTESIAN_POINT ( 'NONE',  ( -61.56765823437498852, 15.84895833299193590, 2.248837904296538515 ) ) ;
#10109=DIRECTION ( 'NONE',  ( 0.000000000000000000, 0.000000000000000000, -1.000000000000000000 ) ) ;
#10110=CARTESIAN_POINT ( 'NONE',  ( -61.99999999999998579, 8.562500000000000000, 0.5000000000000013323 ) ) ;
#10111=CARTESIAN_POINT ( 'NONE',  ( -61.99999999999998579, 9.203124999658601979, 0.5015494609379544944 ) ) ;
#10112=CARTESIAN_POINT ( 'NONE',  ( -61.99999999999998579, 16.00000000000000000, 1.500000000000002220 ) ) ;
#10113=ORIENTED_EDGE ( 'NONE', *, *, #3403, .F. ) ;
#10116=CARTESIAN_POINT ( 'NONE',  ( -61.13531646874997705, 16.05729166632526628, 1.999225269531026417 ) ) ;
#10117=CARTESIAN_POINT ( 'NONE',  ( -61.13531646874998415, 11.80729166632526805, 1.999225269531026417 ) ) ;
#10118=CARTESIAN_POINT ( 'NONE',  ( -62.43234176562498305, 15.97395833299193590, 0.7511620957034662593 ) ) ;
#10121=CARTESIAN_POINT ( 'NONE',  ( -61.49999999999998579, 14.45833333333333393, 2.366025403784441927 ) ) ;
#10122=CARTESIAN_POINT ( 'NONE',  ( -61.13531646874997705, 8.661458332991934128, 1.000774730468978468 ) ) ;
#10123=CARTESIAN_POINT ( 'NONE',  ( -61.49999999999998579, 12.67708333265053611, 2.366025403784441927 ) ) ;
#10125=ADVANCED_FACE ( 'NONE', ( #1701 ), #810, .T. ) ;
#10127=AXIS2_PLACEMENT_3D ( 'NONE', #4131, #9923, #10908 ) ;
#10128=CARTESIAN_POINT ( 'NONE',  ( -62.86468353124998032, 13.43229166632526628, 1.000774730468978246 ) ) ;
#10129=ADVANCED_FACE ( 'NONE', ( #10188 ), #9207, .T. ) ;
#10133=CARTESIAN_POINT ( 'NONE',  ( -62.86468353124999453, 13.01562499965860198, 1.500000000000002220 ) ) ;
#10134=CARTESIAN_POINT ( 'NONE',  ( -61.99999999999998579, 16.00000000000000000, 1.500000000000002220 ) ) ;
#10138=CARTESIAN_POINT ( 'NONE',  ( -62.49999999999998579, 12.33333333333333393, 0.6339745962155627357 ) ) ;
#10142=CARTESIAN_POINT ( 'NONE',  ( -62.49999999999998579, 11.41666666666666785, 2.366025403784441483 ) ) ;
#10144=CARTESIAN_POINT ( 'NONE',  ( -62.86468353124999453, 8.515624999658601979, 1.500000000000002220 ) ) ;
#10148=VECTOR ( 'NONE', #1018, 999.9999999999998863 ) ;
#10149=CARTESIAN_POINT ( 'NONE',  ( -62.43234176562499016, 13.80729166632526805, 2.248837904296538071 ) ) ;
#10150=CARTESIAN_POINT ( 'NONE',  ( -62.99999999999998579, 12.82291666598386826, 0.9226497308103756012 ) ) ;
#10153=ADVANCED_FACE ( 'NONE', ( #8427 ), #3259, .T. ) ;
#10154=ORIENTED_EDGE ( 'NONE', *, *, #8180, .F. ) ;
#10156=CARTESIAN_POINT ( 'NONE',  ( -60.99999999999998579, 13.21874999931720396, 1.500000000000002220 ) ) ;
#10157=CARTESIAN_POINT ( 'NONE',  ( -61.99999999999998579, 15.26562499965860020, 2.498450539062049724 ) ) ;
#10160=CARTESIAN_POINT ( 'NONE',  ( -62.43234176562499016, 12.30729166632526805, 2.248837904296538071 ) ) ;
#10161=CARTESIAN_POINT ( 'NONE',  ( -61.99999999999998579, 8.390624999658601979, 0.5015494609379544944 ) ) ;
#10163=DIRECTION ( 'NONE',  ( 0.000000000000000000, 0.000000000000000000, -1.000000000000000000 ) ) ;
#10164=CARTESIAN_POINT ( 'NONE',  ( -61.56765823437498852, 9.098958332991935904, 2.248837904296538515 ) ) ;
#10165=CARTESIAN_POINT ( 'NONE',  ( -61.49999999999998579, 15.67708333265053611, 2.366025403784441927 ) ) ;
#10170=( BOUNDED_CURVE ( )  B_SPLINE_CURVE ( 2, ( #7778, #8552, #160, #6889, #10260, #3544, #2669, #6944, #10320 ),
 .UNSPECIFIED., .F., .T. ) 
 B_SPLINE_CURVE_WITH_KNOTS ( ( 3, 2, 2, 2, 3 ),
 ( 0.3515625000000000000, 0.3541666666666666852, 0.3593750000000000000, 0.3645833333333333148, 0.3671875000000000000 ),
 .UNSPECIFIED. ) 
 CURVE ( )  GEOMETRIC_REPRESENTATION_ITEM ( )  RATIONAL_B_SPLINE_CURVE ( ( 0.9330127018922194093, 0.9330127018922194093, 1.000000000000000000, 0.8660254037844387076, 1.000000000000000000, 0.8660254037844387076, 1.000000000000000000, 0.9330127018922194093, 0.9330127018922194093 ) ) 
 REPRESENTATION_ITEM ( '' )  );
#10171=CARTESIAN_POINT ( 'NONE',  ( -61.99999999999999289, 15.39062499965860020, 0.5015494609379544944 ) ) ;
#10172=EDGE_CURVE ( 'NONE', #5931, #5580, #2646, .T. ) ;
#10173=CARTESIAN_POINT ( 'NONE',  ( -62.86468353124999453, 11.70312499965860198, 1.500000000000002220 ) ) ;
#10174=CARTESIAN_POINT ( 'NONE',  ( -62.43234176562499016, 16.05729166632526628, 2.248837904296538071 ) ) ;
#10175=CARTESIAN_POINT ( 'NONE',  ( -62.99999999999998579, 13.09374999931720396, 1.500000000000001998 ) ) ;
#10176=ORIENTED_EDGE ( 'NONE', *, *, #821, .T. ) ;
#10177=CARTESIAN_POINT ( 'NONE',  ( -62.49999999999998579, 15.58333333333333393, 0.6339745962155627357 ) ) ;
#10178=CARTESIAN_POINT ( 'NONE',  ( -61.99999999999999289, 8.703124999658601979, 0.5015494609379544944 ) ) ;
#10179=CARTESIAN_POINT ( 'NONE',  ( -62.99999999999998579, 12.84374999931720396, 1.500000000000001998 ) ) ;
#10180=CARTESIAN_POINT ( 'NONE',  ( -62.99999999999998579, 14.62500000000000000, 1.500000000000001998 ) ) ;
#10182=CARTESIAN_POINT ( 'NONE',  ( -61.13531646874998415, 11.82812499965860198, 1.500000000000002220 ) ) ;
#10187=CARTESIAN_POINT ( 'NONE',  ( -61.13531646874998415, 12.39062499965860198, 1.500000000000002220 ) ) ;
#10188=FACE_OUTER_BOUND ( 'NONE', #6456, .T. ) ;
#10189=CARTESIAN_POINT ( 'NONE',  ( -61.99999999999998579, 9.531249999317203958, 0.3452994616207497591 ) ) ;
#10190=ORIENTED_EDGE ( 'NONE', *, *, #9781, .F. ) ;
#10191=ADVANCED_FACE ( 'NONE', ( #4973 ), #2585, .T. ) ;
#10193=ORIENTED_EDGE ( 'NONE', *, *, #1647, .F. ) ;
#10194=DIRECTION ( 'NONE',  ( 0.000000000000000000, 0.000000000000000000, -1.000000000000000000 ) ) ;
#10195=CARTESIAN_POINT ( 'NONE',  ( -62.86468353124998742, 10.97395833299193768, 1.999225269531025972 ) ) ;
#10198=CARTESIAN_POINT ( 'NONE',  ( -62.86468353124998742, 9.036458332991934128, 1.999225269531025972 ) ) ;
#10199=CARTESIAN_POINT ( 'NONE',  ( -61.99999999999998579, 14.18750000000000000, 2.500000000000002665 ) ) ;
#10200=CARTESIAN_POINT ( 'NONE',  ( -61.99999999999998579, 13.57812499965860020, 2.498450539062049724 ) ) ;
#10202=CARTESIAN_POINT ( 'NONE',  ( -62.49999999999998579, 9.333333333333333925, 0.6339745962155627357 ) ) ;
#10204=CARTESIAN_POINT ( 'NONE',  ( -62.26794919243111082, 11.64508544963257286, 2.500000000000006217 ) ) ;
#10205=CARTESIAN_POINT ( 'NONE',  ( -62.86468353124999453, 15.45312499965860020, 1.500000000000002220 ) ) ;
#10206=CARTESIAN_POINT ( 'NONE',  ( -61.99999999999998579, 16.00000000000000000, 1.500000000000002220 ) ) ;
#10208=CARTESIAN_POINT ( 'NONE',  ( -62.99999999999998579, 8.875000000000001776, 1.500000000000001998 ) ) ;
#10209=CARTESIAN_POINT ( 'NONE',  ( -61.99999999999999289, 12.45312499965860020, 0.5015494609379544944 ) ) ;
#10210=CARTESIAN_POINT ( 'NONE',  ( -61.56765823437498852, 8.536458332991934128, 2.248837904296538515 ) ) ;
#10211=EDGE_CURVE ( 'NONE', #4762, #4311, #4664, .T. ) ;
#10213=CARTESIAN_POINT ( 'NONE',  ( -60.99999999999998579, 13.44791666598387003, 2.077350269189628840 ) ) ;
#10214=CARTESIAN_POINT ( 'NONE',  ( -61.99999999999998579, 9.328124999658600203, 2.498450539062049724 ) ) ;
#10215=CARTESIAN_POINT ( 'NONE',  ( -61.99999999999998579, 16.00000000000000000, 1.500000000000002220 ) ) ;
#10216=ORIENTED_EDGE ( 'NONE', *, *, #6766, .T. ) ;
#10218=CARTESIAN_POINT ( 'NONE',  ( -62.26794919243111082, 11.42633545031537068, 2.500000000000006217 ) ) ;
#10219=CARTESIAN_POINT ( 'NONE',  ( -62.43234176562498305, 15.41145833299193590, 0.7511620957034662593 ) ) ;
#10220=CARTESIAN_POINT ( 'NONE',  ( -61.99999999999998579, 10.89062499965860020, 0.5015494609379544944 ) ) ;
#10221=CARTESIAN_POINT ( 'NONE',  ( -62.86468353124999453, 9.473958332991934128, 1.999225269531025750 ) ) ;
#10222=CARTESIAN_POINT ( 'NONE',  ( -62.26794919243111082, 13.14508544963257286, 2.500000000000003109 ) ) ;
#10224=CARTESIAN_POINT ( 'NONE',  ( -62.99999999999998579, 15.35416666666666785, 0.9226497308103756012 ) ) ;
#10226=CARTESIAN_POINT ( 'NONE',  ( -60.99999999999998579, 12.69791666598386826, 2.077350269189628840 ) ) ;
#10229=ADVANCED_FACE ( 'NONE', ( #7590 ), #10035, .F. ) ;
#10231=( BOUNDED_CURVE ( )  B_SPLINE_CURVE ( 2, ( #229, #7680, #114, #62, #5215, #3614, #6174, #4378, #7791 ),
 .UNSPECIFIED., .F., .T. ) 
 B_SPLINE_CURVE_WITH_KNOTS ( ( 3, 2, 2, 2, 3 ),
 ( 0.7265625000000000000, 0.7291666666666666297, 0.7343750000000000000, 0.7395833333333333703, 0.7421875000000000000 ),
 .UNSPECIFIED. ) 
 CURVE ( )  GEOMETRIC_REPRESENTATION_ITEM ( )  RATIONAL_B_SPLINE_CURVE ( ( 0.9330127018922194093, 0.9330127018922194093, 1.000000000000000000, 0.8660254037844387076, 1.000000000000000000, 0.8660254037844387076, 1.000000000000000000, 0.9330127018922194093, 0.9330127018922194093 ) ) 
 REPRESENTATION_ITEM ( '' )  );
#10233=CARTESIAN_POINT ( 'NONE',  ( -62.86468353124999453, 11.20312499965860020, 1.500000000000002220 ) ) ;
#10238=CARTESIAN_POINT ( 'NONE',  ( -62.86468353124998742, 12.78645833299193413, 1.999225269531025972 ) ) ;
#10239=CARTESIAN_POINT ( 'NONE',  ( -61.73205080756886076, 11.52008544963257108, 0.5000000000000014433 ) ) ;
#10241=CARTESIAN_POINT ( 'NONE',  ( -62.49999999999998579, 8.885416665983868256, 2.366025403784441483 ) ) ;
#10246=CARTESIAN_POINT ( 'NONE',  ( -62.99999999999998579, 12.37500000000000000, 1.500000000000001998 ) ) ;
#10247=CARTESIAN_POINT ( 'NONE',  ( -62.86468353124999453, 11.45312499965860020, 1.500000000000002220 ) ) ;
#10250=EDGE_LOOP ( 'NONE', ( #923, #2434, #7443, #347 ) ) ;
#10251=CARTESIAN_POINT ( 'NONE',  ( -61.99999999999998579, 8.578124999658601979, 2.498450539062049724 ) ) ;
#10252=CARTESIAN_POINT ( 'NONE',  ( -61.99999999999997868, 10.53124999931720573, 0.5000000000000013323 ) ) ;
#10254=CARTESIAN_POINT ( 'NONE',  ( -61.13531646874998415, 13.36979166632526628, 1.999225269531026417 ) ) ;
#10256=EDGE_LOOP ( 'NONE', ( #2195, #3712, #2326, #4431 ) ) ;
#10259=VERTEX_POINT ( 'NONE', #6866 ) ;
#10260=CARTESIAN_POINT ( 'NONE',  ( -62.99999999999998579, 10.87500000000000000, 1.500000000000001998 ) ) ;
#10262=CARTESIAN_POINT ( 'NONE',  ( -61.56765823437498142, 14.61979166632526805, 0.7511620957034663704 ) ) ;
#10265=LINE ( 'NONE', #8557, #1389 ) ;
#10266=CARTESIAN_POINT ( 'NONE',  ( -61.99999999999999289, 13.95312499965860198, 0.5015494609379544944 ) ) ;
#10267=CARTESIAN_POINT ( 'NONE',  ( -61.99999999999998579, 9.265624999658600203, 2.498450539062049724 ) ) ;
#10268=DIRECTION ( 'NONE',  ( 0.000000000000000000, 0.000000000000000000, -1.000000000000000000 ) ) ;
#10269=CARTESIAN_POINT ( 'NONE',  ( -61.99999999999998579, 16.00000000000000000, 0.5000000000000041078 ) ) ;
#10270=CARTESIAN_POINT ( 'NONE',  ( -62.86468353124998032, 9.494791666325269830, 1.000774730468978246 ) ) ;
#10271=DIRECTION ( 'NONE',  ( 0.000000000000000000, 1.000000000000000000, 0.000000000000000000 ) ) ;
#10272=ORIENTED_EDGE ( 'NONE', *, *, #10968, .F. ) ;
#10273=CARTESIAN_POINT ( 'NONE',  ( -61.99999999999998579, 16.00000000000000000, 2.500000000000000444 ) ) ;
#10274=CARTESIAN_POINT ( 'NONE',  ( -61.99999999999998579, 16.00000000000000000, 1.500000000000002220 ) ) ;
#10276=EDGE_CURVE ( 'NONE', #8261, #5305, #4090, .T. ) ;
#10278=CARTESIAN_POINT ( 'NONE',  ( -61.99999999999999289, 15.89062499965860198, 0.5015494609379544944 ) ) ;
#10279=CARTESIAN_POINT ( 'NONE',  ( -62.86468353124999453, 11.20312499965860020, 1.500000000000002220 ) ) ;
#10280=CARTESIAN_POINT ( 'NONE',  ( -61.13531646874997705, 8.598958332991934128, 1.000774730468978468 ) ) ;
#10281=VERTEX_POINT ( 'NONE', #32 ) ;
#10282=CARTESIAN_POINT ( 'NONE',  ( -60.99999999999998579, 15.27083333333333393, 0.9226497308103762673 ) ) ;
#10283=CARTESIAN_POINT ( 'NONE',  ( -62.43234176562499016, 10.05729166632526805, 2.248837904296538071 ) ) ;
#10285=CARTESIAN_POINT ( 'NONE',  ( -61.99999999999998579, 13.78124999931720218, 0.3452994616207497591 ) ) ;
#10288=EDGE_CURVE ( 'NONE', #3072, #8746, #5130, .T. ) ;
#10289=CARTESIAN_POINT ( 'NONE',  ( -62.26794919243111082, 11.57366454968462932, 0.5000000000000013323 ) ) ;
#10291=CARTESIAN_POINT ( 'NONE',  ( -61.56765823437498142, 11.86979166632526805, 0.7511620957034663704 ) ) ;
#10294=CARTESIAN_POINT ( 'NONE',  ( -60.99999999999998579, 12.97916666666666607, 2.077350269189628840 ) ) ;
#10295=VERTEX_POINT ( 'NONE', #7931 ) ;
#10296=EDGE_CURVE ( 'NONE', #1159, #5429, #7374, .T. ) ;
#10297=CARTESIAN_POINT ( 'NONE',  ( -61.28647452029539267, 16.00000000000000000, 0.7993707187018740390 ) ) ;
#10298=CARTESIAN_POINT ( 'NONE',  ( -62.86468353124998032, 12.99479166632526805, 1.000774730468978246 ) ) ;
#10300=CARTESIAN_POINT ( 'NONE',  ( -60.99999999999998579, 11.00000000000000000, 1.500000000000002220 ) ) ;
#10301=CARTESIAN_POINT ( 'NONE',  ( -60.99999999999998579, 9.739583332650536107, 0.9226497308103762673 ) ) ;
#10303=VERTEX_POINT ( 'NONE', #9416 ) ;
#10304=( BOUNDED_CURVE ( )  B_SPLINE_CURVE ( 2, ( #4858, #5530, #647, #8985, #8932, #486, #8207, #1325, #598 ),
 .UNSPECIFIED., .F., .T. ) 
 B_SPLINE_CURVE_WITH_KNOTS ( ( 3, 2, 2, 2, 3 ),
 ( 0.6328125000000000000, 0.6354166666666666297, 0.6406250000000000000, 0.6458333333333333703, 0.6484375000000000000 ),
 .UNSPECIFIED. ) 
 CURVE ( )  GEOMETRIC_REPRESENTATION_ITEM ( )  RATIONAL_B_SPLINE_CURVE ( ( 0.9330127018922194093, 0.9330127018922194093, 1.000000000000000000, 0.8660254037844387076, 1.000000000000000000, 0.8660254037844387076, 1.000000000000000000, 0.9330127018922194093, 0.9330127018922194093 ) ) 
 REPRESENTATION_ITEM ( '' )  );
#10306=CARTESIAN_POINT ( 'NONE',  ( -60.99999999999998579, 9.947916665983870033, 2.077350269189628840 ) ) ;
#10307=CARTESIAN_POINT ( 'NONE',  ( -61.56765823437498142, 11.61979166632526805, 0.7511620957034663704 ) ) ;
#10311=CARTESIAN_POINT ( 'NONE',  ( -61.13531646874998415, 8.869791666325268054, 1.999225269531026417 ) ) ;
#10313=CARTESIAN_POINT ( 'NONE',  ( -61.56765823437498852, 14.59895833299193413, 2.248837904296538515 ) ) ;
#10314=CARTESIAN_POINT ( 'NONE',  ( -62.26794919243111082, 12.79241454900183150, 0.5000000000000013323 ) ) ;
#10316=VECTOR ( 'NONE', #1353, 1000.000000000000000 ) ;
#10320=CARTESIAN_POINT ( 'NONE',  ( -61.99999999999998579, 10.93750000000000000, 2.500000000000002665 ) ) ;
#10321=CARTESIAN_POINT ( 'NONE',  ( -61.49999999999998579, 8.291666666666666075, 0.6339745962155628467 ) ) ;
#10322=CARTESIAN_POINT ( 'NONE',  ( -62.26794919243112503, 8.792414549001835056, 0.5000000000000022204 ) ) ;
#10323=CARTESIAN_POINT ( 'NONE',  ( -60.99999999999998579, 12.44791666598386826, 2.077350269189628840 ) ) ;
#10325=FACE_OUTER_BOUND ( 'NONE', #757, .T. ) ;
#10326=AXIS2_PLACEMENT_3D ( 'NONE', #363, #3919, #3976 ) ;
#10327=CARTESIAN_POINT ( 'NONE',  ( -62.43234176562499016, 14.30729166632526983, 2.248837904296538071 ) ) ;
#10328=VECTOR ( 'NONE', #2813, 1000.000000000000000 ) ;
#10329=CARTESIAN_POINT ( 'NONE',  ( -61.13531646874998415, 8.578124999658601979, 1.500000000000002220 ) ) ;
#10332=CARTESIAN_POINT ( 'NONE',  ( -62.86468353124998742, 11.03645833299193413, 1.999225269531025972 ) ) ;
#10336=EDGE_CURVE ( 'NONE', #2581, #2979, #8933, .T. ) ;
#10338=( BOUNDED_CURVE ( )  B_SPLINE_CURVE ( 2, ( #8731, #3611, #7956, #10560, #1171, #2957, #2066, #6342, #10386 ),
 .UNSPECIFIED., .F., .F. ) 
 B_SPLINE_CURVE_WITH_KNOTS ( ( 3, 2, 2, 2, 3 ),
 ( 0.4609375000000000000, 0.4635416666666666852, 0.4687500000000000000, 0.4739583333333333148, 0.4765625000000000000 ),
 .UNSPECIFIED. ) 
 CURVE ( )  GEOMETRIC_REPRESENTATION_ITEM ( )  RATIONAL_B_SPLINE_CURVE ( ( 0.9330127018922194093, 0.9330127018922194093, 1.000000000000000000, 0.8660254037844387076, 1.000000000000000000, 0.8660254037844387076, 1.000000000000000000, 0.9330127018922194093, 0.9330127018922194093 ) ) 
 REPRESENTATION_ITEM ( '' )  );
#10340=LINE ( 'NONE', #9506, #1103 ) ;
#10341=CARTESIAN_POINT ( 'NONE',  ( -62.43234176562499016, 12.74479166632526805, 2.248837904296538071 ) ) ;
#10342=CARTESIAN_POINT ( 'NONE',  ( -62.86468353124999453, 8.223958332991934128, 1.999225269531025750 ) ) ;
#10343=CARTESIAN_POINT ( 'NONE',  ( -61.73205080756886076, 9.667414549001833279, 2.500000000000000000 ) ) ;
#10345=CARTESIAN_POINT ( 'NONE',  ( -60.99999999999998579, 15.22916666666666607, 2.077350269189628840 ) ) ;
#10346=CARTESIAN_POINT ( 'NONE',  ( -61.13531646874997705, 9.661458332991934128, 1.000774730468978468 ) ) ;
#10347=CARTESIAN_POINT ( 'NONE',  ( -61.13531646874998415, 15.09895833299193413, 1.000774730468978468 ) ) ;
#10349=CARTESIAN_POINT ( 'NONE',  ( -60.99999999999998579, 13.23958333265053611, 0.9226497308103762673 ) ) ;
#10353=CARTESIAN_POINT ( 'NONE',  ( -61.56765823437498142, 11.11979166632526805, 0.7511620957034663704 ) ) ;
#10355=CARTESIAN_POINT ( 'NONE',  ( -61.73205080756886076, 13.05133545031537068, 0.5000000000000014433 ) ) ;
#10357=CARTESIAN_POINT ( 'NONE',  ( -60.99999999999998579, 11.27083333333333393, 0.9226497308103762673 ) ) ;
#10358=EDGE_CURVE ( 'NONE', #2581, #6912, #8818, .T. ) ;
#10359=LINE ( 'NONE', #6141, #2526 ) ;
#10360=CARTESIAN_POINT ( 'NONE',  ( -61.13531646874998415, 14.39062499965860020, 1.500000000000002220 ) ) ;
#10361=CARTESIAN_POINT ( 'NONE',  ( -60.99999999999998579, 10.97916666666666607, 2.077350269189628840 ) ) ;
#10362=CARTESIAN_POINT ( 'NONE',  ( -60.99999999999998579, 9.489583332650537884, 0.9226497308103762673 ) ) ;
#10365=CARTESIAN_POINT ( 'NONE',  ( -60.99999999999998579, 13.50000000000000000, 1.500000000000002220 ) ) ;
#10366=CARTESIAN_POINT ( 'NONE',  ( -62.99999999999998579, 13.35416666666666785, 0.9226497308103756012 ) ) ;
#10367=CARTESIAN_POINT ( 'NONE',  ( -61.13531646874998415, 10.84895833299193590, 1.000774730468978468 ) ) ;
#10370=CARTESIAN_POINT ( 'NONE',  ( -61.13531646874998415, 10.41145833299193413, 1.000774730468978468 ) ) ;
#10371=DIRECTION ( 'NONE',  ( 0.000000000000000000, 0.000000000000000000, 1.000000000000000000 ) ) ;
#10372=CARTESIAN_POINT ( 'NONE',  ( -61.13531646874998415, 15.11979166632526628, 1.999225269531026417 ) ) ;
#10373=CARTESIAN_POINT ( 'NONE',  ( -61.99999999999998579, 16.00000000000000000, 2.500000000000000444 ) ) ;
#10374=ORIENTED_EDGE ( 'NONE', *, *, #602, .T. ) ;
#10375=CARTESIAN_POINT ( 'NONE',  ( -62.99999999999998579, 9.354166666666666075, 0.9226497308103756012 ) ) ;
#10379=CARTESIAN_POINT ( 'NONE',  ( -61.49999999999998579, 12.67708333265053611, 2.366025403784441927 ) ) ;
#10380=CARTESIAN_POINT ( 'NONE',  ( -60.99999999999998579, 8.270833333333332149, 0.9226497308103762673 ) ) ;
#10382=CARTESIAN_POINT ( 'NONE',  ( -61.99999999999998579, 9.156249999317203958, 2.500000000000002665 ) ) ;
#10383=CARTESIAN_POINT ( 'NONE',  ( -61.49999999999998579, 10.67708333265053611, 2.366025403784441927 ) ) ;
#10384=CARTESIAN_POINT ( 'NONE',  ( -61.13531646874997705, 13.91145833299193413, 1.000774730468978468 ) ) ;
#10385=CARTESIAN_POINT ( 'NONE',  ( -61.13531646874998415, 8.328124999658601979, 1.500000000000002220 ) ) ;
#10386=CARTESIAN_POINT ( 'NONE',  ( -61.99999999999998579, 12.03124999931720041, 0.5000000000000013323 ) ) ;
#10388=CARTESIAN_POINT ( 'NONE',  ( -62.43234176562499016, 10.05729166632526805, 2.248837904296538071 ) ) ;
#10389=CARTESIAN_POINT ( 'NONE',  ( -61.99999999999998579, 15.65624999931720218, 2.500000000000002665 ) ) ;
#10393=CARTESIAN_POINT ( 'NONE',  ( -61.73205080756886076, 15.69866454968462932, 2.500000000000003109 ) ) ;
#10394=CARTESIAN_POINT ( 'NONE',  ( -61.13531646874998415, 12.30729166632526628, 1.999225269531026417 ) ) ;
#10395=CARTESIAN_POINT ( 'NONE',  ( -61.13531646874997705, 9.348958332991937681, 1.000774730468978468 ) ) ;
#10398=CARTESIAN_POINT ( 'NONE',  ( -61.99999999999998579, 16.00000000000000000, 1.500000000000002220 ) ) ;
#10399=CARTESIAN_POINT ( 'NONE',  ( -61.56765823437498852, 9.598958332991934128, 2.248837904296538515 ) ) ;
#10401=CARTESIAN_POINT ( 'NONE',  ( -61.99999999999998579, 15.89062499965860198, 0.5015494609379544944 ) ) ;
#10402=CARTESIAN_POINT ( 'NONE',  ( -60.99999999999998579, 14.23958333265053611, 0.9226497308103762673 ) ) ;
#10403=CARTESIAN_POINT ( 'NONE',  ( -61.99999999999998579, 14.56249999999999822, 0.5000000000000013323 ) ) ;
#10404=EDGE_LOOP ( 'NONE', ( #8286, #4756, #1197, #5674 ) ) ;
#10406=CARTESIAN_POINT ( 'NONE',  ( -62.99999999999998579, 11.60416666666666785, 0.9226497308103756012 ) ) ;
#10407=CARTESIAN_POINT ( 'NONE',  ( -62.86468353124999453, 10.95312499965860020, 1.500000000000002220 ) ) ;
#10408=CARTESIAN_POINT ( 'NONE',  ( -61.13531646874998415, 8.828124999658601979, 1.500000000000002220 ) ) ;
#10411=CARTESIAN_POINT ( 'NONE',  ( -62.99999999999998579, 11.37500000000000000, 1.500000000000001998 ) ) ;
#10413=CARTESIAN_POINT ( 'NONE',  ( -62.86468353124998742, 14.28645833299193413, 1.999225269531025972 ) ) ;
#10415=CARTESIAN_POINT ( 'NONE',  ( -60.99999999999998579, 9.989583332650534331, 0.9226497308103762673 ) ) ;
#10416=ORIENTED_EDGE ( 'NONE', *, *, #7522, .F. ) ;
#10417=CARTESIAN_POINT ( 'NONE',  ( -60.99999999999998579, 13.97916666666666785, 2.077350269189628840 ) ) ;
#10418=EDGE_CURVE ( 'NONE', #10259, #6385, #4290, .T. ) ;
#10420=CARTESIAN_POINT ( 'NONE',  ( -61.56765823437498852, 11.03645833299193590, 2.248837904296538515 ) ) ;
#10421=CARTESIAN_POINT ( 'NONE',  ( -60.99999999999998579, 16.00000000000000000, 1.500000000000002220 ) ) ;
#10422=ADVANCED_FACE ( 'NONE', ( #9589 ), #6928, .T. ) ;
#10423=ORIENTED_EDGE ( 'NONE', *, *, #3265, .F. ) ;
#10424=AXIS2_PLACEMENT_3D ( 'NONE', #5408, #429, #4521 ) ;
#10425=CARTESIAN_POINT ( 'NONE',  ( -61.13531646874998415, 10.64062499965860198, 1.500000000000002220 ) ) ;
#10427=CARTESIAN_POINT ( 'NONE',  ( -62.86468353124998742, 14.03645833299193590, 1.999225269531025972 ) ) ;
#10429=ORIENTED_EDGE ( 'NONE', *, *, #9084, .F. ) ;
#10430=LINE ( 'NONE', #6223, #6575 ) ;
#10435=CARTESIAN_POINT ( 'NONE',  ( -61.49999999999998579, 9.041666666666666075, 0.6339745962155628467 ) ) ;
#10438=CARTESIAN_POINT ( 'NONE',  ( -62.49999999999998579, 8.916666666666666075, 2.366025403784441483 ) ) ;
#10439=CARTESIAN_POINT ( 'NONE',  ( -61.56765823437498142, 14.43229166632526983, 0.7511620957034663704 ) ) ;
#10442=CARTESIAN_POINT ( 'NONE',  ( -61.13531646874998415, 9.557291666325269830, 1.999225269531026417 ) ) ;
#10445=CARTESIAN_POINT ( 'NONE',  ( -61.13531646874998415, 9.890624999658601979, 1.500000000000002220 ) ) ;
#10447=CARTESIAN_POINT ( 'NONE',  ( -61.99999999999998579, 13.56249999999999822, 0.5000000000000013323 ) ) ;
#10448=ORIENTED_EDGE ( 'NONE', *, *, #3988, .T. ) ;
#10449=CARTESIAN_POINT ( 'NONE',  ( -61.99999999999998579, 14.06250000000000000, 0.5000000000000013323 ) ) ;
#10450=CARTESIAN_POINT ( 'NONE',  ( -60.99999999999998579, 15.25000000000000000, 1.500000000000002220 ) ) ;
#10452=CARTESIAN_POINT ( 'NONE',  ( -61.73205080756886076, 15.80133545031536713, 0.5000000000000014433 ) ) ;
#10453=CARTESIAN_POINT ( 'NONE',  ( -61.13531646874998415, 12.80729166632526805, 1.999225269531026417 ) ) ;
#10454=CARTESIAN_POINT ( 'NONE',  ( -61.99999999999999289, 8.390624999658601979, 0.5015494609379544944 ) ) ;
#10455=DIRECTION ( 'NONE',  ( 0.000000000000000000, 1.000000000000000000, 0.000000000000000000 ) ) ;
#10456=ORIENTED_EDGE ( 'NONE', *, *, #5195, .F. ) ;
#10457=CARTESIAN_POINT ( 'NONE',  ( -60.99999999999998579, 15.77083333333333215, 0.9226497308103762673 ) ) ;
#10458=CARTESIAN_POINT ( 'NONE',  ( -61.56765823437498142, 9.432291666325268054, 0.7511620957034663704 ) ) ;
#10460=CARTESIAN_POINT ( 'NONE',  ( -61.13531646874998415, 15.59895833299193590, 1.000774730468978468 ) ) ;
#10461=VECTOR ( 'NONE', #4657, 1000.000000000000000 ) ;
#10462=CARTESIAN_POINT ( 'NONE',  ( -62.99999999999998579, 14.61458333265053611, 2.077350269189627952 ) ) ;
#10467=CARTESIAN_POINT ( 'NONE',  ( -62.86468353124999453, 12.47395833299193413, 1.999225269531025750 ) ) ;
#10468=CARTESIAN_POINT ( 'NONE',  ( -62.86468353124998032, 8.932291666325268054, 1.000774730468978246 ) ) ;
#10469=AXIS2_PLACEMENT_3D ( 'NONE', #8950, #4711, #504 ) ;
#10472=CARTESIAN_POINT ( 'NONE',  ( -62.49999999999998579, 12.08333333333333393, 0.6339745962155627357 ) ) ;
#10473=CARTESIAN_POINT ( 'NONE',  ( -61.99999999999998579, 15.93749999999999645, 2.500000000000002665 ) ) ;
#10474=CARTESIAN_POINT ( 'NONE',  ( -61.56765823437498852, 14.59895833299193413, 2.248837904296538515 ) ) ;
#10475=( BOUNDED_CURVE ( )  B_SPLINE_CURVE ( 2, ( #7039, #9419, #3699, #10417, #9654, #1926, #1086, #143, #9477 ),
 .UNSPECIFIED., .F., .T. ) 
 B_SPLINE_CURVE_WITH_KNOTS ( ( 3, 2, 2, 2, 3 ),
 ( 0.7421875000000000000, 0.7447916666666666297, 0.7500000000000000000, 0.7552083333333333703, 0.7578125000000000000 ),
 .UNSPECIFIED. ) 
 CURVE ( )  GEOMETRIC_REPRESENTATION_ITEM ( )  RATIONAL_B_SPLINE_CURVE ( ( 0.9330127018922194093, 0.9330127018922194093, 1.000000000000000000, 0.8660254037844387076, 1.000000000000000000, 0.8660254037844387076, 1.000000000000000000, 0.9330127018922194093, 0.9330127018922194093 ) ) 
 REPRESENTATION_ITEM ( '' )  );
#10476=EDGE_CURVE ( 'NONE', #2070, #10833, #1611, .T. ) ;
#10478=CARTESIAN_POINT ( 'NONE',  ( -60.99999999999998579, 11.02083333333333393, 0.9226497308103762673 ) ) ;
#10479=CARTESIAN_POINT ( 'NONE',  ( -61.49999999999998579, 10.76041666598386826, 0.6339745962155628467 ) ) ;
#10481=CARTESIAN_POINT ( 'NONE',  ( -60.99999999999998579, 13.47916666666666785, 2.077350269189628840 ) ) ;
#10482=CARTESIAN_POINT ( 'NONE',  ( -62.99999999999998579, 15.32291666598387003, 0.9226497308103756012 ) ) ;
#10484=CARTESIAN_POINT ( 'NONE',  ( -62.86468353124998032, 12.93229166632526805, 1.000774730468978246 ) ) ;
#10487=CARTESIAN_POINT ( 'NONE',  ( -62.86468353124998032, 10.74479166632526628, 1.000774730468978246 ) ) ;
#10488=CARTESIAN_POINT ( 'NONE',  ( -61.99999999999998579, 15.40624999931720218, 2.500000000000002665 ) ) ;
#10489=CARTESIAN_POINT ( 'NONE',  ( -61.13531646874998415, 14.41145833299193413, 1.000774730468978468 ) ) ;
#10491=EDGE_LOOP ( 'NONE', ( #8710, #2697, #7991, #6694 ) ) ;
#10492=DIRECTION ( 'NONE',  ( -0.000000000000000000, -1.000000000000000000, -0.000000000000000000 ) ) ;
#10493=AXIS2_PLACEMENT_3D ( 'NONE', #10572, #2914, #3674 ) ;
#10494=VERTEX_POINT ( 'NONE', #3228 ) ;
#10496=CARTESIAN_POINT ( 'NONE',  ( -62.86468353124998032, 15.93229166632526805, 1.000774730468978246 ) ) ;
#10497=CARTESIAN_POINT ( 'NONE',  ( -62.49999999999998579, 9.552083332650536107, 0.6339745962155627357 ) ) ;
#10501=CARTESIAN_POINT ( 'NONE',  ( -62.86468353124999453, 14.76562499965860020, 1.500000000000002220 ) ) ;
#10502=CARTESIAN_POINT ( 'NONE',  ( -61.99999999999998579, 10.39062499965860020, 0.5015494609379544944 ) ) ;
#10506=CARTESIAN_POINT ( 'NONE',  ( -61.99999999999998579, 10.32812499965860020, 2.498450539062049724 ) ) ;
#10507=ADVANCED_FACE ( 'NONE', ( #6373 ), #8879, .T. ) ;
#10509=VERTEX_POINT ( 'NONE', #8402 ) ;
#10510=CARTESIAN_POINT ( 'NONE',  ( -62.99999999999998579, 14.37499999999999822, 1.500000000000001998 ) ) ;
#10511=CYLINDRICAL_SURFACE ( 'NONE', #3420, 0.9999999999999981126 ) ;
#10512=ORIENTED_EDGE ( 'NONE', *, *, #7717, .F. ) ;
#10515=CARTESIAN_POINT ( 'NONE',  ( -61.99999999999998579, 11.89062499965860198, 0.5015494609379544944 ) ) ;
#10517=CARTESIAN_POINT ( 'NONE',  ( -62.43234176562498305, 9.661458332991934128, 0.7511620957034662593 ) ) ;
#10519=CARTESIAN_POINT ( 'NONE',  ( -61.99999999999998579, 8.531249999317203958, 0.5000000000000013323 ) ) ;
#10520=CARTESIAN_POINT ( 'NONE',  ( -61.13531646874997705, 10.61979166632526628, 1.999225269531026417 ) ) ;
#10521=CARTESIAN_POINT ( 'NONE',  ( -62.86468353124998742, 15.72395833299193768, 1.999225269531025972 ) ) ;
#10522=CARTESIAN_POINT ( 'NONE',  ( -61.99999999999998579, 15.15624999931720218, 2.654700538379254571 ) ) ;
#10523=CARTESIAN_POINT ( 'NONE',  ( -62.99999999999998579, 16.07291666598386826, 0.9226497308103756012 ) ) ;
#10526=ORIENTED_EDGE ( 'NONE', *, *, #3812, .F. ) ;
#10527=ADVANCED_FACE ( 'NONE', ( #6682 ), #6436, .T. ) ;
#10528=CARTESIAN_POINT ( 'NONE',  ( -61.99999999999999289, 13.01562499965860198, 2.498450539062049724 ) ) ;
#10529=CARTESIAN_POINT ( 'NONE',  ( -61.13531646874998415, 9.057291666325266277, 1.999225269531026417 ) ) ;
#10530=CARTESIAN_POINT ( 'NONE',  ( -61.99999999999998579, 16.00000000000000000, 2.500000000000000444 ) ) ;
#10531=ORIENTED_EDGE ( 'NONE', *, *, #7897, .F. ) ;
#10532=CARTESIAN_POINT ( 'NONE',  ( -62.99999999999998579, 11.87500000000000000, 1.500000000000001998 ) ) ;
#10535=CARTESIAN_POINT ( 'NONE',  ( -61.56765823437498852, 14.09895833299193413, 2.248837904296538515 ) ) ;
#10537=CARTESIAN_POINT ( 'NONE',  ( -62.49999999999998579, 10.38541666598387003, 2.366025403784441483 ) ) ;
#10539=CARTESIAN_POINT ( 'NONE',  ( -61.99999999999998579, 16.00000000000000000, 0.5000000000000041078 ) ) ;
#10542=CARTESIAN_POINT ( 'NONE',  ( -61.99999999999998579, 12.51562499965860198, 2.498450539062049724 ) ) ;
#10544=( BOUNDED_CURVE ( )  B_SPLINE_CURVE ( 2, ( #3128, #3550, #106, #4161, #2727, #2608, #5152, #6837, #6893 ),
 .UNSPECIFIED., .F., .F. ) 
 B_SPLINE_CURVE_WITH_KNOTS ( ( 3, 2, 2, 2, 3 ),
 ( 0.5078125000000000000, 0.5104166666666666297, 0.5156250000000000000, 0.5208333333333333703, 0.5234375000000000000 ),
 .UNSPECIFIED. ) 
 CURVE ( )  GEOMETRIC_REPRESENTATION_ITEM ( )  RATIONAL_B_SPLINE_CURVE ( ( 0.9330127018922194093, 0.9330127018922194093, 1.000000000000000000, 0.8660254037844387076, 1.000000000000000000, 0.8660254037844387076, 1.000000000000000000, 0.9330127018922194093, 0.9330127018922194093 ) ) 
 REPRESENTATION_ITEM ( '' )  );
#10545=ORIENTED_EDGE ( 'NONE', *, *, #7874, .T. ) ;
#10546=CARTESIAN_POINT ( 'NONE',  ( -61.56765823437498852, 9.598958332991934128, 2.248837904296538515 ) ) ;
#10549=CARTESIAN_POINT ( 'NONE',  ( -61.13531646874998415, 14.64062499965860020, 1.500000000000002220 ) ) ;
#10551=ORIENTED_EDGE ( 'NONE', *, *, #4352, .F. ) ;
#10555=CARTESIAN_POINT ( 'NONE',  ( -61.13531646874998415, 16.05729166632526983, 1.999225269531026417 ) ) ;
#10558=CARTESIAN_POINT ( 'NONE',  ( -60.99999999999998579, 10.69791666598386826, 2.077350269189628840 ) ) ;
#10559=CARTESIAN_POINT ( 'NONE',  ( -61.56765823437498142, 10.36979166632526983, 0.7511620957034663704 ) ) ;
#10560=CARTESIAN_POINT ( 'NONE',  ( -60.99999999999998579, 11.94791666598387359, 2.077350269189628840 ) ) ;
#10562=CARTESIAN_POINT ( 'NONE',  ( -62.86468353124998742, 10.03645833299193235, 1.999225269531025972 ) ) ;
#10563=DIRECTION ( 'NONE',  ( 0.000000000000000000, 1.000000000000000000, 0.000000000000000000 ) ) ;
#10569=CARTESIAN_POINT ( 'NONE',  ( -61.13531646874998415, 12.07812499965860198, 1.500000000000002220 ) ) ;
#10571=CARTESIAN_POINT ( 'NONE',  ( -61.99999999999999289, 10.76562499965860020, 2.498450539062049724 ) ) ;
#10572=CARTESIAN_POINT ( 'NONE',  ( -61.99999999999998579, 8.000000000000000000, 1.500000000000002220 ) ) ;
#10574=DIRECTION ( 'NONE',  ( 0.000000000000000000, 0.000000000000000000, -1.000000000000000000 ) ) ;
#10575=CARTESIAN_POINT ( 'NONE',  ( -62.86468353124999453, 10.76562499965860020, 1.500000000000002220 ) ) ;
#10577=CARTESIAN_POINT ( 'NONE',  ( -61.56765823437498142, 15.11979166632526805, 0.7511620957034663704 ) ) ;
#10578=CARTESIAN_POINT ( 'NONE',  ( -60.99999999999998579, 14.19791666598387003, 2.077350269189628840 ) ) ;
#10580=ORIENTED_EDGE ( 'NONE', *, *, #10652, .F. ) ;
#10581=DIRECTION ( 'NONE',  ( -0.000000000000000000, -1.000000000000000000, -0.000000000000000000 ) ) ;
#10583=CARTESIAN_POINT ( 'NONE',  ( -62.86468353124998032, 12.43229166632526805, 1.000774730468978024 ) ) ;
#10584=CARTESIAN_POINT ( 'NONE',  ( -61.13531646874998415, 8.098958332991934128, 1.000774730468978468 ) ) ;
#10587=CARTESIAN_POINT ( 'NONE',  ( -62.49999999999998579, 12.91666666666666607, 2.366025403784441483 ) ) ;
#10590=CARTESIAN_POINT ( 'NONE',  ( -60.99999999999998579, 9.968749999317202182, 1.500000000000002220 ) ) ;
#10592=CYLINDRICAL_SURFACE ( 'NONE', #2798, 0.9999999999999981126 ) ;
#10593=CARTESIAN_POINT ( 'NONE',  ( -61.99999999999998579, 13.14062499965860198, 0.5015494609379544944 ) ) ;
#10595=ORIENTED_EDGE ( 'NONE', *, *, #3784, .F. ) ;
#10596=CARTESIAN_POINT ( 'NONE',  ( -62.86468353124998742, 10.28645833299193590, 1.999225269531025972 ) ) ;
#10597=CARTESIAN_POINT ( 'NONE',  ( -61.73205080756886076, 12.27008544963257286, 0.5000000000000014433 ) ) ;
#10599=CARTESIAN_POINT ( 'NONE',  ( -61.56765823437498142, 15.43229166632526805, 0.7511620957034663704 ) ) ;
#10602=LINE ( 'NONE', #3654, #1060 ) ;
#10603=( BOUNDED_CURVE ( )  B_SPLINE_CURVE ( 2, ( #6939, #10314, #2600, #10150, #876, #5935, #6721, #9275, #4255 ),
 .UNSPECIFIED., .F., .T. ) 
 B_SPLINE_CURVE_WITH_KNOTS ( ( 3, 2, 2, 2, 3 ),
 ( 0.5703125000000000000, 0.5729166666666666297, 0.5781250000000000000, 0.5833333333333333703, 0.5859375000000000000 ),
 .UNSPECIFIED. ) 
 CURVE ( )  GEOMETRIC_REPRESENTATION_ITEM ( )  RATIONAL_B_SPLINE_CURVE ( ( 0.9330127018922194093, 0.9330127018922194093, 1.000000000000000000, 0.8660254037844387076, 1.000000000000000000, 0.8660254037844387076, 1.000000000000000000, 0.9330127018922194093, 0.9330127018922194093 ) ) 
 REPRESENTATION_ITEM ( '' )  );
#10606=CARTESIAN_POINT ( 'NONE',  ( -61.73205080756886787, 8.801335450315370679, 0.4999999999999967804 ) ) ;
#10607=CARTESIAN_POINT ( 'NONE',  ( -61.99999999999998579, 10.31250000000000178, 0.3452994616207497591 ) ) ;
#10608=CARTESIAN_POINT ( 'NONE',  ( -62.99999999999998579, 9.614583332650536107, 2.077350269189627952 ) ) ;
#10611=CARTESIAN_POINT ( 'NONE',  ( -61.56765823437498142, 9.619791666325268054, 0.7511620957034663704 ) ) ;
#10612=FACE_OUTER_BOUND ( 'NONE', #2949, .T. ) ;
#10614=CARTESIAN_POINT ( 'NONE',  ( -62.43234176562498305, 11.22395833299193590, 0.7511620957034662593 ) ) ;
#10616=ORIENTED_EDGE ( 'NONE', *, *, #3433, .T. ) ;
#10621=ORIENTED_EDGE ( 'NONE', *, *, #466, .F. ) ;
#10623=CARTESIAN_POINT ( 'NONE',  ( -61.99999999999998579, 13.76562499965860020, 2.498450539062049724 ) ) ;
#10624=AXIS2_PLACEMENT_3D ( 'NONE', #8904, #1502, #4878 ) ;
#10625=CARTESIAN_POINT ( 'NONE',  ( -62.86468353124998032, 9.932291666325268054, 1.000774730468978024 ) ) ;
#10627=ORIENTED_EDGE ( 'NONE', *, *, #9615, .F. ) ;
#10628=CARTESIAN_POINT ( 'NONE',  ( -61.13531646874997705, 11.66145833299193590, 1.000774730468978468 ) ) ;
#10629=VECTOR ( 'NONE', #5183, 1000.000000000000000 ) ;
#10631=CARTESIAN_POINT ( 'NONE',  ( -61.99999999999998579, 15.06249999999999822, 0.5000000000000013323 ) ) ;
#10632=CARTESIAN_POINT ( 'NONE',  ( -61.49999999999998579, 14.67708333265053611, 2.366025403784441927 ) ) ;
#10635=CARTESIAN_POINT ( 'NONE',  ( -61.49999999999998579, 15.17708333265053611, 2.366025403784441927 ) ) ;
#10637=VERTEX_POINT ( 'NONE', #8293 ) ;
#10639=CARTESIAN_POINT ( 'NONE',  ( -61.99999999999999289, 12.51562499965860198, 2.498450539062049724 ) ) ;
#10640=CARTESIAN_POINT ( 'NONE',  ( -61.56765823437498852, 9.036458332991935904, 2.248837904296538515 ) ) ;
#10643=CARTESIAN_POINT ( 'NONE',  ( -62.99999999999998579, 12.10416666666666430, 0.9226497308103756012 ) ) ;
#10644=CARTESIAN_POINT ( 'NONE',  ( -62.99999999999998579, 11.09374999931720218, 1.500000000000001998 ) ) ;
#10649=CARTESIAN_POINT ( 'NONE',  ( -60.99999999999998579, 10.98958333265053611, 0.9226497308103762673 ) ) ;
#10652=EDGE_CURVE ( 'NONE', #5305, #2384, #3956, .T. ) ;
#10653=CARTESIAN_POINT ( 'NONE',  ( -61.99999999999998579, 14.93749999999999822, 2.500000000000002665 ) ) ;
#10655=CARTESIAN_POINT ( 'NONE',  ( -61.13531646874998415, 12.57812499965860198, 1.500000000000002220 ) ) ;
#10659=ORIENTED_EDGE ( 'NONE', *, *, #801, .T. ) ;
#10660=CARTESIAN_POINT ( 'NONE',  ( -61.56765823437498142, 11.68229166632526805, 0.7511620957034663704 ) ) ;
#10667=CARTESIAN_POINT ( 'NONE',  ( -62.99999999999998579, 10.35416666666666785, 0.9226497308103756012 ) ) ;
#10670=CARTESIAN_POINT ( 'NONE',  ( -61.99999999999998579, 14.53124999931720041, 0.5000000000000013323 ) ) ;
#10671=DIRECTION ( 'NONE',  ( -0.000000000000000000, -1.000000000000000000, -0.000000000000000000 ) ) ;
#10672=CARTESIAN_POINT ( 'NONE',  ( -61.49999999999998579, 8.510416665983868256, 0.6339745962155628467 ) ) ;
#10673=CARTESIAN_POINT ( 'NONE',  ( -62.86468353124998032, 11.74479166632526628, 1.000774730468978246 ) ) ;
#10675=ORIENTED_EDGE ( 'NONE', *, *, #497, .F. ) ;
#10676=EDGE_CURVE ( 'NONE', #5429, #4238, #168, .T. ) ;
#10677=( BOUNDED_CURVE ( )  B_SPLINE_CURVE ( 2, ( #4075, #7476, #2461, #10022, #2405, #9246, #1633, #10342, #7072, #237, #1005, #8745, #9454, #9508, #8683, #10454, #2792, #6961, #1962, #3621, #1125, #7853, #7797, #1182, #181, #10280, #7742, #5164, #6910, #5220, #2685, #6181, #4507, #6011, #350, #9399, #4559, #3506, #8626, #290, #1793, #3562, #5274, #1851, #5330, #2856, #6122, #6068, #7910, #4386, #3673, #6242, #6851, #2739, #1903, #1064, #4450, #7016, #8573, #8800, #2623, #10395, #9570, #2022, #9628, #5394, #7968, #10221, #952, #4331, #121, #5512, #3853, #7242, #5448, #5678, #10517, #8191, #3075, #7300, #8245, #8915, #577, #8857, #3738, #3962, #9072, #9016, #6473, #10625, #9904, #2193, #6353, #8969, #10740, #1242, #9799, #1303, #2913, #6302, #7189, #3125, #468, #5571, #4625, #1461, #4679, #8087, #3022, #2968, #5621, #9854, #6522, #2241, #2294, #1360, #1409, #9740, #4838, #7134, #4786, #7351, #415, #9683, #2077, #8024, #10685, #3799, #4727, #10571, #2136, #6416, #8137, #525, #3910, #1749, #7029, #190, #10407, #906, #3520, #4235, #77, #9520, #1861, #7642, #10353, #8585, #5288, #9467, #10233, #6975, #7698, #7751, #6920, #8699, #1016, #5174, #3574, #5231, #2750, #6080, #6024, #2807, #9410, #8527, #5965, #3407, #5123, #3462, #4288, #4399, #6136, #27, #9581, #6814, #6194, #6860, #2638, #1915, #10182, #1803, #10291, #962, #1075, #4463, #4340, #131, #7868, #2694, #2579, #8636, #248, #7810, #3632, #5070, #8471, #857, #9353, #5585, #9755, #9643, #8811, #1193, #3687, #4573, #7088, #1138, #7981, #10583, #4520, #10467, #3921, #10639, #7923, #6430, #366, #8757, #3038, #6366, #8099, #5462, #10700, #3750, #3089, #2151, #303, #5523, #7148, #1257, #4637, #9697, #8980, #1372, #5407, #8870, #2868, #10528, #2928, #6257, #540, #9811, #1318, #8927, #6485, #6313, #2089, #1974, #2033, #8039, #428, #3813, #7203, #2981, #4691, #7311, #481, #3866, #7257, #2205, #4742, #8151, #5344, #5635, #2309, #2403, #10952, #3239, #4801, #3341, #6593, #8258, #641, #4073, #6645, #6690, #9086, #10066, #4020, #3294, #7474, #1475, #9244, #9867, #744, #1573, #793, #2459, #593, #5793, #9189, #8299, #1422, #7416, #5849, #10800, #10853, #8202, #3139, #3191, #6536, #4958, #689, #9972, #3977, #8358, #5009, #4851, #2255, #2355, #4128, #7523, #9030, #4172, #5691, #10020, #1630, #10905, #8411, #7572, #5743, #7366, #9137, #10750, #9920, #1526, #4900, #5904, #8458, #8681, #4383, #1685, #177, #5108, #2515, #7795, #119, #1849, #842, #67, #5162, #7850, #3503, #5059, #6907, #8514, #6009, #9397, #3449, #2737, #6120, #10171, #10219, #4224, #894, #2568, #7629, #5270, #2683, #2620, #4275, #235, #5954, #9341, #6744, #14, #6849, #1791, #8571, #6800, #950, #4329, #1062, #7738, #6066, #10278, #9452, #5218, #1901, #8624, #1733, #7684, #1002, #10116, #3560 ),
 .UNSPECIFIED., .F., .T. ) 
 B_SPLINE_CURVE_WITH_KNOTS ( ( 3, 2, 2, 2, 2, 2, 2, 2, 2, 2, 2, 2, 2, 2, 2, 2, 2, 2, 2, 2, 2, 2, 2, 2, 2, 2, 2, 2, 2, 2, 2, 2, 2, 2, 2, 2, 2, 2, 2, 2, 2, 2, 2, 2, 2, 2, 2, 2, 2, 2, 2, 2, 2, 2, 2, 2, 2, 2, 2, 2, 2, 2, 2, 2, 2, 2, 2, 2, 2, 2, 2, 2, 2, 2, 2, 2, 2, 2, 2, 2, 2, 2, 2, 2, 2, 2, 2, 2, 2, 2, 2, 2, 2, 2, 2, 2, 2, 2, 2, 2, 2, 2, 2, 2, 2, 2, 2, 2, 2, 2, 2, 2, 2, 2, 2, 2, 2, 2, 2, 2, 2, 2, 2, 2, 2, 2, 2, 2, 2, 2, 2, 2, 2, 2, 2, 2, 2, 2, 2, 2, 2, 2, 2, 2, 2, 2, 2, 2, 2, 2, 2, 2, 2, 2, 2, 2, 2, 2, 2, 2, 2, 2, 2, 2, 2, 2, 2, 2, 2, 2, 2, 2, 2, 2, 2, 2, 2, 2, 2, 2, 2, 2, 2, 2, 2, 2, 2, 2, 2, 2, 2, 2, 3 ),
 ( 0.000000000000000000, 0.005208333333333333044, 0.01041666666666666609, 0.01562500000000000000, 0.02083333333333333218, 0.02604166666666666782, 0.03125000000000000000, 0.03645833333333333565, 0.04166666666666666435, 0.04687500000000000000, 0.05208333333333333565, 0.05729166666666666435, 0.06250000000000000000, 0.06770833333333332871, 0.07291666666666667129, 0.07812500000000000000, 0.08333333333333332871, 0.08854166666666667129, 0.09375000000000000000, 0.09895833333333332871, 0.1041666666666666713, 0.1093750000000000000, 0.1145833333333333287, 0.1197916666666666713, 0.1250000000000000000, 0.1302083333333333426, 0.1354166666666666574, 0.1406250000000000000, 0.1458333333333333426, 0.1510416666666666574, 0.1562500000000000000, 0.1614583333333333426, 0.1666666666666666574, 0.1718750000000000000, 0.1770833333333333426, 0.1822916666666666574, 0.1875000000000000000, 0.1927083333333333426, 0.1979166666666666574, 0.2031250000000000000, 0.2083333333333333426, 0.2135416666666666574, 0.2187500000000000000, 0.2239583333333333426, 0.2291666666666666574, 0.2343750000000000000, 0.2395833333333333426, 0.2447916666666666574, 0.2500000000000000000, 0.2552083333333333148, 0.2604166666666666852, 0.2656250000000000000, 0.2708333333333333148, 0.2760416666666666852, 0.2812500000000000000, 0.2864583333333333148, 0.2916666666666666852, 0.2968750000000000000, 0.3020833333333333148, 0.3072916666666666852, 0.3125000000000000000, 0.3177083333333333148, 0.3229166666666666852, 0.3281250000000000000, 0.3333333333333333148, 0.3385416666666666852, 0.3437500000000000000, 0.3489583333333333148, 0.3541666666666666852, 0.3593750000000000000, 0.3645833333333333148, 0.3697916666666666852, 0.3750000000000000000, 0.3802083333333333148, 0.3854166666666666852, 0.3906250000000000000, 0.3958333333333333148, 0.4010416666666666852, 0.4062500000000000000, 0.4114583333333333148, 0.4166666666666666852, 0.4218750000000000000, 0.4270833333333333148, 0.4322916666666666852, 0.4375000000000000000, 0.4427083333333333148, 0.4479166666666666852, 0.4531250000000000000, 0.4583333333333333148, 0.4635416666666666852, 0.4687500000000000000, 0.4739583333333333148, 0.4791666666666666852, 0.4843750000000000000, 0.4895833333333333148, 0.4947916666666666852, 0.5000000000000000000, 0.5052083333333333703, 0.5104166666666666297, 0.5156250000000000000, 0.5208333333333333703, 0.5260416666666666297, 0.5312500000000000000, 0.5364583333333333703, 0.5416666666666666297, 0.5468750000000000000, 0.5520833333333333703, 0.5572916666666666297, 0.5625000000000000000, 0.5677083333333333703, 0.5729166666666666297, 0.5781250000000000000, 0.5833333333333333703, 0.5885416666666666297, 0.5937500000000000000, 0.5989583333333333703, 0.6041666666666666297, 0.6093750000000000000, 0.6145833333333333703, 0.6197916666666666297, 0.6250000000000000000, 0.6302083333333333703, 0.6354166666666666297, 0.6406250000000000000, 0.6458333333333333703, 0.6510416666666666297, 0.6562500000000000000, 0.6614583333333333703, 0.6666666666666666297, 0.6718750000000000000, 0.6770833333333333703, 0.6822916666666666297, 0.6875000000000000000, 0.6927083333333333703, 0.6979166666666666297, 0.7031250000000000000, 0.7083333333333333703, 0.7135416666666666297, 0.7187500000000000000, 0.7239583333333333703, 0.7291666666666666297, 0.7343750000000000000, 0.7395833333333333703, 0.7447916666666666297, 0.7500000000000000000, 0.7552083333333333703, 0.7604166666666666297, 0.7656250000000000000, 0.7708333333333333703, 0.7760416666666666297, 0.7812500000000000000, 0.7864583333333333703, 0.7916666666666666297, 0.7968750000000000000, 0.8020833333333333703, 0.8072916666666666297, 0.8125000000000000000, 0.8177083333333333703, 0.8229166666666666297, 0.8281250000000000000, 0.8333333333333333703, 0.8385416666666666297, 0.8437500000000000000, 0.8489583333333333703, 0.8541666666666666297, 0.8593750000000000000, 0.8645833333333333703, 0.8697916666666666297, 0.8750000000000000000, 0.8802083333333333703, 0.8854166666666666297, 0.8906250000000000000, 0.8958333333333333703, 0.9010416666666666297, 0.9062500000000000000, 0.9114583333333333703, 0.9166666666666666297, 0.9218750000000000000, 0.9270833333333333703, 0.9322916666666666297, 0.9375000000000000000, 0.9427083333333333703, 0.9479166666666666297, 0.9531250000000000000, 0.9583333333333333703, 0.9635416666666666297, 0.9687500000000000000, 0.9739583333333333703, 0.9791666666666666297, 0.9843750000000000000, 0.9895833333333333703, 0.9947916666666666297, 1.000000000000000000 ),
 .UNSPECIFIED. ) 
 CURVE ( )  GEOMETRIC_REPRESENTATION_ITEM ( )  RATIONAL_B_SPLINE_CURVE ( ( 1.000000000000000000, 0.8660254037844387076, 1.000000000000000000, 0.8660254037844387076, 1.000000000000000000, 0.8660254037844387076, 1.000000000000000000, 0.8660254037844387076, 1.000000000000000000, 0.8660254037844387076, 1.000000000000000000, 0.8660254037844387076, 1.000000000000000000, 0.8660254037844387076, 1.000000000000000000, 0.8660254037844387076, 1.000000000000000000, 0.8660254037844387076, 1.000000000000000000, 0.8660254037844387076, 1.000000000000000000, 0.8660254037844387076, 1.000000000000000000, 0.8660254037844387076, 1.000000000000000000, 0.8660254037844387076, 1.000000000000000000, 0.8660254037844387076, 1.000000000000000000, 0.8660254037844387076, 1.000000000000000000, 0.8660254037844387076, 1.000000000000000000, 0.8660254037844387076, 1.000000000000000000, 0.8660254037844387076, 1.000000000000000000, 0.8660254037844387076, 1.000000000000000000, 0.8660254037844387076, 1.000000000000000000, 0.8660254037844387076, 1.000000000000000000, 0.8660254037844387076, 1.000000000000000000, 0.8660254037844387076, 1.000000000000000000, 0.8660254037844387076, 1.000000000000000000, 0.8660254037844387076, 1.000000000000000000, 0.8660254037844387076, 1.000000000000000000, 0.8660254037844387076, 1.000000000000000000, 0.8660254037844387076, 1.000000000000000000, 0.8660254037844387076, 1.000000000000000000, 0.8660254037844387076, 1.000000000000000000, 0.8660254037844387076, 1.000000000000000000, 0.8660254037844387076, 1.000000000000000000, 0.8660254037844387076, 1.000000000000000000, 0.8660254037844387076, 1.000000000000000000, 0.8660254037844387076, 1.000000000000000000, 0.8660254037844387076, 1.000000000000000000, 0.8660254037844387076, 1.000000000000000000, 0.8660254037844387076, 1.000000000000000000, 0.8660254037844387076, 1.000000000000000000, 0.8660254037844387076, 1.000000000000000000, 0.8660254037844387076, 1.000000000000000000, 0.8660254037844387076, 1.000000000000000000, 0.8660254037844387076, 1.000000000000000000, 0.8660254037844387076, 1.000000000000000000, 0.8660254037844387076, 1.000000000000000000, 0.8660254037844387076, 1.000000000000000000, 0.8660254037844387076, 1.000000000000000000, 0.8660254037844387076, 1.000000000000000000, 0.8660254037844387076, 1.000000000000000000, 0.8660254037844387076, 1.000000000000000000, 0.8660254037844387076, 1.000000000000000000, 0.8660254037844387076, 1.000000000000000000, 0.8660254037844387076, 1.000000000000000000, 0.8660254037844387076, 1.000000000000000000, 0.8660254037844387076, 1.000000000000000000, 0.8660254037844387076, 1.000000000000000000, 0.8660254037844387076, 1.000000000000000000, 0.8660254037844387076, 1.000000000000000000, 0.8660254037844387076, 1.000000000000000000, 0.8660254037844387076, 1.000000000000000000, 0.8660254037844387076, 1.000000000000000000, 0.8660254037844387076, 1.000000000000000000, 0.8660254037844387076, 1.000000000000000000, 0.8660254037844387076, 1.000000000000000000, 0.8660254037844387076, 1.000000000000000000, 0.8660254037844387076, 1.000000000000000000, 0.8660254037844387076, 1.000000000000000000, 0.8660254037844387076, 1.000000000000000000, 0.8660254037844387076, 1.000000000000000000, 0.8660254037844387076, 1.000000000000000000, 0.8660254037844387076, 1.000000000000000000, 0.8660254037844387076, 1.000000000000000000, 0.8660254037844387076, 1.000000000000000000, 0.8660254037844387076, 1.000000000000000000, 0.8660254037844387076, 1.000000000000000000, 0.8660254037844387076, 1.000000000000000000, 0.8660254037844387076, 1.000000000000000000, 0.8660254037844387076, 1.000000000000000000, 0.8660254037844387076, 1.000000000000000000, 0.8660254037844387076, 1.000000000000000000, 0.8660254037844387076, 1.000000000000000000, 0.8660254037844387076, 1.000000000000000000, 0.8660254037844387076, 1.000000000000000000, 0.8660254037844387076, 1.000000000000000000, 0.8660254037844387076, 1.000000000000000000, 0.8660254037844387076, 1.000000000000000000, 0.8660254037844387076, 1.000000000000000000, 0.8660254037844387076, 1.000000000000000000, 0.8660254037844387076, 1.000000000000000000, 0.8660254037844387076, 1.000000000000000000, 0.8660254037844387076, 1.000000000000000000, 0.8660254037844387076, 1.000000000000000000, 0.8660254037844387076, 1.000000000000000000, 0.8660254037844387076, 1.000000000000000000, 0.8660254037844387076, 1.000000000000000000, 0.8660254037844387076, 1.000000000000000000, 0.8660254037844387076, 1.000000000000000000, 0.8660254037844387076, 1.000000000000000000, 0.8660254037844387076, 1.000000000000000000, 0.8660254037844387076, 1.000000000000000000, 0.8660254037844387076, 1.000000000000000000, 0.8660254037844387076, 1.000000000000000000, 0.8660254037844387076, 1.000000000000000000, 0.8660254037844387076, 1.000000000000000000, 0.8660254037844387076, 1.000000000000000000, 0.8660254037844387076, 1.000000000000000000, 0.8660254037844387076, 1.000000000000000000, 0.8660254037844387076, 1.000000000000000000, 0.8660254037844387076, 1.000000000000000000, 0.8660254037844387076, 1.000000000000000000, 0.8660254037844387076, 1.000000000000000000, 0.8660254037844387076, 1.000000000000000000, 0.8660254037844387076, 1.000000000000000000, 0.8660254037844387076, 1.000000000000000000, 0.8660254037844387076, 1.000000000000000000, 0.8660254037844387076, 1.000000000000000000, 0.8660254037844387076, 1.000000000000000000, 0.8660254037844387076, 1.000000000000000000, 0.8660254037844387076, 1.000000000000000000, 0.8660254037844387076, 1.000000000000000000, 0.8660254037844387076, 1.000000000000000000, 0.8660254037844387076, 1.000000000000000000, 0.8660254037844387076, 1.000000000000000000, 0.8660254037844387076, 1.000000000000000000, 0.8660254037844387076, 1.000000000000000000, 0.8660254037844387076, 1.000000000000000000, 0.8660254037844387076, 1.000000000000000000, 0.8660254037844387076, 1.000000000000000000, 0.8660254037844387076, 1.000000000000000000, 0.8660254037844387076, 1.000000000000000000, 0.8660254037844387076, 1.000000000000000000, 0.8660254037844387076, 1.000000000000000000, 0.8660254037844387076, 1.000000000000000000, 0.8660254037844387076, 1.000000000000000000, 0.8660254037844387076, 1.000000000000000000, 0.8660254037844387076, 1.000000000000000000, 0.8660254037844387076, 1.000000000000000000, 0.8660254037844387076, 1.000000000000000000, 0.8660254037844387076, 1.000000000000000000, 0.8660254037844387076, 1.000000000000000000, 0.8660254037844387076, 1.000000000000000000, 0.8660254037844387076, 1.000000000000000000, 0.8660254037844387076, 1.000000000000000000, 0.8660254037844387076, 1.000000000000000000, 0.8660254037844387076, 1.000000000000000000, 0.8660254037844387076, 1.000000000000000000, 0.8660254037844387076, 1.000000000000000000, 0.8660254037844387076, 1.000000000000000000, 0.8660254037844387076, 1.000000000000000000, 0.8660254037844387076, 1.000000000000000000, 0.8660254037844387076, 1.000000000000000000, 0.8660254037844387076, 1.000000000000000000, 0.8660254037844387076, 1.000000000000000000, 0.8660254037844387076, 1.000000000000000000, 0.8660254037844387076, 1.000000000000000000, 0.8660254037844387076, 1.000000000000000000, 0.8660254037844387076, 1.000000000000000000, 0.8660254037844387076, 1.000000000000000000, 0.8660254037844387076, 1.000000000000000000, 0.8660254037844387076, 1.000000000000000000, 0.8660254037844387076, 1.000000000000000000, 0.8660254037844387076, 1.000000000000000000, 0.8660254037844387076, 1.000000000000000000, 0.8660254037844387076, 1.000000000000000000, 0.8660254037844387076, 1.000000000000000000, 0.8660254037844387076, 1.000000000000000000, 0.8660254037844387076, 1.000000000000000000, 0.8660254037844387076, 1.000000000000000000, 0.8660254037844387076, 1.000000000000000000, 0.8660254037844387076, 1.000000000000000000, 0.8660254037844387076, 1.000000000000000000, 0.8660254037844387076, 1.000000000000000000, 0.8660254037844387076, 1.000000000000000000, 0.8660254037844387076, 1.000000000000000000, 0.8660254037844387076, 1.000000000000000000, 0.8660254037844387076, 1.000000000000000000, 0.8660254037844387076, 1.000000000000000000, 0.8660254037844387076, 1.000000000000000000, 0.8660254037844387076, 1.000000000000000000, 0.8660254037844387076, 1.000000000000000000, 0.8660254037844387076, 1.000000000000000000, 0.8660254037844387076, 1.000000000000000000, 0.8660254037844387076, 1.000000000000000000, 0.8660254037844387076, 1.000000000000000000, 0.8660254037844387076, 1.000000000000000000, 0.8660254037844387076, 1.000000000000000000, 0.8660254037844387076, 1.000000000000000000, 0.8660254037844387076, 1.000000000000000000, 0.8660254037844387076, 1.000000000000000000, 0.8660254037844387076, 1.000000000000000000, 0.8660254037844387076, 1.000000000000000000, 0.8660254037844387076, 1.000000000000000000 ) ) 
 REPRESENTATION_ITEM ( '' )  );
#10684=CARTESIAN_POINT ( 'NONE',  ( -61.13531646874998415, 13.30729166632526983, 1.999225269531026417 ) ) ;
#10685=CARTESIAN_POINT ( 'NONE',  ( -62.86468353124999453, 10.70312499965860020, 1.500000000000002220 ) ) ;
#10686=LINE ( 'NONE', #8858, #4757 ) ;
#10687=VERTEX_POINT ( 'NONE', #8450 ) ;
#10688=CARTESIAN_POINT ( 'NONE',  ( -61.99999999999998579, 16.00000000000000000, 0.5000000000000041078 ) ) ;
#10689=CARTESIAN_POINT ( 'NONE',  ( -61.99999999999999289, 11.32812499965860020, 2.498450539062049724 ) ) ;
#10693=CARTESIAN_POINT ( 'NONE',  ( -61.99999999999998579, 8.203124999658601979, 0.5015494609379544944 ) ) ;
#10694=DIRECTION ( 'NONE',  ( 0.000000000000000000, 0.000000000000000000, -1.000000000000000000 ) ) ;
#10696=CARTESIAN_POINT ( 'NONE',  ( -61.73205080756886076, 15.27008544963257108, 0.5000000000000014433 ) ) ;
#10698=AXIS2_PLACEMENT_3D ( 'NONE', #6293, #10563, #1294 ) ;
#10700=CARTESIAN_POINT ( 'NONE',  ( -62.86468353124999453, 12.70312499965860198, 1.500000000000002220 ) ) ;
#10701=CARTESIAN_POINT ( 'NONE',  ( -62.86468353124999453, 9.953124999658601979, 1.500000000000002220 ) ) ;
#10704=CARTESIAN_POINT ( 'NONE',  ( -62.99999999999998579, 14.10416666666666607, 0.9226497308103756012 ) ) ;
#10705=CARTESIAN_POINT ( 'NONE',  ( -61.99999999999998579, 16.00000000000000000, 1.500000000000002220 ) ) ;
#10707=UNCERTAINTY_MEASURE_WITH_UNIT (LENGTH_MEASURE( 1.000000000000000082E-05 ), #8264, 'distance_accuracy_value', 'NONE');
#10710=CARTESIAN_POINT ( 'NONE',  ( -62.99999999999998579, 12.59374999931720396, 1.500000000000001998 ) ) ;
#10712=VECTOR ( 'NONE', #9691, 1000.000000000000000 ) ;
#10713=CARTESIAN_POINT ( 'NONE',  ( -61.99999999999998579, 12.39062499965860198, 0.5015494609379544944 ) ) ;
#10714=ADVANCED_FACE ( 'NONE', ( #3553 ), #1783, .T. ) ;
#10715=CARTESIAN_POINT ( 'NONE',  ( -60.99999999999998579, 11.52083333333333393, 0.9226497308103762673 ) ) ;
#10716=ORIENTED_EDGE ( 'NONE', *, *, #10676, .T. ) ;
#10717=ADVANCED_FACE ( 'NONE', ( #7620 ), #9286, .T. ) ;
#10718=CARTESIAN_POINT ( 'NONE',  ( -61.56765823437498852, 11.09895833299193590, 2.248837904296538515 ) ) ;
#10721=CARTESIAN_POINT ( 'NONE',  ( -61.99999999999998579, 10.90624999931720218, 2.500000000000002665 ) ) ;
#10722=ORIENTED_EDGE ( 'NONE', *, *, #2597, .T. ) ;
#10723=CARTESIAN_POINT ( 'NONE',  ( -62.99999999999998579, 11.12500000000000000, 1.500000000000001998 ) ) ;
#10726=CARTESIAN_POINT ( 'NONE',  ( -62.99999999999998579, 10.39583333333333215, 2.077350269189627952 ) ) ;
#10727=CARTESIAN_POINT ( 'NONE',  ( -61.73205080756886076, 11.19866454968462754, 2.500000000000003109 ) ) ;
#10728=FACE_OUTER_BOUND ( 'NONE', #6832, .T. ) ;
#10729=CARTESIAN_POINT ( 'NONE',  ( -61.99999999999998579, 12.18749999999999822, 2.500000000000002665 ) ) ;
#10732=CARTESIAN_POINT ( 'NONE',  ( -62.86468353124998742, 11.78645833299193590, 1.999225269531025972 ) ) ;
#10734=VERTEX_POINT ( 'NONE', #6897 ) ;
#10737=ORIENTED_EDGE ( 'NONE', *, *, #8905, .T. ) ;
#10739=CARTESIAN_POINT ( 'NONE',  ( -61.13531646874998415, 13.34895833299193413, 1.000774730468978468 ) ) ;
#10740=CARTESIAN_POINT ( 'NONE',  ( -61.56765823437498852, 10.03645833299193413, 2.248837904296538515 ) ) ;
#10742=ORIENTED_EDGE ( 'NONE', *, *, #6052, .F. ) ;
#10743=CARTESIAN_POINT ( 'NONE',  ( -62.86468353124999453, 11.26562499965860020, 1.500000000000002220 ) ) ;
#10744=CARTESIAN_POINT ( 'NONE',  ( -62.86468353124999453, 16.01562499965860198, 1.500000000000002220 ) ) ;
#10745=CARTESIAN_POINT ( 'NONE',  ( -62.99999999999998579, 16.11458333265053255, 2.077350269189627952 ) ) ;
#10747=ORIENTED_EDGE ( 'NONE', *, *, #3784, .T. ) ;
#10750=CARTESIAN_POINT ( 'NONE',  ( -61.13531646874997705, 14.80729166632526805, 1.999225269531026417 ) ) ;
#10751=CARTESIAN_POINT ( 'NONE',  ( -62.43234176562499016, 9.744791666325268054, 2.248837904296538071 ) ) ;
#10754=CARTESIAN_POINT ( 'NONE',  ( -61.99999999999998579, 14.31250000000000000, 0.3452994616207497591 ) ) ;
#10755=CARTESIAN_POINT ( 'NONE',  ( -62.49999999999998579, 8.552083332650536107, 0.6339745962155627357 ) ) ;
#10756=CARTESIAN_POINT ( 'NONE',  ( -61.99999999999998579, 12.03124999931720218, 0.3452994616207497591 ) ) ;
#10757=CARTESIAN_POINT ( 'NONE',  ( -61.99999999999998579, 12.28124999931720041, 0.5000000000000013323 ) ) ;
#10758=CARTESIAN_POINT ( 'NONE',  ( -61.13531646874998415, 14.34895833299193413, 1.000774730468978468 ) ) ;
#10759=ADVANCED_FACE ( 'NONE', ( #7677 ), #9333, .T. ) ;
#10762=CARTESIAN_POINT ( 'NONE',  ( -61.13531646874998415, 12.16145833299193413, 1.000774730468978468 ) ) ;
#10764=CARTESIAN_POINT ( 'NONE',  ( -61.13531646874998415, 15.39062499965860020, 1.500000000000002220 ) ) ;
#10765=ORIENTED_EDGE ( 'NONE', *, *, #7061, .T. ) ;
#10766=FACE_OUTER_BOUND ( 'NONE', #3378, .T. ) ;
#10770=CARTESIAN_POINT ( 'NONE',  ( -60.99999999999998579, 9.270833333333333925, 0.9226497308103762673 ) ) ;
#10771=CARTESIAN_POINT ( 'NONE',  ( -62.99999999999998579, 12.85416666666666607, 0.9226497308103756012 ) ) ;
#10772=FACE_OUTER_BOUND ( 'NONE', #6361, .T. ) ;
#10773=CARTESIAN_POINT ( 'NONE',  ( -61.99999999999998579, 12.31249999999999822, 0.5000000000000013323 ) ) ;
#10775=CARTESIAN_POINT ( 'NONE',  ( -61.56765823437498852, 11.59895833299193590, 2.248837904296538515 ) ) ;
#10777=ORIENTED_EDGE ( 'NONE', *, *, #535, .F. ) ;
#10778=CARTESIAN_POINT ( 'NONE',  ( -60.99999999999998579, 9.197916665983870033, 2.077350269189628840 ) ) ;
#10780=ADVANCED_FACE ( 'NONE', ( #8562 ), #5100, .T. ) ;
#10782=CARTESIAN_POINT ( 'NONE',  ( -61.99999999999998579, 13.78124999931720218, 0.5000000000000013323 ) ) ;
#10783=EDGE_CURVE ( 'NONE', #9337, #1260, #3896, .T. ) ;
#10784=CARTESIAN_POINT ( 'NONE',  ( -61.13531646874998415, 13.82812499965860198, 1.500000000000002220 ) ) ;
#10786=CARTESIAN_POINT ( 'NONE',  ( -62.99999999999998579, 8.145833333333333925, 2.077350269189627952 ) ) ;
#10787=CARTESIAN_POINT ( 'NONE',  ( -62.49999999999998579, 8.302083332650536107, 0.6339745962155627357 ) ) ;
#10788=CARTESIAN_POINT ( 'NONE',  ( -62.43234176562499016, 11.05729166632526805, 2.248837904296538071 ) ) ;
#10790=CARTESIAN_POINT ( 'NONE',  ( -61.99999999999998579, 15.57812499965860198, 2.498450539062049724 ) ) ;
#10792=CARTESIAN_POINT ( 'NONE',  ( -61.99999999999998579, 13.53124999931720041, 0.5000000000000013323 ) ) ;
#10793=CARTESIAN_POINT ( 'NONE',  ( -62.99999999999998579, 15.34374999931720218, 1.500000000000001998 ) ) ;
#10796=ORIENTED_EDGE ( 'NONE', *, *, #646, .T. ) ;
#10798=CARTESIAN_POINT ( 'NONE',  ( -62.99999999999998579, 12.62500000000000000, 1.500000000000001998 ) ) ;
#10800=CARTESIAN_POINT ( 'NONE',  ( -62.86468353124999453, 14.22395833299193590, 1.999225269531025750 ) ) ;
#10801=CARTESIAN_POINT ( 'NONE',  ( -62.86468353124998742, 9.473958332991934128, 1.999225269531025972 ) ) ;
#10802=AXIS2_PLACEMENT_3D ( 'NONE', #9763, #5735, #4064 ) ;
#10805=CARTESIAN_POINT ( 'NONE',  ( -61.49999999999998579, 13.45833333333333215, 2.366025403784441927 ) ) ;
#10806=CARTESIAN_POINT ( 'NONE',  ( -62.99999999999998579, 8.572916665983868256, 0.9226497308103756012 ) ) ;
#10807=AXIS2_PLACEMENT_3D ( 'NONE', #7678, #3332, #6683 ) ;
#10808=CARTESIAN_POINT ( 'NONE',  ( -60.99999999999998579, 12.19791666598386826, 2.077350269189628840 ) ) ;
#10810=CARTESIAN_POINT ( 'NONE',  ( -61.56765823437498142, 14.11979166632526805, 0.7511620957034663704 ) ) ;
#10811=FACE_OUTER_BOUND ( 'NONE', #9856, .T. ) ;
#10816=CARTESIAN_POINT ( 'NONE',  ( -62.86468353124998032, 11.99479166632526805, 1.000774730468978246 ) ) ;
#10817=DIRECTION ( 'NONE',  ( -0.000000000000000000, -1.000000000000000000, -0.000000000000000000 ) ) ;
#10818=ADVANCED_FACE ( 'NONE', ( #6735 ), #5050, .T. ) ;
#10826=CARTESIAN_POINT ( 'NONE',  ( -62.99999999999998579, 9.625000000000000000, 1.500000000000001998 ) ) ;
#10827=CARTESIAN_POINT ( 'NONE',  ( -61.49999999999998579, 15.01041666598386826, 0.6339745962155628467 ) ) ;
#10828=CARTESIAN_POINT ( 'NONE',  ( -61.99999999999997868, 8.312499999999998224, 0.5000000000000013323 ) ) ;
#10829=( BOUNDED_SURFACE ( )  B_SPLINE_SURFACE ( 1, 2, ( 
 ( #7204, #10584, #9756, #9698, #4692, #1194, #7149, #2809, #1139, #7869, #3814, #2034, #7924, #6367, #2152, #5345, #5524, #5463, #1975, #9812, #6195, #8040, #4574, #3633, #8928, #3751, #304, #1319, #1258, #8100, #9582, #3688, #7030, #2206, #3867, #6314, #10408, #8758, #7982, #8700, #7090, #10468, #2869, #7258, #368, #6258, #10640, #10529, #8871, #4638, #3039, #6431, #1076, #4464, #10067, #9973, #1527, #3192, #3240, #5586, #7312, #8152, #1476, #4901, #2404, #2310, #9921, #10801, #9138, #8981, #7524, #10854, #541, #8360, #4743, #8300, #6646, #5794, #6487, #4852, #10751, #8259, #9868, #745, #4129, #2256, #9190, #4074, #7475, #690, #10701, #5636, #10021, #10906, #9087, #3922, #5692, #1574, #1423, #594, #6537, #4959, #3295, #642, #6691, #1373, #9031, #3090, #4802, #8203, #3978, #2356, #7367, #3140, #4022, #7417, #6594, #5744, #8459, #951, #7685, #4330, #8625, #9398, #3451, #1792, #1735, #2684, #68, #9245, #7630, #1686, #7740, #8572, #2569, #10220, #2621, #120, #4276, #4173, #9453, #7573, #3504, #5163, #5109, #2516, #3561, #15, #2460, #6908, #10279, #6850, #7796, #3393, #5906, #9296, #6067, #5219, #1850, #6010, #6801, #4384, #1004, #178, #5955, #9342, #6959, #5850, #1632, #5060, #843, #8515, #5010, #3342, #10173, #10953, #8412, #794, #6745, #10117, #4225, #895, #3798, #10515, #3737, #8086, #6179, #3620, #6352, #5272, #7188, #467, #10569, #7133, #2967, #289, #7015, #1902, #1961, #4558, #9738, #1063, #8682, #10394, #2912, #7966, #2791, #6300, #3851, #9682, #9569, #4448, #8799, #7909, #1124, #349, #2076, #2135, #5329, #8742, #7851, #5510, #5447, #8855, #10341, #4506, #2738, #10453, #3672, #413, #6121, #1241, #8914, #9507, #1302, #4678, #7070, #2855, #236, #6241, #9627, #2020, #5393, #1181, #4624, #8023, #5570, #4837, #5778, #9123, #8190, #10684, #2293, #10739, #4057, #8288, #671, #3124, #7350, #4885, #1510, #6579, #3074, #7299, #6521, #8244, #8135, #576, #1359, #7402, #2340, #523, #9172, #10623, #2191, #7458, #10784, #628, #4940, #6472, #3909, #3220, #8968, #10837, #8343, #6629, #4008, #10008, #3960, #9853, #9798, #2240, #1460, #2388, #4726, #5620, #9015, #3174, #9958, #1407, #5729, #728, #1559, #4785, #9903, #5676, #9071, #7241, #3021, #6415, #936, #779, #2499, #1615, #10262, #882, #8497, #4110, #4158, #7508, #4208, #5044, #5149, #1835, #6834, #4315, #10890, #7725, #6890, #9280, #1672, #2670, #10102, #6049, #3380, #5206, #8609, #10936, #6676, #2440, #1719, #9436, #5993, #8444, #7559, #10157, #7613, #103, #8553, #3488, #714, #829, #3327, #9381, #10205, #6783, #4261, #7669, #1776, #5940, #5832, #3281, #9230, #2605, #52, #2553, #6728, #10052, #9326, #4991, #8395, #5887, #5094, #3436, #1944, #1044, #7834, #10496, #3779, #8837, #5377, #6163, #2952, #10555, #2895 ),
 ( #331, #4543, #4604, #1887, #7002, #161, #5493, #2059, #6226, #3547, #5258, #5315, #988, #10380, #10321, #4433, #8008, #8726, #8662, #5431, #273, #218, #1108, #393, #6338, #6283, #6945, #4367, #8783, #7949, #9608, #9668, #7779, #2724, #6107, #7894, #3718, #1224, #4490, #3658, #2002, #7117, #9492, #9722, #7172, #3604, #2116, #2776, #9551, #7054, #10435, #2839, #1164, #3061, #564, #9784, #661, #7445, #2173, #1498, #7391, #10770, #1444, #3008, #5553, #9946, #4042, #1392, #452, #5606, #617, #4713, #3893, #9840, #9108, #4874, #9001, #3160, #10826, #1344, #4821, #6564, #3210, #8121, #2278, #3996, #2329, #6397, #9995, #4770, #8231, #7286, #5711, #3110, #8277, #6617, #2378, #9888, #8898, #8175, #1284, #6507, #4661, #8069, #5660, #3836, #3943, #7337, #8954, #509, #7227, #10607, #2227, #10667, #6458, #10726, #9059, #2755, #2489, #10091, #10980, #9471, #9161, #7872, #193, #717, #8704, #4927, #1865, #3577, #6140, #6666, #5033, #10926, #8432, #10042, #1079, #4467, #2427, #9526, #4404, #7814, #5236, #10879, #5818, #6979, #252, #9266, #8325, #5873, #8640, #1601, #766, #6714, #1919, #5292, #1659, #10357, #3635, #9217, #1020, #7033, #10411, #4981, #10142, #5767, #1545, #3268, #4098, #817, #7495, #4148, #8382, #3369, #7546, #3315, #4196, #6770, #7600, #2698, #6082, #8043, #9586, #3871, #3817, #9815, #10532, #1261, #7927, #6261, #1978, #8931, #3754, #2037, #4695, #5527, #10472, #10643, #7207, #7093, #3925, #307, #2155, #2932, #5348, #1323, #8874, #5411, #8103, #6371, #6434, #3691, #8815, #8761, #7315, #7262, #432, #1142, #2872, #7152, #2812, #1198, #4524, #9647, #2209, #6317, #4578, #3042, #2093, #7984, #9701, #5589, #8156, #485, #371, #6198, #10587, #9759, #2985, #8984, #5467, #4641, #1375, #4747, #545, #7529, #645, #10910, #3299, #7421, #1579, #2465, #3143, #3245, #4963, #9249, #6541, #4078, #5798, #9195, #8206, #799, #10805, #6650, #5695, #8364, #4905, #749, #5854, #10025, #695, #2408, #9978, #6695, #8305, #6490, #4133, #7479, #10070, #3195, #9142, #4805, #9925, #9871, #1636, #4025, #2313, #5014, #8416, #7370, #4177, #10858, #3981, #10704, #597, #3093, #6597, #2259, #5640, #5748, #9090, #9035, #1426, #10754, #1479, #4856, #8262, #2360, #1530, #1796, #10121, #848, #8519, #1067, #2573, #5910, #19, #184, #899, #8463, #8629, #6854, #7634, #4280, #3564, #1906, #9456, #2520, #7577, #954, #3509, #5167, #5223, #10958, #9300, #1690, #3455, #6913, #4389, #7690, #72, #8576, #123, #3347, #9512, #1854, #5065, #10345, #6749, #10282, #1007, #7801, #4229, #10224, #1740, #2626, #3397, #2742, #6126, #6805, #6964, #6071, #5277, #2687, #10177, #5959, #8686, #9347, #6015, #5114, #9402, #4333, #7745, #10457, #8027, #9572, #8747, #5515, #7245, #7971, #7019, #1185, #7192, #293, #2859 ) ),
 .UNSPECIFIED., .F., .F., .F. ) 
 B_SPLINE_SURFACE_WITH_KNOTS ( ( 2, 2 ),
 ( 3, 2, 2, 2, 2, 2, 2, 2, 2, 2, 2, 2, 2, 2, 2, 2, 2, 2, 2, 2, 2, 2, 2, 2, 2, 2, 2, 2, 2, 2, 2, 2, 2, 2, 2, 2, 2, 2, 2, 2, 2, 2, 2, 2, 2, 2, 2, 2, 2, 2, 2, 2, 2, 2, 2, 2, 2, 2, 2, 2, 2, 2, 2, 2, 2, 2, 2, 2, 2, 2, 2, 2, 2, 2, 2, 2, 2, 2, 2, 2, 2, 2, 2, 2, 2, 2, 2, 2, 2, 2, 2, 2, 2, 2, 2, 2, 2, 2, 2, 2, 2, 2, 2, 2, 2, 2, 2, 2, 2, 2, 2, 2, 2, 2, 2, 2, 2, 2, 2, 2, 2, 2, 2, 2, 2, 2, 2, 2, 2, 2, 2, 2, 2, 2, 2, 2, 2, 2, 2, 2, 2, 2, 2, 2, 2, 2, 2, 2, 2, 2, 2, 2, 2, 2, 2, 2, 2, 2, 2, 2, 2, 2, 2, 2, 2, 2, 2, 2, 2, 2, 2, 2, 2, 2, 2, 2, 2, 2, 2, 2, 2, 2, 2, 2, 2, 2, 2, 2, 2, 2, 2, 2, 3 ),
 ( 0.000000000000000000, 1.000000000000000000 ),
 ( 0.000000000000000000, 0.005208333333333333044, 0.01041666666666666609, 0.01562500000000000000, 0.02083333333333333218, 0.02604166666666666782, 0.03125000000000000000, 0.03645833333333333565, 0.04166666666666666435, 0.04687500000000000000, 0.05208333333333333565, 0.05729166666666666435, 0.06250000000000000000, 0.06770833333333332871, 0.07291666666666667129, 0.07812500000000000000, 0.08333333333333332871, 0.08854166666666667129, 0.09375000000000000000, 0.09895833333333332871, 0.1041666666666666713, 0.1093750000000000000, 0.1145833333333333287, 0.1197916666666666713, 0.1250000000000000000, 0.1302083333333333426, 0.1354166666666666574, 0.1406250000000000000, 0.1458333333333333426, 0.1510416666666666574, 0.1562500000000000000, 0.1614583333333333426, 0.1666666666666666574, 0.1718750000000000000, 0.1770833333333333426, 0.1822916666666666574, 0.1875000000000000000, 0.1927083333333333426, 0.1979166666666666574, 0.2031250000000000000, 0.2083333333333333426, 0.2135416666666666574, 0.2187500000000000000, 0.2239583333333333426, 0.2291666666666666574, 0.2343750000000000000, 0.2395833333333333426, 0.2447916666666666574, 0.2500000000000000000, 0.2552083333333333148, 0.2604166666666666852, 0.2656250000000000000, 0.2708333333333333148, 0.2760416666666666852, 0.2812500000000000000, 0.2864583333333333148, 0.2916666666666666852, 0.2968750000000000000, 0.3020833333333333148, 0.3072916666666666852, 0.3125000000000000000, 0.3177083333333333148, 0.3229166666666666852, 0.3281250000000000000, 0.3333333333333333148, 0.3385416666666666852, 0.3437500000000000000, 0.3489583333333333148, 0.3541666666666666852, 0.3593750000000000000, 0.3645833333333333148, 0.3697916666666666852, 0.3750000000000000000, 0.3802083333333333148, 0.3854166666666666852, 0.3906250000000000000, 0.3958333333333333148, 0.4010416666666666852, 0.4062500000000000000, 0.4114583333333333148, 0.4166666666666666852, 0.4218750000000000000, 0.4270833333333333148, 0.4322916666666666852, 0.4375000000000000000, 0.4427083333333333148, 0.4479166666666666852, 0.4531250000000000000, 0.4583333333333333148, 0.4635416666666666852, 0.4687500000000000000, 0.4739583333333333148, 0.4791666666666666852, 0.4843750000000000000, 0.4895833333333333148, 0.4947916666666666852, 0.5000000000000000000, 0.5052083333333333703, 0.5104166666666666297, 0.5156250000000000000, 0.5208333333333333703, 0.5260416666666666297, 0.5312500000000000000, 0.5364583333333333703, 0.5416666666666666297, 0.5468750000000000000, 0.5520833333333333703, 0.5572916666666666297, 0.5625000000000000000, 0.5677083333333333703, 0.5729166666666666297, 0.5781250000000000000, 0.5833333333333333703, 0.5885416666666666297, 0.5937500000000000000, 0.5989583333333333703, 0.6041666666666666297, 0.6093750000000000000, 0.6145833333333333703, 0.6197916666666666297, 0.6250000000000000000, 0.6302083333333333703, 0.6354166666666666297, 0.6406250000000000000, 0.6458333333333333703, 0.6510416666666666297, 0.6562500000000000000, 0.6614583333333333703, 0.6666666666666666297, 0.6718750000000000000, 0.6770833333333333703, 0.6822916666666666297, 0.6875000000000000000, 0.6927083333333333703, 0.6979166666666666297, 0.7031250000000000000, 0.7083333333333333703, 0.7135416666666666297, 0.7187500000000000000, 0.7239583333333333703, 0.7291666666666666297, 0.7343750000000000000, 0.7395833333333333703, 0.7447916666666666297, 0.7500000000000000000, 0.7552083333333333703, 0.7604166666666666297, 0.7656250000000000000, 0.7708333333333333703, 0.7760416666666666297, 0.7812500000000000000, 0.7864583333333333703, 0.7916666666666666297, 0.7968750000000000000, 0.8020833333333333703, 0.8072916666666666297, 0.8125000000000000000, 0.8177083333333333703, 0.8229166666666666297, 0.8281250000000000000, 0.8333333333333333703, 0.8385416666666666297, 0.8437500000000000000, 0.8489583333333333703, 0.8541666666666666297, 0.8593750000000000000, 0.8645833333333333703, 0.8697916666666666297, 0.8750000000000000000, 0.8802083333333333703, 0.8854166666666666297, 0.8906250000000000000, 0.8958333333333333703, 0.9010416666666666297, 0.9062500000000000000, 0.9114583333333333703, 0.9166666666666666297, 0.9218750000000000000, 0.9270833333333333703, 0.9322916666666666297, 0.9375000000000000000, 0.9427083333333333703, 0.9479166666666666297, 0.9531250000000000000, 0.9583333333333333703, 0.9635416666666666297, 0.9687500000000000000, 0.9739583333333333703, 0.9791666666666666297, 0.9843750000000000000, 0.9895833333333333703, 0.9947916666666666297, 1.000000000000000000 ),
 .UNSPECIFIED. ) 
 GEOMETRIC_REPRESENTATION_ITEM ( )  RATIONAL_B_SPLINE_SURFACE ( (
 ( 1.000000000000000000, 0.8660254037844387076, 1.000000000000000000, 0.8660254037844387076, 1.000000000000000000, 0.8660254037844387076, 1.000000000000000000, 0.8660254037844387076, 1.000000000000000000, 0.8660254037844387076, 1.000000000000000000, 0.8660254037844387076, 1.000000000000000000, 0.8660254037844387076, 1.000000000000000000, 0.8660254037844387076, 1.000000000000000000, 0.8660254037844387076, 1.000000000000000000, 0.8660254037844387076, 1.000000000000000000, 0.8660254037844387076, 1.000000000000000000, 0.8660254037844387076, 1.000000000000000000, 0.8660254037844387076, 1.000000000000000000, 0.8660254037844387076, 1.000000000000000000, 0.8660254037844387076, 1.000000000000000000, 0.8660254037844387076, 1.000000000000000000, 0.8660254037844387076, 1.000000000000000000, 0.8660254037844387076, 1.000000000000000000, 0.8660254037844387076, 1.000000000000000000, 0.8660254037844387076, 1.000000000000000000, 0.8660254037844387076, 1.000000000000000000, 0.8660254037844387076, 1.000000000000000000, 0.8660254037844387076, 1.000000000000000000, 0.8660254037844387076, 1.000000000000000000, 0.8660254037844387076, 1.000000000000000000, 0.8660254037844387076, 1.000000000000000000, 0.8660254037844387076, 1.000000000000000000, 0.8660254037844387076, 1.000000000000000000, 0.8660254037844387076, 1.000000000000000000, 0.8660254037844387076, 1.000000000000000000, 0.8660254037844387076, 1.000000000000000000, 0.8660254037844387076, 1.000000000000000000, 0.8660254037844387076, 1.000000000000000000, 0.8660254037844387076, 1.000000000000000000, 0.8660254037844387076, 1.000000000000000000, 0.8660254037844387076, 1.000000000000000000, 0.8660254037844387076, 1.000000000000000000, 0.8660254037844387076, 1.000000000000000000, 0.8660254037844387076, 1.000000000000000000, 0.8660254037844387076, 1.000000000000000000, 0.8660254037844387076, 1.000000000000000000, 0.8660254037844387076, 1.000000000000000000, 0.8660254037844387076, 1.000000000000000000, 0.8660254037844387076, 1.000000000000000000, 0.8660254037844387076, 1.000000000000000000, 0.8660254037844387076, 1.000000000000000000, 0.8660254037844387076, 1.000000000000000000, 0.8660254037844387076, 1.000000000000000000, 0.8660254037844387076, 1.000000000000000000, 0.8660254037844387076, 1.000000000000000000, 0.8660254037844387076, 1.000000000000000000, 0.8660254037844387076, 1.000000000000000000, 0.8660254037844387076, 1.000000000000000000, 0.8660254037844387076, 1.000000000000000000, 0.8660254037844387076, 1.000000000000000000, 0.8660254037844387076, 1.000000000000000000, 0.8660254037844387076, 1.000000000000000000, 0.8660254037844387076, 1.000000000000000000, 0.8660254037844387076, 1.000000000000000000, 0.8660254037844387076, 1.000000000000000000, 0.8660254037844387076, 1.000000000000000000, 0.8660254037844387076, 1.000000000000000000, 0.8660254037844387076, 1.000000000000000000, 0.8660254037844387076, 1.000000000000000000, 0.8660254037844387076, 1.000000000000000000, 0.8660254037844387076, 1.000000000000000000, 0.8660254037844387076, 1.000000000000000000, 0.8660254037844387076, 1.000000000000000000, 0.8660254037844387076, 1.000000000000000000, 0.8660254037844387076, 1.000000000000000000, 0.8660254037844387076, 1.000000000000000000, 0.8660254037844387076, 1.000000000000000000, 0.8660254037844387076, 1.000000000000000000, 0.8660254037844387076, 1.000000000000000000, 0.8660254037844387076, 1.000000000000000000, 0.8660254037844387076, 1.000000000000000000, 0.8660254037844387076, 1.000000000000000000, 0.8660254037844387076, 1.000000000000000000, 0.8660254037844387076, 1.000000000000000000, 0.8660254037844387076, 1.000000000000000000, 0.8660254037844387076, 1.000000000000000000, 0.8660254037844387076, 1.000000000000000000, 0.8660254037844387076, 1.000000000000000000, 0.8660254037844387076, 1.000000000000000000, 0.8660254037844387076, 1.000000000000000000, 0.8660254037844387076, 1.000000000000000000, 0.8660254037844387076, 1.000000000000000000, 0.8660254037844387076, 1.000000000000000000, 0.8660254037844387076, 1.000000000000000000, 0.8660254037844387076, 1.000000000000000000, 0.8660254037844387076, 1.000000000000000000, 0.8660254037844387076, 1.000000000000000000, 0.8660254037844387076, 1.000000000000000000, 0.8660254037844387076, 1.000000000000000000, 0.8660254037844387076, 1.000000000000000000, 0.8660254037844387076, 1.000000000000000000, 0.8660254037844387076, 1.000000000000000000, 0.8660254037844387076, 1.000000000000000000, 0.8660254037844387076, 1.000000000000000000, 0.8660254037844387076, 1.000000000000000000, 0.8660254037844387076, 1.000000000000000000, 0.8660254037844387076, 1.000000000000000000, 0.8660254037844387076, 1.000000000000000000, 0.8660254037844387076, 1.000000000000000000, 0.8660254037844387076, 1.000000000000000000, 0.8660254037844387076, 1.000000000000000000, 0.8660254037844387076, 1.000000000000000000, 0.8660254037844387076, 1.000000000000000000, 0.8660254037844387076, 1.000000000000000000, 0.8660254037844387076, 1.000000000000000000, 0.8660254037844387076, 1.000000000000000000, 0.8660254037844387076, 1.000000000000000000, 0.8660254037844387076, 1.000000000000000000, 0.8660254037844387076, 1.000000000000000000, 0.8660254037844387076, 1.000000000000000000, 0.8660254037844387076, 1.000000000000000000, 0.8660254037844387076, 1.000000000000000000, 0.8660254037844387076, 1.000000000000000000, 0.8660254037844387076, 1.000000000000000000, 0.8660254037844387076, 1.000000000000000000, 0.8660254037844387076, 1.000000000000000000, 0.8660254037844387076, 1.000000000000000000, 0.8660254037844387076, 1.000000000000000000, 0.8660254037844387076, 1.000000000000000000, 0.8660254037844387076, 1.000000000000000000, 0.8660254037844387076, 1.000000000000000000, 0.8660254037844387076, 1.000000000000000000, 0.8660254037844387076, 1.000000000000000000, 0.8660254037844387076, 1.000000000000000000, 0.8660254037844387076, 1.000000000000000000, 0.8660254037844387076, 1.000000000000000000, 0.8660254037844387076, 1.000000000000000000, 0.8660254037844387076, 1.000000000000000000, 0.8660254037844387076, 1.000000000000000000, 0.8660254037844387076, 1.000000000000000000, 0.8660254037844387076, 1.000000000000000000, 0.8660254037844387076, 1.000000000000000000, 0.8660254037844387076, 1.000000000000000000, 0.8660254037844387076, 1.000000000000000000, 0.8660254037844387076, 1.000000000000000000, 0.8660254037844387076, 1.000000000000000000, 0.8660254037844387076, 1.000000000000000000, 0.8660254037844387076, 1.000000000000000000, 0.8660254037844387076, 1.000000000000000000, 0.8660254037844387076, 1.000000000000000000, 0.8660254037844387076, 1.000000000000000000, 0.8660254037844387076, 1.000000000000000000, 0.8660254037844387076, 1.000000000000000000, 0.8660254037844387076, 1.000000000000000000, 0.8660254037844387076, 1.000000000000000000, 0.8660254037844387076, 1.000000000000000000, 0.8660254037844387076, 1.000000000000000000, 0.8660254037844387076, 1.000000000000000000, 0.8660254037844387076, 1.000000000000000000, 0.8660254037844387076, 1.000000000000000000, 0.8660254037844387076, 1.000000000000000000, 0.8660254037844387076, 1.000000000000000000, 0.8660254037844387076, 1.000000000000000000, 0.8660254037844387076, 1.000000000000000000, 0.8660254037844387076, 1.000000000000000000, 0.8660254037844387076, 1.000000000000000000, 0.8660254037844387076, 1.000000000000000000, 0.8660254037844387076, 1.000000000000000000, 0.8660254037844387076, 1.000000000000000000, 0.8660254037844387076, 1.000000000000000000, 0.8660254037844387076, 1.000000000000000000, 0.8660254037844387076, 1.000000000000000000, 0.8660254037844387076, 1.000000000000000000, 0.8660254037844387076, 1.000000000000000000, 0.8660254037844387076, 1.000000000000000000, 0.8660254037844387076, 1.000000000000000000, 0.8660254037844387076, 1.000000000000000000, 0.8660254037844387076, 1.000000000000000000, 0.8660254037844387076, 1.000000000000000000, 0.8660254037844387076, 1.000000000000000000, 0.8660254037844387076, 1.000000000000000000, 0.8660254037844387076, 1.000000000000000000, 0.8660254037844387076, 1.000000000000000000, 0.8660254037844387076, 1.000000000000000000, 0.8660254037844387076, 1.000000000000000000, 0.8660254037844387076, 1.000000000000000000, 0.8660254037844387076, 1.000000000000000000, 0.8660254037844387076, 1.000000000000000000, 0.8660254037844387076, 1.000000000000000000, 0.8660254037844387076, 1.000000000000000000, 0.8660254037844387076, 1.000000000000000000, 0.8660254037844387076, 1.000000000000000000, 0.8660254037844387076, 1.000000000000000000, 0.8660254037844387076, 1.000000000000000000, 0.8660254037844387076, 1.000000000000000000, 0.8660254037844387076, 1.000000000000000000, 0.8660254037844387076, 1.000000000000000000),
 ( 1.000000000000000000, 0.8660254037844387076, 1.000000000000000000, 0.8660254037844387076, 1.000000000000000000, 0.8660254037844387076, 1.000000000000000000, 0.8660254037844387076, 1.000000000000000000, 0.8660254037844387076, 1.000000000000000000, 0.8660254037844387076, 1.000000000000000000, 0.8660254037844387076, 1.000000000000000000, 0.8660254037844387076, 1.000000000000000000, 0.8660254037844387076, 1.000000000000000000, 0.8660254037844387076, 1.000000000000000000, 0.8660254037844387076, 1.000000000000000000, 0.8660254037844387076, 1.000000000000000000, 0.8660254037844387076, 1.000000000000000000, 0.8660254037844387076, 1.000000000000000000, 0.8660254037844387076, 1.000000000000000000, 0.8660254037844387076, 1.000000000000000000, 0.8660254037844387076, 1.000000000000000000, 0.8660254037844387076, 1.000000000000000000, 0.8660254037844387076, 1.000000000000000000, 0.8660254037844387076, 1.000000000000000000, 0.8660254037844387076, 1.000000000000000000, 0.8660254037844387076, 1.000000000000000000, 0.8660254037844387076, 1.000000000000000000, 0.8660254037844387076, 1.000000000000000000, 0.8660254037844387076, 1.000000000000000000, 0.8660254037844387076, 1.000000000000000000, 0.8660254037844387076, 1.000000000000000000, 0.8660254037844387076, 1.000000000000000000, 0.8660254037844387076, 1.000000000000000000, 0.8660254037844387076, 1.000000000000000000, 0.8660254037844387076, 1.000000000000000000, 0.8660254037844387076, 1.000000000000000000, 0.8660254037844387076, 1.000000000000000000, 0.8660254037844387076, 1.000000000000000000, 0.8660254037844387076, 1.000000000000000000, 0.8660254037844387076, 1.000000000000000000, 0.8660254037844387076, 1.000000000000000000, 0.8660254037844387076, 1.000000000000000000, 0.8660254037844387076, 1.000000000000000000, 0.8660254037844387076, 1.000000000000000000, 0.8660254037844387076, 1.000000000000000000, 0.8660254037844387076, 1.000000000000000000, 0.8660254037844387076, 1.000000000000000000, 0.8660254037844387076, 1.000000000000000000, 0.8660254037844387076, 1.000000000000000000, 0.8660254037844387076, 1.000000000000000000, 0.8660254037844387076, 1.000000000000000000, 0.8660254037844387076, 1.000000000000000000, 0.8660254037844387076, 1.000000000000000000, 0.8660254037844387076, 1.000000000000000000, 0.8660254037844387076, 1.000000000000000000, 0.8660254037844387076, 1.000000000000000000, 0.8660254037844387076, 1.000000000000000000, 0.8660254037844387076, 1.000000000000000000, 0.8660254037844387076, 1.000000000000000000, 0.8660254037844387076, 1.000000000000000000, 0.8660254037844387076, 1.000000000000000000, 0.8660254037844387076, 1.000000000000000000, 0.8660254037844387076, 1.000000000000000000, 0.8660254037844387076, 1.000000000000000000, 0.8660254037844387076, 1.000000000000000000, 0.8660254037844387076, 1.000000000000000000, 0.8660254037844387076, 1.000000000000000000, 0.8660254037844387076, 1.000000000000000000, 0.8660254037844387076, 1.000000000000000000, 0.8660254037844387076, 1.000000000000000000, 0.8660254037844387076, 1.000000000000000000, 0.8660254037844387076, 1.000000000000000000, 0.8660254037844387076, 1.000000000000000000, 0.8660254037844387076, 1.000000000000000000, 0.8660254037844387076, 1.000000000000000000, 0.8660254037844387076, 1.000000000000000000, 0.8660254037844387076, 1.000000000000000000, 0.8660254037844387076, 1.000000000000000000, 0.8660254037844387076, 1.000000000000000000, 0.8660254037844387076, 1.000000000000000000, 0.8660254037844387076, 1.000000000000000000, 0.8660254037844387076, 1.000000000000000000, 0.8660254037844387076, 1.000000000000000000, 0.8660254037844387076, 1.000000000000000000, 0.8660254037844387076, 1.000000000000000000, 0.8660254037844387076, 1.000000000000000000, 0.8660254037844387076, 1.000000000000000000, 0.8660254037844387076, 1.000000000000000000, 0.8660254037844387076, 1.000000000000000000, 0.8660254037844387076, 1.000000000000000000, 0.8660254037844387076, 1.000000000000000000, 0.8660254037844387076, 1.000000000000000000, 0.8660254037844387076, 1.000000000000000000, 0.8660254037844387076, 1.000000000000000000, 0.8660254037844387076, 1.000000000000000000, 0.8660254037844387076, 1.000000000000000000, 0.8660254037844387076, 1.000000000000000000, 0.8660254037844387076, 1.000000000000000000, 0.8660254037844387076, 1.000000000000000000, 0.8660254037844387076, 1.000000000000000000, 0.8660254037844387076, 1.000000000000000000, 0.8660254037844387076, 1.000000000000000000, 0.8660254037844387076, 1.000000000000000000, 0.8660254037844387076, 1.000000000000000000, 0.8660254037844387076, 1.000000000000000000, 0.8660254037844387076, 1.000000000000000000, 0.8660254037844387076, 1.000000000000000000, 0.8660254037844387076, 1.000000000000000000, 0.8660254037844387076, 1.000000000000000000, 0.8660254037844387076, 1.000000000000000000, 0.8660254037844387076, 1.000000000000000000, 0.8660254037844387076, 1.000000000000000000, 0.8660254037844387076, 1.000000000000000000, 0.8660254037844387076, 1.000000000000000000, 0.8660254037844387076, 1.000000000000000000, 0.8660254037844387076, 1.000000000000000000, 0.8660254037844387076, 1.000000000000000000, 0.8660254037844387076, 1.000000000000000000, 0.8660254037844387076, 1.000000000000000000, 0.8660254037844387076, 1.000000000000000000, 0.8660254037844387076, 1.000000000000000000, 0.8660254037844387076, 1.000000000000000000, 0.8660254037844387076, 1.000000000000000000, 0.8660254037844387076, 1.000000000000000000, 0.8660254037844387076, 1.000000000000000000, 0.8660254037844387076, 1.000000000000000000, 0.8660254037844387076, 1.000000000000000000, 0.8660254037844387076, 1.000000000000000000, 0.8660254037844387076, 1.000000000000000000, 0.8660254037844387076, 1.000000000000000000, 0.8660254037844387076, 1.000000000000000000, 0.8660254037844387076, 1.000000000000000000, 0.8660254037844387076, 1.000000000000000000, 0.8660254037844387076, 1.000000000000000000, 0.8660254037844387076, 1.000000000000000000, 0.8660254037844387076, 1.000000000000000000, 0.8660254037844387076, 1.000000000000000000, 0.8660254037844387076, 1.000000000000000000, 0.8660254037844387076, 1.000000000000000000, 0.8660254037844387076, 1.000000000000000000, 0.8660254037844387076, 1.000000000000000000, 0.8660254037844387076, 1.000000000000000000, 0.8660254037844387076, 1.000000000000000000, 0.8660254037844387076, 1.000000000000000000, 0.8660254037844387076, 1.000000000000000000, 0.8660254037844387076, 1.000000000000000000, 0.8660254037844387076, 1.000000000000000000, 0.8660254037844387076, 1.000000000000000000, 0.8660254037844387076, 1.000000000000000000, 0.8660254037844387076, 1.000000000000000000, 0.8660254037844387076, 1.000000000000000000, 0.8660254037844387076, 1.000000000000000000, 0.8660254037844387076, 1.000000000000000000, 0.8660254037844387076, 1.000000000000000000, 0.8660254037844387076, 1.000000000000000000, 0.8660254037844387076, 1.000000000000000000, 0.8660254037844387076, 1.000000000000000000, 0.8660254037844387076, 1.000000000000000000, 0.8660254037844387076, 1.000000000000000000, 0.8660254037844387076, 1.000000000000000000, 0.8660254037844387076, 1.000000000000000000, 0.8660254037844387076, 1.000000000000000000, 0.8660254037844387076, 1.000000000000000000, 0.8660254037844387076, 1.000000000000000000, 0.8660254037844387076, 1.000000000000000000, 0.8660254037844387076, 1.000000000000000000, 0.8660254037844387076, 1.000000000000000000, 0.8660254037844387076, 1.000000000000000000, 0.8660254037844387076, 1.000000000000000000, 0.8660254037844387076, 1.000000000000000000, 0.8660254037844387076, 1.000000000000000000, 0.8660254037844387076, 1.000000000000000000, 0.8660254037844387076, 1.000000000000000000, 0.8660254037844387076, 1.000000000000000000, 0.8660254037844387076, 1.000000000000000000, 0.8660254037844387076, 1.000000000000000000, 0.8660254037844387076, 1.000000000000000000, 0.8660254037844387076, 1.000000000000000000, 0.8660254037844387076, 1.000000000000000000, 0.8660254037844387076, 1.000000000000000000, 0.8660254037844387076, 1.000000000000000000, 0.8660254037844387076, 1.000000000000000000, 0.8660254037844387076, 1.000000000000000000, 0.8660254037844387076, 1.000000000000000000, 0.8660254037844387076, 1.000000000000000000, 0.8660254037844387076, 1.000000000000000000, 0.8660254037844387076, 1.000000000000000000, 0.8660254037844387076, 1.000000000000000000, 0.8660254037844387076, 1.000000000000000000, 0.8660254037844387076, 1.000000000000000000, 0.8660254037844387076, 1.000000000000000000, 0.8660254037844387076, 1.000000000000000000, 0.8660254037844387076, 1.000000000000000000, 0.8660254037844387076, 1.000000000000000000, 0.8660254037844387076, 1.000000000000000000, 0.8660254037844387076, 1.000000000000000000) ) ) 
 REPRESENTATION_ITEM ( '' )  SURFACE ( )  );
#10830=CARTESIAN_POINT ( 'NONE',  ( -62.49999999999998579, 15.88541666598386826, 2.366025403784441483 ) ) ;
#10831=CARTESIAN_POINT ( 'NONE',  ( -61.13531646874998415, 11.39062499965860020, 1.500000000000002220 ) ) ;
#10833=VERTEX_POINT ( 'NONE', #4322 ) ;
#10837=CARTESIAN_POINT ( 'NONE',  ( -62.86468353124998742, 13.97395833299193413, 1.999225269531025972 ) ) ;
#10838=CARTESIAN_POINT ( 'NONE',  ( -61.99999999999998579, 16.00000000000000000, 1.500000000000002220 ) ) ;
#10839=CARTESIAN_POINT ( 'NONE',  ( -61.49999999999998579, 14.45833333333333393, 2.366025403784441927 ) ) ;
#10840=CYLINDRICAL_SURFACE ( 'NONE', #1015, 0.9999999999999981126 ) ;
#10841=CARTESIAN_POINT ( 'NONE',  ( -61.56765823437498142, 12.68229166632526805, 0.7511620957034663704 ) ) ;
#10842=CARTESIAN_POINT ( 'NONE',  ( -61.13531646874998415, 15.41145833299193413, 1.000774730468978468 ) ) ;
#10847=CARTESIAN_POINT ( 'NONE',  ( -62.86468353124998742, 8.286458332991934128, 1.999225269531025972 ) ) ;
#10853=CARTESIAN_POINT ( 'NONE',  ( -62.43234176562499016, 14.24479166632526983, 2.248837904296538071 ) ) ;
#10854=CARTESIAN_POINT ( 'NONE',  ( -61.13531646874998415, 9.557291666325269830, 1.999225269531026417 ) ) ;
#10855=CARTESIAN_POINT ( 'NONE',  ( -61.56765823437498852, 15.34895833299193590, 2.248837904296538515 ) ) ;
#10856=DIRECTION ( 'NONE',  ( -0.000000000000000000, -1.000000000000000000, -0.000000000000000000 ) ) ;
#10857=VERTEX_POINT ( 'NONE', #7008 ) ;
#10858=CARTESIAN_POINT ( 'NONE',  ( -61.99999999999998579, 14.06250000000000178, 0.3452994616207497591 ) ) ;
#10859=CARTESIAN_POINT ( 'NONE',  ( -62.86468353124998032, 9.244791666325268054, 1.000774730468978024 ) ) ;
#10860=CARTESIAN_POINT ( 'NONE',  ( -61.99999999999998579, 12.53124999931720396, 0.3452994616207497591 ) ) ;
#10862=EDGE_CURVE ( 'NONE', #6385, #10637, #5384, .T. ) ;
#10864=CARTESIAN_POINT ( 'NONE',  ( -62.43234176562498305, 13.91145833299193413, 0.7511620957034662593 ) ) ;
#10865=CARTESIAN_POINT ( 'NONE',  ( -61.73205080756886076, 11.44866454968463110, 2.500000000000000000 ) ) ;
#10868=AXIS2_PLACEMENT_3D ( 'NONE', #522, #7349, #5675 ) ;
#10869=CARTESIAN_POINT ( 'NONE',  ( -62.43234176562498305, 12.22395833299193413, 0.7511620957034662593 ) ) ;
#10871=CYLINDRICAL_SURFACE ( 'NONE', #1036, 0.9999999999999981126 ) ;
#10876=VERTEX_POINT ( 'NONE', #7901 ) ;
#10879=CARTESIAN_POINT ( 'NONE',  ( -60.99999999999998579, 10.97916666666666607, 2.077350269189628840 ) ) ;
#10880=CYLINDRICAL_SURFACE ( 'NONE', #1032, 0.9999999999999981126 ) ;
#10883=CARTESIAN_POINT ( 'NONE',  ( -62.99999999999998579, 8.843749999317203958, 1.500000000000001998 ) ) ;
#10884=CARTESIAN_POINT ( 'NONE',  ( -62.43234176562498305, 13.72395833299193413, 0.7511620957034662593 ) ) ;
#10885=CARTESIAN_POINT ( 'NONE',  ( -61.99999999999997868, 10.68749999999999822, 2.500000000000002665 ) ) ;
#10888=EDGE_LOOP ( 'NONE', ( #7651, #7767, #7663, #5623 ) ) ;
#10890=CARTESIAN_POINT ( 'NONE',  ( -61.56765823437498142, 14.86979166632526805, 0.7511620957034663704 ) ) ;
#10891=FACE_OUTER_BOUND ( 'NONE', #3535, .T. ) ;
#10892=CARTESIAN_POINT ( 'NONE',  ( -61.99999999999998579, 9.906249999317202182, 2.500000000000002665 ) ) ;
#10893=( BOUNDED_CURVE ( )  B_SPLINE_CURVE ( 2, ( #6786, #4264, #7672, #55, #10208, #6166, #10438, #2119, #455 ),
 .UNSPECIFIED., .F., .F. ) 
 B_SPLINE_CURVE_WITH_KNOTS ( ( 3, 2, 2, 2, 3 ),
 ( 0.1015625000000000833, 0.1041666666666666713, 0.1093750000000000000, 0.1145833333333333287, 0.1171875000000000278 ),
 .UNSPECIFIED. ) 
 CURVE ( )  GEOMETRIC_REPRESENTATION_ITEM ( )  RATIONAL_B_SPLINE_CURVE ( ( 0.9330127018922194093, 0.9330127018922215187, 1.000000000000000000, 0.8660254037844387076, 1.000000000000000000, 0.8660254037844387076, 1.000000000000000000, 0.9330127018922186322, 0.9330127018922194093 ) ) 
 REPRESENTATION_ITEM ( '' )  );
#10895=CARTESIAN_POINT ( 'NONE',  ( -61.13531646874997705, 12.16145833299193413, 1.000774730468978468 ) ) ;
#10896=CARTESIAN_POINT ( 'NONE',  ( -61.13531646874998415, 16.14062499965860198, 1.500000000000002220 ) ) ;
#10899=CARTESIAN_POINT ( 'NONE',  ( -61.13531646874998415, 8.161458332991935904, 1.000774730468978468 ) ) ;
#10901=ORIENTED_EDGE ( 'NONE', *, *, #3545, .T. ) ;
#10902=DIRECTION ( 'NONE',  ( -0.000000000000000000, -1.000000000000000000, -0.000000000000000000 ) ) ;
#10903=CARTESIAN_POINT ( 'NONE',  ( -62.26794919243111082, 12.57366454968463110, 0.5000000000000013323 ) ) ;
#10904=EDGE_CURVE ( 'NONE', #1104, #4762, #7716, .T. ) ;
#10905=CARTESIAN_POINT ( 'NONE',  ( -62.86468353124998032, 14.68229166632526805, 1.000774730468978024 ) ) ;
#10906=CARTESIAN_POINT ( 'NONE',  ( -61.99999999999998579, 10.01562499965860020, 2.498450539062049724 ) ) ;
#10907=CARTESIAN_POINT ( 'NONE',  ( -61.13531646874997705, 15.41145833299193590, 1.000774730468978468 ) ) ;
#10908=DIRECTION ( 'NONE',  ( 0.000000000000000000, 0.000000000000000000, -1.000000000000000000 ) ) ;
#10910=CARTESIAN_POINT ( 'NONE',  ( -62.99999999999998579, 13.14583333333333215, 2.077350269189627952 ) ) ;
#10911=CARTESIAN_POINT ( 'NONE',  ( -61.13531646874997705, 8.411458332991934128, 1.000774730468978468 ) ) ;
#10912=CARTESIAN_POINT ( 'NONE',  ( -62.49999999999998579, 11.30208333265053611, 0.6339745962155627357 ) ) ;
#10913=CYLINDRICAL_SURFACE ( 'NONE', #1292, 0.9999999999999981126 ) ;
#10914=CARTESIAN_POINT ( 'NONE',  ( -61.99999999999998579, 14.39062499965859843, 0.5015494609379544944 ) ) ;
#10915=CARTESIAN_POINT ( 'NONE',  ( -61.99999999999998579, 11.56250000000000000, 0.5000000000000013323 ) ) ;
#10916=ORIENTED_EDGE ( 'NONE', *, *, #479, .T. ) ;
#10918=CARTESIAN_POINT ( 'NONE',  ( -61.56765823437498852, 13.34895833299193413, 2.248837904296538515 ) ) ;
#10919=DIRECTION ( 'NONE',  ( -0.000000000000000000, -1.000000000000000000, -0.000000000000000000 ) ) ;
#10926=CARTESIAN_POINT ( 'NONE',  ( -60.99999999999998579, 10.77083333333333215, 0.9226497308103762673 ) ) ;
#10927=ORIENTED_EDGE ( 'NONE', *, *, #4449, .F. ) ;
#10928=CARTESIAN_POINT ( 'NONE',  ( -62.86468353124998742, 8.286458332991934128, 1.999225269531025972 ) ) ;
#10930=CARTESIAN_POINT ( 'NONE',  ( -61.13531646874998415, 12.91145833299193590, 1.000774730468978468 ) ) ;
#10935=CARTESIAN_POINT ( 'NONE',  ( -61.49999999999998579, 12.70833333333333393, 2.366025403784441927 ) ) ;
#10936=CARTESIAN_POINT ( 'NONE',  ( -61.13531646874998415, 15.09895833299193413, 1.000774730468978468 ) ) ;
#10937=LINE ( 'NONE', #5095, #8940 ) ;
#10939=CARTESIAN_POINT ( 'NONE',  ( -61.49999999999998579, 10.79166666666666607, 0.6339745962155628467 ) ) ;
#10940=CARTESIAN_POINT ( 'NONE',  ( -61.13531646874998415, 12.64062499965860198, 1.500000000000002220 ) ) ;
#10941=CARTESIAN_POINT ( 'NONE',  ( -61.56765823437498142, 14.93229166632526805, 0.7511620957034663704 ) ) ;
#10942=DIRECTION ( 'NONE',  ( 0.000000000000000000, 0.000000000000000000, -1.000000000000000000 ) ) ;
#10943=CARTESIAN_POINT ( 'NONE',  ( -61.99999999999998579, 13.53124999931720041, 0.5000000000000013323 ) ) ;
#10944=CARTESIAN_POINT ( 'NONE',  ( -61.13531646874998415, 9.161458332991935904, 1.000774730468978468 ) ) ;
#10946=DIRECTION ( 'NONE',  ( -0.000000000000000000, -1.000000000000000000, -0.000000000000000000 ) ) ;
#10947=ORIENTED_EDGE ( 'NONE', *, *, #8053, .T. ) ;
#10951=( BOUNDED_CURVE ( )  B_SPLINE_CURVE ( 2, ( #7296, #463, #1237, #8130, #9680, #9734, #4673, #6468, #519 ),
 .UNSPECIFIED., .F., .T. ) 
 B_SPLINE_CURVE_WITH_KNOTS ( ( 3, 2, 2, 2, 3 ),
 ( 0.1328125000000000000, 0.1354166666666666574, 0.1406250000000000000, 0.1458333333333333426, 0.1484374999999999722 ),
 .UNSPECIFIED. ) 
 CURVE ( )  GEOMETRIC_REPRESENTATION_ITEM ( )  RATIONAL_B_SPLINE_CURVE ( ( 0.9330127018922194093, 0.9330127018922194093, 1.000000000000000000, 0.8660254037844387076, 1.000000000000000000, 0.8660254037844387076, 1.000000000000000000, 0.9330127018922200755, 0.9330127018922194093 ) ) 
 REPRESENTATION_ITEM ( '' )  );
#10952=CARTESIAN_POINT ( 'NONE',  ( -61.56765823437498142, 13.61979166632526805, 0.7511620957034663704 ) ) ;
#10953=CARTESIAN_POINT ( 'NONE',  ( -62.86468353124998742, 11.72395833299193413, 1.999225269531025972 ) ) ;
#10954=VECTOR ( 'NONE', #5836, 1000.000000000000000 ) ;
#10955=CARTESIAN_POINT ( 'NONE',  ( -62.86468353124999453, 15.26562499965860020, 1.500000000000002220 ) ) ;
#10956=CARTESIAN_POINT ( 'NONE',  ( -61.49999999999998579, 14.51041666598387003, 0.6339745962155628467 ) ) ;
#10958=CARTESIAN_POINT ( 'NONE',  ( -61.99999999999998579, 14.93749999999999822, 2.654700538379254571 ) ) ;
#10960=CARTESIAN_POINT ( 'NONE',  ( -62.86468353124999453, 8.536458332991934128, 1.999225269531025750 ) ) ;
#10961=CARTESIAN_POINT ( 'NONE',  ( -61.49999999999998579, 13.51041666598387003, 0.6339745962155628467 ) ) ;
#10963=AXIS2_PLACEMENT_3D ( 'NONE', #5768, #9062, #1394 ) ;
#10965=CARTESIAN_POINT ( 'NONE',  ( -61.99999999999998579, 14.01562499965860376, 2.498450539062049724 ) ) ;
#10968=EDGE_CURVE ( 'NONE', #10494, #7302, #8903, .T. ) ;
#10971=CARTESIAN_POINT ( 'NONE',  ( -61.13531646874998415, 12.66145833299193413, 1.000774730468978468 ) ) ;
#10972=DIRECTION ( 'NONE',  ( 0.000000000000000000, 0.000000000000000000, -1.000000000000000000 ) ) ;
#10973=EDGE_CURVE ( 'NONE', #8746, #7043, #10338, .T. ) ;
#10978=CARTESIAN_POINT ( 'NONE',  ( -61.99999999999998579, 8.437500000000000000, 2.500000000000002665 ) ) ;
#10979=VERTEX_POINT ( 'NONE', #337 ) ;
#10980=CARTESIAN_POINT ( 'NONE',  ( -60.99999999999998579, 10.50000000000000000, 1.500000000000002220 ) ) ;
#10981=CARTESIAN_POINT ( 'NONE',  ( -61.73205080756886076, 13.80133545031537068, 0.5000000000000014433 ) ) ;
#11021=COLOUR_RGB('Black',0.12,0.14,0.17);
#11022=FILL_AREA_STYLE_COLOUR('',#11021);
#11023=FILL_AREA_STYLE('',(#11022));
#11024=SURFACE_STYLE_FILL_AREA(#11023);
#11025=SURFACE_SIDE_STYLE('',(#11024));
#11026=SURFACE_STYLE_USAGE(.BOTH.,#11025);
#11027=PRESENTATION_STYLE_ASSIGNMENT((#11026));
ENDSEC;
END-ISO-10303-21;
